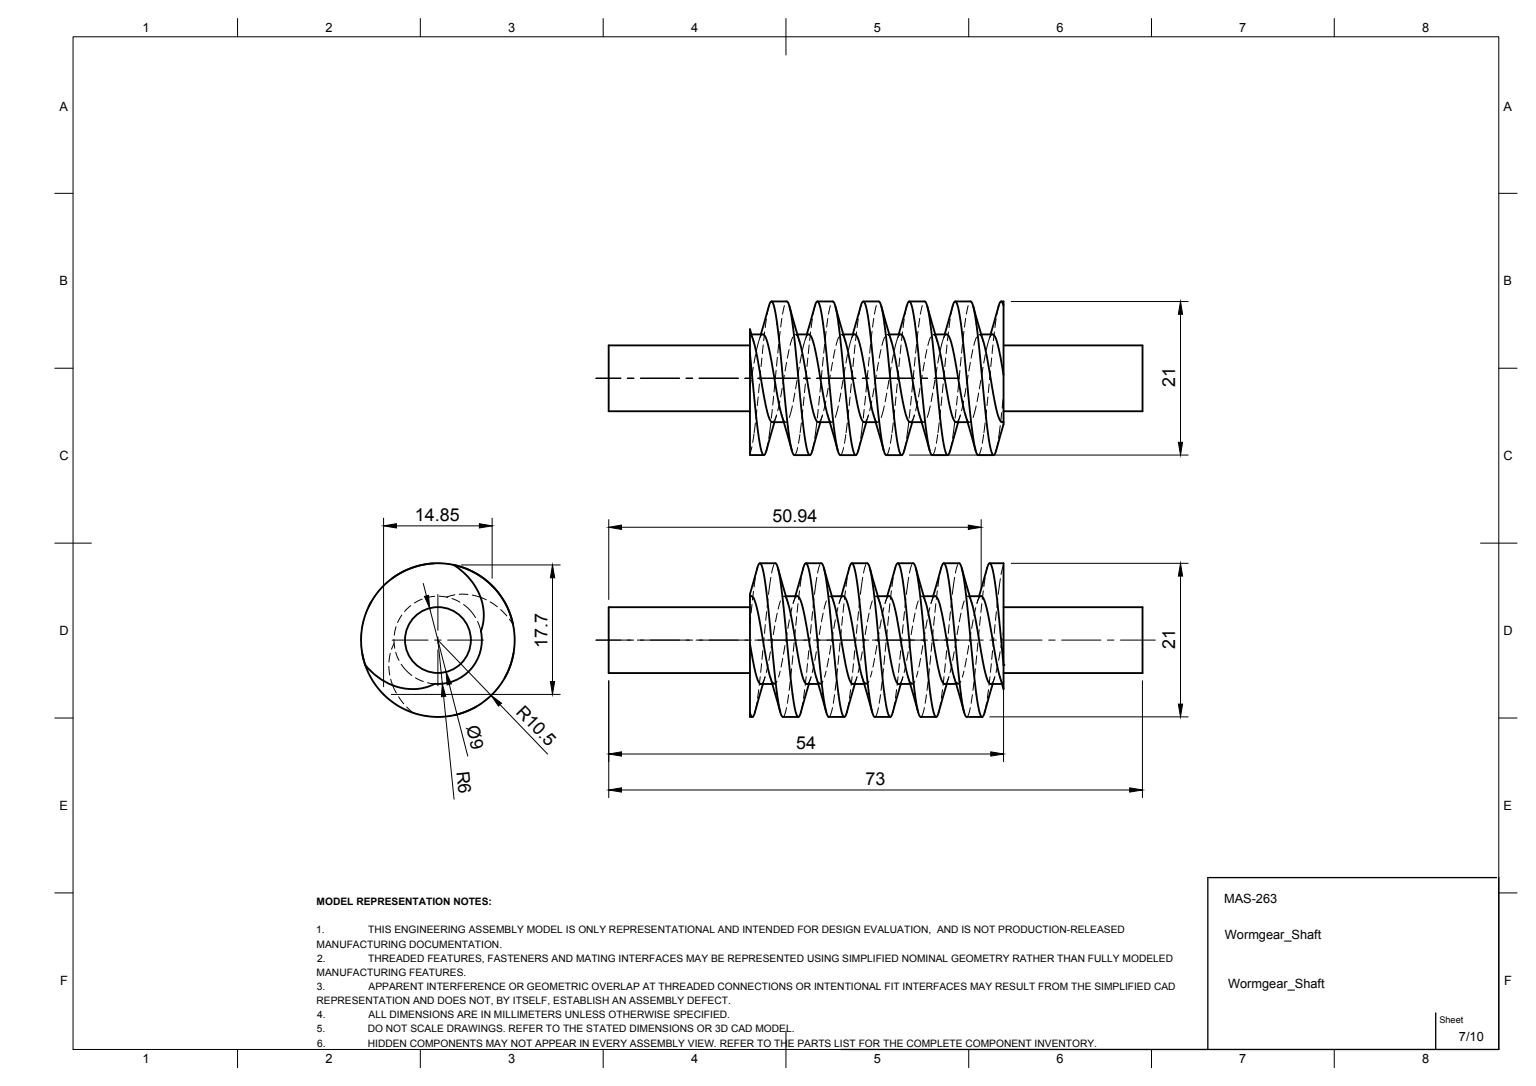
ISO-10303-21;
HEADER;
/* Generated by software containing ST-Developer
 * from STEP Tools, Inc. (www.steptools.com) 
 */

FILE_DESCRIPTION(
/* description */ (''),
/* implementation_level */ '2;1');

FILE_NAME(
/* name */ 'Wormgear_Shaft.step',
/* time_stamp */ '2026-10-12T15:47:30-07:00',
/* author */ (''),
/* organization */ (''),
/* preprocessor_version */ 'ST-DEVELOPER v20.2',
/* originating_system */ 'Autodesk Translation Framework v15.15.0.0',
/* authorisation */ '');

FILE_SCHEMA (('AUTOMOTIVE_DESIGN { 1 0 10303 214 3 1 1 }'));
ENDSEC;

DATA;
#10=MECHANICAL_DESIGN_GEOMETRIC_PRESENTATION_REPRESENTATION('',(#85),#88483);
#67=SHAPE_REPRESENTATION_RELATIONSHIP('SRR','None',#88523,#76);
#76=ADVANCED_BREP_SHAPE_REPRESENTATION('',(#120),#88477);
#85=STYLED_ITEM('',(#88574),#120);
#120=MANIFOLD_SOLID_BREP('Body1',#12995);
#238=ELLIPSE('',#13840,8.40043383461932,7.09899410493904);
#239=ELLIPSE('',#13843,8.34870203930529,7.04180185640227);
#366=FACE_BOUND('',#1889,.T.);
#367=FACE_BOUND('',#1894,.T.);
#519=PLANE('',#13839);
#520=PLANE('',#13842);
#521=PLANE('',#13849);
#522=PLANE('',#13850);
#758=B_SPLINE_SURFACE_WITH_KNOTS('',3,3,((#85029,#85030,#85031,#85032),
(#85033,#85034,#85035,#85036),(#85037,#85038,#85039,#85040),(#85041,#85042,
#85043,#85044)),.UNSPECIFIED.,.F.,.F.,.F.,(4,4),(4,4),(0.0217391304347818,
0.617536119336012),(0.774386899537597,1.),.UNSPECIFIED.);
#759=B_SPLINE_SURFACE_WITH_KNOTS('',3,3,((#85046,#85047,#85048,#85049,#85050,
#85051,#85052,#85053,#85054,#85055),(#85056,#85057,#85058,#85059,#85060,
#85061,#85062,#85063,#85064,#85065),(#85066,#85067,#85068,#85069,#85070,
#85071,#85072,#85073,#85074,#85075),(#85076,#85077,#85078,#85079,#85080,
#85081,#85082,#85083,#85084,#85085)),.UNSPECIFIED.,.F.,.F.,.F.,(4,4),(4,
1,1,1,1,1,1,4),(0.0216104565420008,1.00130145442866),(-0.000128673892780755,
0.142857142857143,0.285714285714286,0.428571428571429,0.571428571428571,
0.714285714285714,0.857142857142857,1.00130145442866),.UNSPECIFIED.);
#760=B_SPLINE_SURFACE_WITH_KNOTS('',3,3,((#85096,#85097,#85098,#85099,#85100,
#85101,#85102,#85103),(#85104,#85105,#85106,#85107,#85108,#85109,#85110,
#85111),(#85112,#85113,#85114,#85115,#85116,#85117,#85118,#85119),(#85120,
#85121,#85122,#85123,#85124,#85125,#85126,#85127)),.UNSPECIFIED.,.F.,.F.,
 .F.,(4,4),(4,1,1,1,1,4),(0.,1.00001448148635),(0.144829272278474,0.266996519095835,
0.389163765913196,0.633498259547918,0.877832753182639,1.00001448148635),
 .UNSPECIFIED.);
#761=B_SPLINE_SURFACE_WITH_KNOTS('',3,3,((#85395,#85396,#85397,#85398,#85399,
#85400,#85401,#85402,#85403),(#85404,#85405,#85406,#85407,#85408,#85409,
#85410,#85411,#85412),(#85413,#85414,#85415,#85416,#85417,#85418,#85419,
#85420,#85421),(#85422,#85423,#85424,#85425,#85426,#85427,#85428,#85429,
#85430)),.UNSPECIFIED.,.F.,.F.,.F.,(4,4),(4,1,1,1,1,1,4),(-1.22172294938054E-5,
1.),(-1.22172294938054E-5,0.12216720883009,0.24433441766018,0.488668835320359,
0.610836044150449,0.733003252980539,0.855170461810629),.UNSPECIFIED.);
#762=B_SPLINE_SURFACE_WITH_KNOTS('',3,3,((#85465,#85466,#85467,#85468),
(#85469,#85470,#85471,#85472),(#85473,#85474,#85475,#85476),(#85477,#85478,
#85479,#85480)),.UNSPECIFIED.,.F.,.F.,.F.,(4,4),(4,4),(0.512899287463832,
1.),(0.,0.18445259717643),.UNSPECIFIED.);
#763=B_SPLINE_SURFACE_WITH_KNOTS('',3,3,((#85482,#85483,#85484,#85485,#85486,
#85487,#85488,#85489,#85490,#85491),(#85492,#85493,#85494,#85495,#85496,
#85497,#85498,#85499,#85500,#85501),(#85502,#85503,#85504,#85505,#85506,
#85507,#85508,#85509,#85510,#85511),(#85512,#85513,#85514,#85515,#85516,
#85517,#85518,#85519,#85520,#85521)),.UNSPECIFIED.,.F.,.F.,.F.,(4,4),(4,
1,1,1,1,1,1,4),(0.0216104646765061,1.),(-0.000128665758275638,0.142857142857143,
0.285714285714286,0.428571428571429,0.571428571428571,0.714285714285714,
0.857142857142857,1.),.UNSPECIFIED.);
#764=B_SPLINE_SURFACE_WITH_KNOTS('',3,3,((#85543,#85544,#85545,#85546),
(#85547,#85548,#85549,#85550),(#85551,#85552,#85553,#85554),(#85555,#85556,
#85557,#85558)),.UNSPECIFIED.,.F.,.F.,.F.,(4,4),(4,4),(0.382464506767468,
0.978260874456547),(0.,0.225612834551505),.UNSPECIFIED.);
#765=B_SPLINE_SURFACE_WITH_KNOTS('',3,3,((#85560,#85561,#85562,#85563,#85564,
#85565,#85566,#85567,#85568,#85569),(#85570,#85571,#85572,#85573,#85574,
#85575,#85576,#85577,#85578,#85579),(#85580,#85581,#85582,#85583,#85584,
#85585,#85586,#85587,#85588,#85589),(#85590,#85591,#85592,#85593,#85594,
#85595,#85596,#85597,#85598,#85599)),.UNSPECIFIED.,.F.,.F.,.F.,(4,4),(4,
1,1,1,1,1,1,4),(0.,0.97838954356546),(-0.00012866910891396,0.142857142857143,
0.285714285714286,0.428571428571429,0.571428571428571,0.714285714285714,
0.857142857142857,1.00010925279131),.UNSPECIFIED.);
#766=B_SPLINE_SURFACE_WITH_KNOTS('',3,3,((#85613,#85614,#85615,#85616,#85617,
#85618,#85619,#85620,#85621,#85622),(#85623,#85624,#85625,#85626,#85627,
#85628,#85629,#85630,#85631,#85632),(#85633,#85634,#85635,#85636,#85637,
#85638,#85639,#85640,#85641,#85642),(#85643,#85644,#85645,#85646,#85647,
#85648,#85649,#85650,#85651,#85652)),.UNSPECIFIED.,.F.,.F.,.F.,(4,4),(4,
1,1,1,1,1,1,4),(0.,1.),(0.,0.142857142857143,0.285714285714286,0.428571428571429,
0.571428571428571,0.714285714285714,0.857142857142857,1.),.UNSPECIFIED.);
#767=B_SPLINE_SURFACE_WITH_KNOTS('',3,3,((#85654,#85655,#85656,#85657,#85658,
#85659,#85660,#85661,#85662,#85663),(#85664,#85665,#85666,#85667,#85668,
#85669,#85670,#85671,#85672,#85673),(#85674,#85675,#85676,#85677,#85678,
#85679,#85680,#85681,#85682,#85683),(#85684,#85685,#85686,#85687,#85688,
#85689,#85690,#85691,#85692,#85693)),.UNSPECIFIED.,.F.,.F.,.F.,(4,4),(4,
1,1,1,1,1,1,4),(0.0216103522188689,1.),(-0.00012877821591213,0.142857142857143,
0.285714285714286,0.428571428571429,0.571428571428571,0.714285714285714,
0.857142857142857,1.00010930858083),.UNSPECIFIED.);
#768=B_SPLINE_SURFACE_WITH_KNOTS('',3,3,((#85708,#85709,#85710,#85711,#85712,
#85713,#85714,#85715,#85716,#85717),(#85718,#85719,#85720,#85721,#85722,
#85723,#85724,#85725,#85726,#85727),(#85728,#85729,#85730,#85731,#85732,
#85733,#85734,#85735,#85736,#85737),(#85738,#85739,#85740,#85741,#85742,
#85743,#85744,#85745,#85746,#85747)),.UNSPECIFIED.,.F.,.F.,.F.,(4,4),(4,
1,1,1,1,1,1,4),(0.,0.97838966897386),(-0.00012879451731267,0.142857142857143,
0.285714285714286,0.428571428571429,0.571428571428571,0.714285714285714,
0.857142857142857,1.00010890844888),.UNSPECIFIED.);
#769=B_SPLINE_SURFACE_WITH_KNOTS('',3,3,((#85762,#85763,#85764,#85765,#85766,
#85767,#85768,#85769,#85770,#85771),(#85772,#85773,#85774,#85775,#85776,
#85777,#85778,#85779,#85780,#85781),(#85782,#85783,#85784,#85785,#85786,
#85787,#85788,#85789,#85790,#85791),(#85792,#85793,#85794,#85795,#85796,
#85797,#85798,#85799,#85800,#85801)),.UNSPECIFIED.,.F.,.F.,.F.,(4,4),(4,
1,1,1,1,1,1,4),(0.,1.),(0.,0.142857142857143,0.285714285714286,0.428571428571429,
0.571428571428571,0.714285714285714,0.857142857142857,1.),.UNSPECIFIED.);
#770=B_SPLINE_SURFACE_WITH_KNOTS('',3,3,((#85804,#85805,#85806,#85807,#85808,
#85809,#85810,#85811,#85812,#85813),(#85814,#85815,#85816,#85817,#85818,
#85819,#85820,#85821,#85822,#85823),(#85824,#85825,#85826,#85827,#85828,
#85829,#85830,#85831,#85832,#85833),(#85834,#85835,#85836,#85837,#85838,
#85839,#85840,#85841,#85842,#85843)),.UNSPECIFIED.,.F.,.F.,.F.,(4,4),(4,
1,1,1,1,1,1,4),(0.0216102027499123,1.),(-0.000128927684868709,0.142857142857143,
0.285714285714286,0.428571428571429,0.571428571428571,0.714285714285714,
0.857142857142857,1.00010894090728),.UNSPECIFIED.);
#771=B_SPLINE_SURFACE_WITH_KNOTS('',3,3,((#85858,#85859,#85860,#85861,#85862,
#85863,#85864,#85865,#85866,#85867),(#85868,#85869,#85870,#85871,#85872,
#85873,#85874,#85875,#85876,#85877),(#85878,#85879,#85880,#85881,#85882,
#85883,#85884,#85885,#85886,#85887),(#85888,#85889,#85890,#85891,#85892,
#85893,#85894,#85895,#85896,#85897)),.UNSPECIFIED.,.F.,.F.,.F.,(4,4),(4,
1,1,1,1,1,1,4),(-3.49469805785124E-7,0.978389836394998),(-0.000128961938451469,
0.142857142857143,0.285714285714286,0.428571428571429,0.571428571428571,
0.714285714285714,0.857142857142857,1.00010852689685),.UNSPECIFIED.);
#772=B_SPLINE_SURFACE_WITH_KNOTS('',3,3,((#85920,#85921,#85922,#85923,#85924,
#85925,#85926,#85927,#85928,#85929),(#85930,#85931,#85932,#85933,#85934,
#85935,#85936,#85937,#85938,#85939),(#85940,#85941,#85942,#85943,#85944,
#85945,#85946,#85947,#85948,#85949),(#85950,#85951,#85952,#85953,#85954,
#85955,#85956,#85957,#85958,#85959)),.UNSPECIFIED.,.F.,.F.,.F.,(4,4),(4,
1,1,1,1,1,1,4),(0.,1.00000113587033),(0.,0.142857142857143,0.285714285714286,
0.428571428571429,0.571428571428571,0.714285714285714,0.857142857142857,
1.),.UNSPECIFIED.);
#773=B_SPLINE_SURFACE_WITH_KNOTS('',3,3,((#85962,#85963,#85964,#85965,#85966,
#85967,#85968,#85969,#85970,#85971),(#85972,#85973,#85974,#85975,#85976,
#85977,#85978,#85979,#85980,#85981),(#85982,#85983,#85984,#85985,#85986,
#85987,#85988,#85989,#85990,#85991),(#85992,#85993,#85994,#85995,#85996,
#85997,#85998,#85999,#86000,#86001)),.UNSPECIFIED.,.F.,.F.,.F.,(4,4),(4,
1,1,1,1,1,1,4),(0.0216101883594699,1.),(-0.000128942075311584,0.142857142857143,
0.285714285714286,0.428571428571429,0.571428571428571,0.714285714285714,
0.857142857142857,1.00010890887743),.UNSPECIFIED.);
#774=B_SPLINE_SURFACE_WITH_KNOTS('',3,3,((#86028,#86029,#86030,#86031,#86032,
#86033,#86034,#86035,#86036,#86037),(#86038,#86039,#86040,#86041,#86042,
#86043,#86044,#86045,#86046,#86047),(#86048,#86049,#86050,#86051,#86052,
#86053,#86054,#86055,#86056,#86057),(#86058,#86059,#86060,#86061,#86062,
#86063,#86064,#86065,#86066,#86067)),.UNSPECIFIED.,.F.,.F.,.F.,(4,4),(4,
1,1,1,1,1,1,4),(0.,0.978389731943835),(-0.00012885748728817,0.142857142857143,
0.285714285714286,0.428571428571429,0.571428571428571,0.714285714285714,
0.857142857142857,1.00010875621283),.UNSPECIFIED.);
#775=B_SPLINE_SURFACE_WITH_KNOTS('',3,3,((#86082,#86083,#86084,#86085,#86086,
#86087,#86088,#86089,#86090,#86091),(#86092,#86093,#86094,#86095,#86096,
#86097,#86098,#86099,#86100,#86101),(#86102,#86103,#86104,#86105,#86106,
#86107,#86108,#86109,#86110,#86111),(#86112,#86113,#86114,#86115,#86116,
#86117,#86118,#86119,#86120,#86121)),.UNSPECIFIED.,.F.,.F.,.F.,(4,4),(4,
1,1,1,1,1,1,4),(0.,1.),(0.,0.142857142857143,0.285714285714286,0.428571428571429,
0.571428571428571,0.714285714285714,0.857142857142857,1.),.UNSPECIFIED.);
#776=B_SPLINE_SURFACE_WITH_KNOTS('',3,3,((#86124,#86125,#86126,#86127,#86128,
#86129,#86130,#86131,#86132,#86133),(#86134,#86135,#86136,#86137,#86138,
#86139,#86140,#86141,#86142,#86143),(#86144,#86145,#86146,#86147,#86148,
#86149,#86150,#86151,#86152,#86153),(#86154,#86155,#86156,#86157,#86158,
#86159,#86160,#86161,#86162,#86163)),.UNSPECIFIED.,.F.,.F.,.F.,(4,4),(4,
1,1,1,1,1,1,4),(0.0216103414761888,1.),(-0.000128788958592299,0.142857142857143,
0.285714285714286,0.428571428571429,0.571428571428571,0.714285714285714,
0.857142857142857,1.00010927970758),.UNSPECIFIED.);
#777=B_SPLINE_SURFACE_WITH_KNOTS('',3,3,((#86190,#86191,#86192,#86193,#86194,
#86195,#86196,#86197,#86198,#86199),(#86200,#86201,#86202,#86203,#86204,
#86205,#86206,#86207,#86208,#86209),(#86210,#86211,#86212,#86213,#86214,
#86215,#86216,#86217,#86218,#86219),(#86220,#86221,#86222,#86223,#86224,
#86225,#86226,#86227,#86228,#86229)),.UNSPECIFIED.,.F.,.F.,.F.,(4,4),(4,
1,1,1,1,1,1,4),(0.,0.978389590969423),(-0.000128716512876252,0.142857142857143,
0.285714285714286,0.428571428571429,0.571428571428571,0.714285714285714,
0.857142857142857,1.00010911520136),.UNSPECIFIED.);
#778=B_SPLINE_SURFACE_WITH_KNOTS('',3,3,((#86244,#86245,#86246,#86247,#86248,
#86249,#86250,#86251,#86252,#86253),(#86254,#86255,#86256,#86257,#86258,
#86259,#86260,#86261,#86262,#86263),(#86264,#86265,#86266,#86267,#86268,
#86269,#86270,#86271,#86272,#86273),(#86274,#86275,#86276,#86277,#86278,
#86279,#86280,#86281,#86282,#86283)),.UNSPECIFIED.,.F.,.F.,.F.,(4,4),(4,
1,1,1,1,1,1,4),(0.,1.),(0.,0.142857142857143,0.285714285714286,0.428571428571429,
0.571428571428571,0.714285714285714,0.857142857142857,1.),.UNSPECIFIED.);
#779=B_SPLINE_SURFACE_WITH_KNOTS('',3,3,((#86286,#86287,#86288,#86289),
(#86290,#86291,#86292,#86293),(#86294,#86295,#86296,#86297),(#86298,#86299,
#86300,#86301)),.UNSPECIFIED.,.F.,.F.,.F.,(4,4),(4,4),(0.,0.487101414751205),
(0.815547136912673,1.),.UNSPECIFIED.);
#780=B_SPLINE_SURFACE_WITH_KNOTS('',3,3,((#86303,#86304,#86305,#86306,#86307,
#86308,#86309,#86310,#86311,#86312),(#86313,#86314,#86315,#86316,#86317,
#86318,#86319,#86320,#86321,#86322),(#86323,#86324,#86325,#86326,#86327,
#86328,#86329,#86330,#86331,#86332),(#86333,#86334,#86335,#86336,#86337,
#86338,#86339,#86340,#86341,#86342)),.UNSPECIFIED.,.F.,.F.,.F.,(4,4),(4,
1,1,1,1,1,1,4),(-0.00139422224055136,0.978389538674135),(-0.00139422224055136,
0.142857142857143,0.285714285714286,0.428571428571429,0.571428571428571,
0.714285714285714,0.857142857142857,1.00012866910892),.UNSPECIFIED.);
#781=B_SPLINE_SURFACE_WITH_KNOTS('',3,3,((#86343,#86344,#86345,#86346,#86347,
#86348,#86349,#86350,#86351,#86352),(#86353,#86354,#86355,#86356,#86357,
#86358,#86359,#86360,#86361,#86362),(#86363,#86364,#86365,#86366,#86367,
#86368,#86369,#86370,#86371,#86372),(#86373,#86374,#86375,#86376,#86377,
#86378,#86379,#86380,#86381,#86382)),.UNSPECIFIED.,.F.,.F.,.F.,(4,4),(4,
1,1,1,1,1,1,4),(0.0216103522188697,1.),(-0.000128778215911952,0.142857142857143,
0.285714285714286,0.428571428571429,0.571428571428571,0.714285714285714,
0.857142857142857,1.00012877821591),.UNSPECIFIED.);
#782=B_SPLINE_SURFACE_WITH_KNOTS('',3,3,((#86393,#86394,#86395,#86396,#86397,
#86398,#86399,#86400,#86401,#86402),(#86403,#86404,#86405,#86406,#86407,
#86408,#86409,#86410,#86411,#86412),(#86413,#86414,#86415,#86416,#86417,
#86418,#86419,#86420,#86421,#86422),(#86423,#86424,#86425,#86426,#86427,
#86428,#86429,#86430,#86431,#86432)),.UNSPECIFIED.,.F.,.F.,.F.,(4,4),(4,
1,1,1,1,1,1,4),(0.,0.978389664082536),(-0.000128794517316134,0.142857142857143,
0.285714285714286,0.428571428571429,0.571428571428571,0.714285714285714,
0.857142857142857,1.00012879451732),.UNSPECIFIED.);
#783=B_SPLINE_SURFACE_WITH_KNOTS('',3,3,((#86443,#86444,#86445,#86446,#86447,
#86448,#86449,#86450,#86451,#86452),(#86453,#86454,#86455,#86456,#86457,
#86458,#86459,#86460,#86461,#86462),(#86463,#86464,#86465,#86466,#86467,
#86468,#86469,#86470,#86471,#86472),(#86473,#86474,#86475,#86476,#86477,
#86478,#86479,#86480,#86481,#86482)),.UNSPECIFIED.,.F.,.F.,.F.,(4,4),(4,
1,1,1,1,1,1,4),(0.,1.),(0.,0.142857142857143,0.285714285714286,0.428571428571429,
0.571428571428571,0.714285714285714,0.857142857142857,1.),.UNSPECIFIED.);
#784=B_SPLINE_SURFACE_WITH_KNOTS('',3,3,((#86483,#86484,#86485,#86486,#86487,
#86488,#86489,#86490,#86491,#86492),(#86493,#86494,#86495,#86496,#86497,
#86498,#86499,#86500,#86501,#86502),(#86503,#86504,#86505,#86506,#86507,
#86508,#86509,#86510,#86511,#86512),(#86513,#86514,#86515,#86516,#86517,
#86518,#86519,#86520,#86521,#86522)),.UNSPECIFIED.,.F.,.F.,.F.,(4,4),(4,
1,1,1,1,1,1,4),(0.0216102027499124,1.),(-0.000128927684869032,0.142857142857143,
0.285714285714286,0.428571428571429,0.571428571428571,0.714285714285714,
0.857142857142857,1.00012892768487),.UNSPECIFIED.);
#785=B_SPLINE_SURFACE_WITH_KNOTS('',3,3,((#86533,#86534,#86535,#86536,#86537,
#86538,#86539,#86540,#86541,#86542),(#86543,#86544,#86545,#86546,#86547,
#86548,#86549,#86550,#86551,#86552),(#86553,#86554,#86555,#86556,#86557,
#86558,#86559,#86560,#86561,#86562),(#86563,#86564,#86565,#86566,#86567,
#86568,#86569,#86570,#86571,#86572)),.UNSPECIFIED.,.F.,.F.,.F.,(4,4),(4,
1,1,1,1,1,1,4),(-3.49469809180723E-7,0.978389831503672),(-0.000128961938453871,
0.142857142857143,0.285714285714286,0.428571428571429,0.571428571428571,
0.714285714285714,0.857142857142857,1.00012896193845),.UNSPECIFIED.);
#786=B_SPLINE_SURFACE_WITH_KNOTS('',3,3,((#86591,#86592,#86593,#86594,#86595,
#86596,#86597,#86598,#86599,#86600),(#86601,#86602,#86603,#86604,#86605,
#86606,#86607,#86608,#86609,#86610),(#86611,#86612,#86613,#86614,#86615,
#86616,#86617,#86618,#86619,#86620),(#86621,#86622,#86623,#86624,#86625,
#86626,#86627,#86628,#86629,#86630)),.UNSPECIFIED.,.F.,.F.,.F.,(4,4),(4,
1,1,1,1,1,1,4),(0.,1.00000113587032),(0.,0.142857142857143,0.285714285714286,
0.428571428571429,0.571428571428571,0.714285714285714,0.857142857142857,
1.),.UNSPECIFIED.);
#787=B_SPLINE_SURFACE_WITH_KNOTS('',3,3,((#86631,#86632,#86633,#86634,#86635,
#86636,#86637,#86638,#86639,#86640),(#86641,#86642,#86643,#86644,#86645,
#86646,#86647,#86648,#86649,#86650),(#86651,#86652,#86653,#86654,#86655,
#86656,#86657,#86658,#86659,#86660),(#86661,#86662,#86663,#86664,#86665,
#86666,#86667,#86668,#86669,#86670)),.UNSPECIFIED.,.F.,.F.,.F.,(4,4),(4,
1,1,1,1,1,1,4),(0.0216101418372936,1.00000073923771),(-0.000128988597488103,
0.142857142857143,0.285714285714286,0.428571428571429,0.571428571428571,
0.714285714285714,0.857142857142857,1.00012898859749),.UNSPECIFIED.);
#788=B_SPLINE_SURFACE_WITH_KNOTS('',3,3,((#86689,#86690,#86691,#86692,#86693,
#86694,#86695,#86696,#86697,#86698),(#86699,#86700,#86701,#86702,#86703,
#86704,#86705,#86706,#86707,#86708),(#86709,#86710,#86711,#86712,#86713,
#86714,#86715,#86716,#86717,#86718),(#86719,#86720,#86721,#86722,#86723,
#86724,#86725,#86726,#86727,#86728)),.UNSPECIFIED.,.F.,.F.,.F.,(4,4),(4,
1,1,1,1,1,1,4),(0.,0.978389769713518),(-0.000128900148299539,0.142857142857143,
0.285714285714286,0.428571428571429,0.571428571428571,0.714285714285714,
0.857142857142857,1.0001289001483),.UNSPECIFIED.);
#789=B_SPLINE_SURFACE_WITH_KNOTS('',3,3,((#86739,#86740,#86741,#86742,#86743,
#86744,#86745,#86746,#86747,#86748),(#86749,#86750,#86751,#86752,#86753,
#86754,#86755,#86756,#86757,#86758),(#86759,#86760,#86761,#86762,#86763,
#86764,#86765,#86766,#86767,#86768),(#86769,#86770,#86771,#86772,#86773,
#86774,#86775,#86776,#86777,#86778)),.UNSPECIFIED.,.F.,.F.,.F.,(4,4),(4,
1,1,1,1,1,1,4),(-6.04327751791771E-7,1.),(0.,0.142857142857143,0.285714285714286,
0.428571428571429,0.571428571428571,0.714285714285714,0.857142857142857,
1.),.UNSPECIFIED.);
#790=B_SPLINE_SURFACE_WITH_KNOTS('',3,3,((#86779,#86780,#86781,#86782,#86783,
#86784,#86785,#86786,#86787,#86788),(#86789,#86790,#86791,#86792,#86793,
#86794,#86795,#86796,#86797,#86798),(#86799,#86800,#86801,#86802,#86803,
#86804,#86805,#86806,#86807,#86808),(#86809,#86810,#86811,#86812,#86813,
#86814,#86815,#86816,#86817,#86818)),.UNSPECIFIED.,.F.,.F.,.F.,(4,4),(4,
1,1,1,1,1,1,4),(0.0216103068508826,1.),(-0.000128823583898755,0.142857142857143,
0.285714285714286,0.428571428571429,0.571428571428571,0.714285714285714,
0.857142857142857,1.0001288235839),.UNSPECIFIED.);
#791=B_SPLINE_SURFACE_WITH_KNOTS('',3,3,((#86841,#86842,#86843,#86844,#86845,
#86846,#86847,#86848,#86849,#86850),(#86851,#86852,#86853,#86854,#86855,
#86856,#86857,#86858,#86859,#86860),(#86861,#86862,#86863,#86864,#86865,
#86866,#86867,#86868,#86869,#86870),(#86871,#86872,#86873,#86874,#86875,
#86876,#86877,#86878,#86879,#86880)),.UNSPECIFIED.,.F.,.F.,.F.,(4,4),(4,
1,1,1,1,1,1,4),(0.,0.978389618033113),(-0.000128748467894749,0.142857142857143,
0.285714285714286,0.428571428571429,0.571428571428571,0.714285714285714,
0.857142857142857,1.0001287484679),.UNSPECIFIED.);
#792=B_SPLINE_SURFACE_WITH_KNOTS('',3,3,((#86891,#86892,#86893,#86894,#86895,
#86896,#86897,#86898,#86899,#86900),(#86901,#86902,#86903,#86904,#86905,
#86906,#86907,#86908,#86909,#86910),(#86911,#86912,#86913,#86914,#86915,
#86916,#86917,#86918,#86919,#86920),(#86921,#86922,#86923,#86924,#86925,
#86926,#86927,#86928,#86929,#86930)),.UNSPECIFIED.,.F.,.F.,.F.,(4,4),(4,
1,1,1,1,1,1,4),(0.,1.),(0.,0.142857142857143,0.285714285714286,0.428571428571429,
0.571428571428571,0.714285714285714,0.857142857142857,1.),.UNSPECIFIED.);
#793=B_SPLINE_SURFACE_WITH_KNOTS('',3,3,((#86931,#86932,#86933,#86934,#86935,
#86936,#86937,#86938,#86939,#86940),(#86941,#86942,#86943,#86944,#86945,
#86946,#86947,#86948,#86949,#86950),(#86951,#86952,#86953,#86954,#86955,
#86956,#86957,#86958,#86959,#86960),(#86961,#86962,#86963,#86964,#86965,
#86966,#86967,#86968,#86969,#86970)),.UNSPECIFIED.,.F.,.F.,.F.,(4,4),(4,
1,1,1,1,1,1,4),(0.0216104303767174,1.),(-0.000128700058064298,0.142857142857143,
0.285714285714286,0.428571428571429,0.571428571428571,0.714285714285714,
0.857142857142857,1.00012870005806),.UNSPECIFIED.);
#794=B_SPLINE_SURFACE_WITH_KNOTS('',3,3,((#86993,#86994,#86995,#86996,#86997,
#86998,#86999,#87000,#87001,#87002),(#87003,#87004,#87005,#87006,#87007,
#87008,#87009,#87010,#87011,#87012),(#87013,#87014,#87015,#87016,#87017,
#87018,#87019,#87020,#87021,#87022),(#87023,#87024,#87025,#87026,#87027,
#87028,#87029,#87030,#87031,#87032)),.UNSPECIFIED.,.F.,.F.,.F.,(4,4),(4,
1,1,1,1,1,1,4),(0.,0.978370229937023),(0.,0.142857142857143,0.285714285714286,
0.428571428571429,0.571428571428571,0.714285714285714,0.857142857142857,
1.0001093603718),.UNSPECIFIED.);
#795=B_SPLINE_SURFACE_WITH_KNOTS('',3,3,((#87043,#87044,#87045,#87046,#87047,
#87048,#87049,#87050,#87051,#87052),(#87053,#87054,#87055,#87056,#87057,
#87058,#87059,#87060,#87061,#87062),(#87063,#87064,#87065,#87066,#87067,
#87068,#87069,#87070,#87071,#87072),(#87073,#87074,#87075,#87076,#87077,
#87078,#87079,#87080,#87081,#87082)),.UNSPECIFIED.,.F.,.F.,.F.,(4,4),(4,
1,1,1,1,1,1,4),(0.,1.),(0.,0.142857142857143,0.285714285714286,0.428571428571429,
0.571428571428571,0.714285714285714,0.857142857142857,1.),.UNSPECIFIED.);
#1196=FACE_OUTER_BOUND('',#1881,.T.);
#1197=FACE_OUTER_BOUND('',#1882,.T.);
#1198=FACE_OUTER_BOUND('',#1883,.T.);
#1199=FACE_OUTER_BOUND('',#1884,.T.);
#1200=FACE_OUTER_BOUND('',#1885,.T.);
#1201=FACE_OUTER_BOUND('',#1886,.T.);
#1202=FACE_OUTER_BOUND('',#1887,.T.);
#1203=FACE_OUTER_BOUND('',#1888,.T.);
#1204=FACE_OUTER_BOUND('',#1890,.T.);
#1205=FACE_OUTER_BOUND('',#1891,.T.);
#1206=FACE_OUTER_BOUND('',#1892,.T.);
#1207=FACE_OUTER_BOUND('',#1893,.T.);
#1208=FACE_OUTER_BOUND('',#1895,.T.);
#1209=FACE_OUTER_BOUND('',#1896,.T.);
#1210=FACE_OUTER_BOUND('',#1897,.T.);
#1211=FACE_OUTER_BOUND('',#1898,.T.);
#1212=FACE_OUTER_BOUND('',#1899,.T.);
#1213=FACE_OUTER_BOUND('',#1900,.T.);
#1214=FACE_OUTER_BOUND('',#1901,.T.);
#1215=FACE_OUTER_BOUND('',#1902,.T.);
#1216=FACE_OUTER_BOUND('',#1903,.T.);
#1217=FACE_OUTER_BOUND('',#1904,.T.);
#1218=FACE_OUTER_BOUND('',#1905,.T.);
#1219=FACE_OUTER_BOUND('',#1906,.T.);
#1220=FACE_OUTER_BOUND('',#1907,.T.);
#1221=FACE_OUTER_BOUND('',#1908,.T.);
#1222=FACE_OUTER_BOUND('',#1909,.T.);
#1223=FACE_OUTER_BOUND('',#1910,.T.);
#1224=FACE_OUTER_BOUND('',#1911,.T.);
#1225=FACE_OUTER_BOUND('',#1912,.T.);
#1226=FACE_OUTER_BOUND('',#1913,.T.);
#1227=FACE_OUTER_BOUND('',#1914,.T.);
#1228=FACE_OUTER_BOUND('',#1915,.T.);
#1229=FACE_OUTER_BOUND('',#1916,.T.);
#1230=FACE_OUTER_BOUND('',#1917,.T.);
#1231=FACE_OUTER_BOUND('',#1918,.T.);
#1232=FACE_OUTER_BOUND('',#1919,.T.);
#1233=FACE_OUTER_BOUND('',#1920,.T.);
#1234=FACE_OUTER_BOUND('',#1921,.T.);
#1235=FACE_OUTER_BOUND('',#1922,.T.);
#1236=FACE_OUTER_BOUND('',#1923,.T.);
#1237=FACE_OUTER_BOUND('',#1924,.T.);
#1238=FACE_OUTER_BOUND('',#1925,.T.);
#1239=FACE_OUTER_BOUND('',#1926,.T.);
#1240=FACE_OUTER_BOUND('',#1927,.T.);
#1241=FACE_OUTER_BOUND('',#1928,.T.);
#1242=FACE_OUTER_BOUND('',#1929,.T.);
#1243=FACE_OUTER_BOUND('',#1930,.T.);
#1244=FACE_OUTER_BOUND('',#1931,.T.);
#1245=FACE_OUTER_BOUND('',#1932,.T.);
#1246=FACE_OUTER_BOUND('',#1933,.T.);
#1881=EDGE_LOOP('',(#10958,#10959,#10960,#10961,#10962,#10963));
#1882=EDGE_LOOP('',(#10964,#10965,#10966,#10967,#10968,#10969,#10970,#10971));
#1883=EDGE_LOOP('',(#10972,#10973,#10974,#10975,#10976,#10977,#10978,#10979));
#1884=EDGE_LOOP('',(#10980,#10981,#10982,#10983,#10984,#10985,#10986,#10987));
#1885=EDGE_LOOP('',(#10988,#10989,#10990,#10991,#10992,#10993,#10994,#10995));
#1886=EDGE_LOOP('',(#10996,#10997,#10998,#10999,#11000,#11001,#11002,#11003,
#11004));
#1887=EDGE_LOOP('',(#11005,#11006,#11007));
#1888=EDGE_LOOP('',(#11008,#11009,#11010,#11011,#11012,#11013));
#1889=EDGE_LOOP('',(#11014));
#1890=EDGE_LOOP('',(#11015,#11016,#11017));
#1891=EDGE_LOOP('',(#11018,#11019,#11020,#11021,#11022,#11023));
#1892=EDGE_LOOP('',(#11024,#11025,#11026,#11027));
#1893=EDGE_LOOP('',(#11028,#11029,#11030,#11031,#11032,#11033,#11034));
#1894=EDGE_LOOP('',(#11035));
#1895=EDGE_LOOP('',(#11036,#11037,#11038,#11039));
#1896=EDGE_LOOP('',(#11040,#11041,#11042));
#1897=EDGE_LOOP('',(#11043,#11044,#11045,#11046,#11047,#11048));
#1898=EDGE_LOOP('',(#11049,#11050,#11051,#11052));
#1899=EDGE_LOOP('',(#11053,#11054,#11055,#11056));
#1900=EDGE_LOOP('',(#11057));
#1901=EDGE_LOOP('',(#11058,#11059,#11060));
#1902=EDGE_LOOP('',(#11061,#11062,#11063,#11064,#11065));
#1903=EDGE_LOOP('',(#11066,#11067,#11068,#11069));
#1904=EDGE_LOOP('',(#11070,#11071,#11072,#11073,#11074));
#1905=EDGE_LOOP('',(#11075,#11076,#11077,#11078,#11079));
#1906=EDGE_LOOP('',(#11080,#11081,#11082,#11083));
#1907=EDGE_LOOP('',(#11084,#11085,#11086,#11087,#11088));
#1908=EDGE_LOOP('',(#11089,#11090,#11091,#11092,#11093));
#1909=EDGE_LOOP('',(#11094,#11095,#11096,#11097));
#1910=EDGE_LOOP('',(#11098,#11099,#11100,#11101,#11102));
#1911=EDGE_LOOP('',(#11103,#11104,#11105,#11106,#11107));
#1912=EDGE_LOOP('',(#11108,#11109,#11110,#11111));
#1913=EDGE_LOOP('',(#11112,#11113,#11114,#11115,#11116));
#1914=EDGE_LOOP('',(#11117,#11118,#11119,#11120,#11121));
#1915=EDGE_LOOP('',(#11122,#11123,#11124,#11125));
#1916=EDGE_LOOP('',(#11126,#11127,#11128));
#1917=EDGE_LOOP('',(#11129,#11130,#11131,#11132,#11133));
#1918=EDGE_LOOP('',(#11134,#11135,#11136,#11137));
#1919=EDGE_LOOP('',(#11138,#11139,#11140,#11141));
#1920=EDGE_LOOP('',(#11142,#11143,#11144,#11145));
#1921=EDGE_LOOP('',(#11146,#11147,#11148,#11149));
#1922=EDGE_LOOP('',(#11150,#11151,#11152,#11153));
#1923=EDGE_LOOP('',(#11154,#11155,#11156,#11157));
#1924=EDGE_LOOP('',(#11158,#11159,#11160,#11161));
#1925=EDGE_LOOP('',(#11162,#11163,#11164,#11165));
#1926=EDGE_LOOP('',(#11166,#11167,#11168,#11169));
#1927=EDGE_LOOP('',(#11170,#11171,#11172,#11173));
#1928=EDGE_LOOP('',(#11174,#11175,#11176,#11177));
#1929=EDGE_LOOP('',(#11178,#11179,#11180,#11181));
#1930=EDGE_LOOP('',(#11182,#11183,#11184,#11185));
#1931=EDGE_LOOP('',(#11186,#11187,#11188,#11189,#11190));
#1932=EDGE_LOOP('',(#11191,#11192,#11193,#11194));
#1933=EDGE_LOOP('',(#11195));
#2618=CIRCLE('',#13830,6.);
#2619=CIRCLE('',#13836,6.);
#2620=CIRCLE('',#13838,6.);
#2621=CIRCLE('',#13841,4.5);
#2622=CIRCLE('',#13844,4.5);
#2623=CIRCLE('',#13846,4.5);
#2624=CIRCLE('',#13848,4.5);
#3560=B_SPLINE_CURVE_WITH_KNOTS('',3,(#81965,#81966,#81967,#81968,#81969,
#81970,#81971,#81972,#81973,#81974,#81975,#81976,#81977,#81978,#81979,#81980,
#81981,#81982,#81983,#81984,#81985,#81986,#81987,#81988,#81989,#81990,#81991,
#81992,#81993,#81994,#81995,#81996,#81997,#81998,#81999,#82000,#82001,#82002,
#82003,#82004,#82005,#82006,#82007,#82008,#82009,#82010,#82011,#82012,#82013,
#82014,#82015,#82016,#82017,#82018,#82019,#82020,#82021,#82022,#82023,#82024,
#82025,#82026,#82027,#82028),.UNSPECIFIED.,.F.,.F.,(4,3,3,3,3,3,3,3,3,3,
3,3,3,3,3,3,3,3,3,3,3,4),(0.479292617177209,0.505000840917307,0.530713137629105,
0.547756394224347,0.57336762750038,0.598976297476449,0.62458735299975,0.650198139465077,
0.675813884972614,0.684683947910694,0.710199819641625,0.735710769342924,
0.761221509088754,0.786730721796191,0.812243799751802,0.821611501597041,
0.847360903592922,0.873107128637788,0.898853495292093,0.924597895094032,
0.95034373058283,0.958539055283388),.UNSPECIFIED.);
#3561=B_SPLINE_CURVE_WITH_KNOTS('',3,(#82030,#82031,#82032,#82033,#82034,
#82035,#82036,#82037,#82038,#82039,#82040,#82041,#82042,#82043,#82044,#82045,
#82046,#82047,#82048,#82049,#82050,#82051,#82052,#82053,#82054,#82055,#82056,
#82057,#82058,#82059,#82060,#82061,#82062,#82063,#82064,#82065,#82066,#82067,
#82068,#82069,#82070,#82071,#82072,#82073,#82074,#82075,#82076,#82077,#82078,
#82079,#82080,#82081,#82082,#82083,#82084,#82085,#82086,#82087,#82088,#82089,
#82090,#82091,#82092,#82093,#82094,#82095,#82096,#82097,#82098,#82099,#82100,
#82101,#82102,#82103,#82104,#82105,#82106,#82107,#82108,#82109,#82110,#82111,
#82112,#82113,#82114,#82115,#82116,#82117,#82118,#82119,#82120,#82121,#82122,
#82123,#82124,#82125,#82126,#82127,#82128,#82129,#82130,#82131,#82132),
 .UNSPECIFIED.,.F.,.F.,(4,3,3,3,3,3,3,3,3,3,3,3,3,3,3,3,3,3,3,3,3,3,3,3,
3,3,3,3,3,3,3,3,3,3,4),(0.,0.0255611682442398,0.0511196475252543,0.0766807791052086,
0.102241920428134,0.127808798952552,0.136937787707076,0.162568577806161,
0.188195056364783,0.213821211828165,0.23944549133029,0.265072298366607,
0.273875575414151,0.299433431887937,0.32498835629455,0.350545625560006,
0.376102741264404,0.401665398667488,0.410813363121227,0.436405033823088,
0.461991883117399,0.487578024623893,0.513162172427522,0.538748975424076,
0.547751150828302,0.573364266367873,0.59897482287007,0.624587772130241,
0.650200456525016,0.675818106794432,0.684688938535378,0.710236075973954,
0.735777726404149,0.761318556176312,0.780281541707351),.UNSPECIFIED.);
#3562=B_SPLINE_CURVE_WITH_KNOTS('',3,(#82136,#82137,#82138,#82139,#82140,
#82141),.UNSPECIFIED.,.F.,.F.,(4,2,4),(0.,0.216145308133088,0.432258182334419),
 .UNSPECIFIED.);
#3563=B_SPLINE_CURVE_WITH_KNOTS('',3,(#82142,#82143,#82144,#82145,#82146,
#82147,#82148,#82149,#82150,#82151,#82152,#82153,#82154,#82155,#82156,#82157,
#82158,#82159,#82160,#82161,#82162,#82163,#82164,#82165,#82166,#82167,#82168,
#82169,#82170,#82171,#82172,#82173,#82174,#82175,#82176,#82177,#82178,#82179,
#82180,#82181,#82182,#82183,#82184,#82185,#82186,#82187,#82188,#82189,#82190,
#82191,#82192,#82193,#82194,#82195,#82196,#82197,#82198,#82199,#82200,#82201,
#82202,#82203,#82204,#82205),.UNSPECIFIED.,.F.,.F.,(4,3,3,3,3,3,3,3,3,3,
3,3,3,3,3,3,3,3,3,3,3,4),(0.,0.0257479719507909,0.0514943137831926,0.0772430807474856,
0.102991209339309,0.12874269019043,0.136940747823198,0.162456524286232,
0.18796862101097,0.213482344429356,0.23899560263191,0.264514271518437,0.273881495646396,
0.299499689510765,0.325113349245822,0.350726484436241,0.376337663430009,
0.401951356406392,0.410822243469594,0.436536016946579,0.462248012834959,
0.47929261717721),.UNSPECIFIED.);
#3564=B_SPLINE_CURVE_WITH_KNOTS('',3,(#82211,#82212,#82213,#82214,#82215,
#82216,#82217,#82218,#82219,#82220,#82221,#82222,#82223,#82224,#82225,#82226,
#82227,#82228,#82229,#82230,#82231,#82232,#82233,#82234,#82235,#82236,#82237,
#82238,#82239,#82240,#82241,#82242,#82243,#82244,#82245,#82246,#82247,#82248,
#82249,#82250,#82251,#82252,#82253,#82254,#82255,#82256,#82257,#82258,#82259,
#82260,#82261,#82262,#82263,#82264,#82265,#82266,#82267,#82268,#82269,#82270,
#82271,#82272,#82273,#82274),.UNSPECIFIED.,.F.,.F.,(4,3,3,3,3,3,3,3,3,3,
3,3,3,3,3,3,3,3,3,3,3,4),(0.479292617177209,0.505001327382096,0.530714120836313,
0.547756394224347,0.573367708107215,0.5989764517365,0.624587569678354,0.650198411765993,
0.675814202278988,0.684683947910694,0.710199270596006,0.735709680648712,
0.761219898903124,0.786728601757571,0.812241190362207,0.82161150159704,
0.847361553520347,0.873108430011801,0.89885544393772,0.92460048661686,0.950346953615207,
0.958539055283387),.UNSPECIFIED.);
#3565=B_SPLINE_CURVE_WITH_KNOTS('',3,(#82276,#82277,#82278,#82279,#82280,
#82281,#82282,#82283,#82284,#82285,#82286,#82287,#82288,#82289,#82290,#82291,
#82292,#82293,#82294,#82295,#82296,#82297,#82298,#82299,#82300,#82301,#82302,
#82303,#82304,#82305,#82306,#82307,#82308,#82309,#82310,#82311,#82312,#82313,
#82314,#82315,#82316,#82317,#82318,#82319,#82320,#82321,#82322,#82323,#82324,
#82325,#82326,#82327,#82328,#82329,#82330,#82331,#82332,#82333,#82334,#82335,
#82336,#82337,#82338,#82339,#82340,#82341,#82342,#82343,#82344,#82345,#82346,
#82347,#82348,#82349,#82350,#82351,#82352,#82353,#82354,#82355,#82356,#82357,
#82358,#82359,#82360,#82361,#82362,#82363,#82364,#82365,#82366,#82367,#82368,
#82369,#82370,#82371,#82372,#82373,#82374,#82375,#82376,#82377,#82378,#82379,
#82380,#82381,#82382,#82383,#82384,#82385,#82386,#82387,#82388,#82389,#82390,
#82391,#82392,#82393,#82394,#82395,#82396,#82397,#82398,#82399,#82400,#82401,
#82402),.UNSPECIFIED.,.F.,.F.,(4,3,3,3,3,3,3,3,3,3,3,3,3,3,3,3,3,3,3,3,
3,3,3,3,3,3,3,3,3,3,3,3,3,3,3,3,3,3,3,3,3,3,4),(0.,0.0255611464246521,0.05111961735306,
0.0766807545207074,0.102241907980011,0.127808803185896,0.13693415075477,
0.162564198332204,0.188189930450198,0.21381533459465,0.239438860313218,
0.265064910696906,0.273868301509539,0.299425506394592,0.324979768153375,
0.35053635819426,0.376092785100791,0.401654739600194,0.410802452264309,
0.436393221748823,0.46197917265453,0.487564421430711,0.513147680282411,
0.538733601021664,0.547736603019078,0.573349086037912,0.598959003993817,
0.62457130498956,0.650183335334688,0.675800322512345,0.684670753773848,
0.710187725086894,0.73569977633771,0.761211621888362,0.786721943062233,
0.812236134492197,0.821604904528618,0.847355702730773,0.873103324254661,
0.89885108648345,0.924596880763502,0.9503441081478,0.958539055283387),
 .UNSPECIFIED.);
#3566=B_SPLINE_CURVE_WITH_KNOTS('',3,(#82403,#82404,#82405,#82406,#82407,
#82408,#82409,#82410,#82411,#82412,#82413,#82414,#82415,#82416,#82417,#82418,
#82419,#82420,#82421,#82422,#82423,#82424,#82425,#82426,#82427,#82428,#82429,
#82430,#82431,#82432,#82433,#82434,#82435,#82436,#82437,#82438,#82439,#82440,
#82441,#82442,#82443,#82444,#82445,#82446,#82447,#82448,#82449,#82450,#82451,
#82452,#82453,#82454,#82455,#82456,#82457,#82458,#82459,#82460,#82461,#82462,
#82463,#82464,#82465,#82466),.UNSPECIFIED.,.F.,.F.,(4,3,3,3,3,3,3,3,3,3,
3,3,3,3,3,3,3,3,3,3,3,4),(0.,0.0255621962959842,0.0511217133779092,0.0766838931244148,
0.102246087451785,0.12781402264808,0.136940747823198,0.162572051839977,
0.188199041285704,0.213825704029898,0.239450488906111,0.265077799247033,
0.273881495646396,0.299439922937785,0.324995409932617,0.35055322974378,
0.376110888981581,0.401674079835378,0.410822243469594,0.436808285767853,
0.462788710530963,0.479292617177209),.UNSPECIFIED.);
#3567=B_SPLINE_CURVE_WITH_KNOTS('',3,(#82468,#82469,#82470,#82471,#82472,
#82473,#82474,#82475,#82476,#82477,#82478,#82479,#82480,#82481,#82482,#82483,
#82484,#82485,#82486,#82487,#82488,#82489,#82490,#82491,#82492,#82493,#82494,
#82495,#82496,#82497,#82498,#82499,#82500,#82501,#82502,#82503,#82504,#82505,
#82506,#82507,#82508,#82509,#82510,#82511,#82512,#82513,#82514,#82515,#82516,
#82517,#82518,#82519,#82520,#82521,#82522,#82523,#82524,#82525,#82526,#82527,
#82528,#82529,#82530,#82531),.UNSPECIFIED.,.F.,.F.,(4,3,3,3,3,3,3,3,3,3,
3,3,3,3,3,3,3,3,3,3,3,4),(0.47929261717721,0.50526908884444,0.531253388712084,
0.547756394224346,0.573317123506841,0.598872836724378,0.624427812859824,
0.649980850854883,0.675536835901665,0.684683947910693,0.710308819151011,
0.735931126543647,0.761555691319374,0.787179876706826,0.812808757477038,
0.82161150159704,0.847176507707005,0.872736342186476,0.898295157372897,
0.923851855982624,0.949411200600672,0.958539055283387),.UNSPECIFIED.);
#3568=B_SPLINE_CURVE_WITH_KNOTS('',3,(#82533,#82534,#82535,#82536,#82537,
#82538,#82539,#82540,#82541,#82542,#82543,#82544,#82545,#82546,#82547,#82548,
#82549,#82550,#82551,#82552,#82553,#82554,#82555,#82556,#82557,#82558,#82559,
#82560,#82561,#82562,#82563,#82564,#82565,#82566,#82567,#82568,#82569,#82570,
#82571,#82572,#82573,#82574,#82575,#82576,#82577,#82578,#82579,#82580,#82581,
#82582,#82583,#82584,#82585,#82586,#82587,#82588,#82589,#82590,#82591,#82592,
#82593,#82594,#82595,#82596,#82597,#82598,#82599,#82600,#82601,#82602,#82603,
#82604,#82605,#82606,#82607,#82608,#82609,#82610,#82611,#82612,#82613,#82614,
#82615,#82616,#82617,#82618,#82619,#82620,#82621,#82622,#82623,#82624,#82625,
#82626,#82627,#82628,#82629,#82630,#82631,#82632,#82633,#82634,#82635,#82636,
#82637,#82638,#82639,#82640,#82641,#82642,#82643,#82644,#82645,#82646,#82647,
#82648,#82649,#82650,#82651,#82652,#82653,#82654,#82655,#82656,#82657,#82658,
#82659),.UNSPECIFIED.,.F.,.F.,(4,3,3,3,3,3,3,3,3,3,3,3,3,3,3,3,3,3,3,3,
3,3,3,3,3,3,3,3,3,3,3,3,3,3,3,3,3,3,3,3,3,3,4),(0.,0.0257468698833424,0.0514921116641796,
0.0772397799040712,0.102986810214673,0.128737192099745,0.136934150754769,
0.162448594603267,0.187959355420383,0.213471738614108,0.238983654397716,
0.264500978128848,0.273868301509539,0.299485263220318,0.32509769272638,
0.350709600094688,0.376319552699293,0.401932020998882,0.410802452264308,
0.436388483272024,0.461971827501006,0.48755761887005,0.513143244771744,
0.538734180026944,0.547736603019078,0.573298556820878,0.598855497016331,
0.624411704087103,0.649965975236065,0.675523196940356,0.684670753773847,
0.710296844933874,0.735920372698376,0.761546159030797,0.787171566648004,
0.812801671053547,0.821604904528617,0.847171306528443,0.872732535722516,
0.898292742853538,0.923850831355127,0.949411562047455,0.958539055283386),
 .UNSPECIFIED.);
#3569=B_SPLINE_CURVE_WITH_KNOTS('',3,(#82660,#82661,#82662,#82663,#82664,
#82665,#82666,#82667,#82668,#82669,#82670,#82671,#82672,#82673,#82674,#82675,
#82676,#82677,#82678,#82679,#82680,#82681,#82682,#82683,#82684,#82685,#82686,
#82687,#82688,#82689,#82690,#82691,#82692,#82693,#82694,#82695,#82696,#82697,
#82698,#82699,#82700,#82701,#82702,#82703,#82704,#82705,#82706,#82707,#82708,
#82709,#82710,#82711,#82712,#82713,#82714,#82715,#82716,#82717,#82718,#82719,
#82720,#82721,#82722,#82723),.UNSPECIFIED.,.F.,.F.,(4,3,3,3,3,3,3,3,3,3,
3,3,3,3,3,3,3,3,3,3,3,4),(0.,0.0257485479088003,0.0514954739738495,0.0772448314910723,
0.102993552532202,0.128745623912882,0.136940747823198,0.16245608850035,
0.187967734750382,0.213480989744456,0.23899377013341,0.264511950710105,
0.273881495646396,0.299499709480288,0.3251133965368,0.35072656922542,0.376337791412174,
0.401951535304368,0.410822243469594,0.436536442242556,0.462248854910223,
0.47929261717721),.UNSPECIFIED.);
#3570=B_SPLINE_CURVE_WITH_KNOTS('',3,(#82729,#82730,#82731,#82732,#82733,
#82734,#82735,#82736,#82737,#82738,#82739,#82740,#82741,#82742,#82743,#82744,
#82745,#82746,#82747,#82748,#82749,#82750,#82751,#82752,#82753,#82754,#82755,
#82756,#82757,#82758,#82759,#82760,#82761,#82762,#82763,#82764,#82765,#82766,
#82767,#82768,#82769,#82770,#82771,#82772,#82773,#82774,#82775,#82776,#82777,
#82778,#82779,#82780,#82781,#82782,#82783,#82784,#82785,#82786,#82787,#82788,
#82789,#82790,#82791,#82792),.UNSPECIFIED.,.F.,.F.,(4,3,3,3,3,3,3,3,3,3,
3,3,3,3,3,3,3,3,3,3,3,4),(0.479292617177209,0.505001679057846,0.530714831987189,
0.547756394224347,0.573367782262073,0.598976595249061,0.624587774647072,
0.650198673372923,0.675814512887766,0.684683947910694,0.710198896452721,
0.735708938883533,0.761218802071892,0.78672715789912,0.812239413611988,
0.82161150159704,0.84736198318122,0.873109289958388,0.898856730869144,0.924602197319219,
0.950349080143881,0.958539055283387),.UNSPECIFIED.);
#3571=B_SPLINE_CURVE_WITH_KNOTS('',3,(#82794,#82795,#82796,#82797,#82798,
#82799,#82800,#82801,#82802,#82803,#82804,#82805,#82806,#82807,#82808,#82809,
#82810,#82811,#82812,#82813,#82814,#82815,#82816,#82817,#82818,#82819,#82820,
#82821,#82822,#82823,#82824,#82825,#82826,#82827,#82828,#82829,#82830,#82831,
#82832,#82833,#82834,#82835,#82836,#82837,#82838,#82839,#82840,#82841,#82842,
#82843,#82844,#82845,#82846,#82847,#82848,#82849,#82850,#82851,#82852,#82853,
#82854,#82855,#82856,#82857,#82858,#82859,#82860,#82861,#82862,#82863,#82864,
#82865,#82866,#82867,#82868,#82869,#82870,#82871,#82872,#82873,#82874,#82875,
#82876,#82877,#82878,#82879,#82880,#82881,#82882,#82883,#82884,#82885,#82886,
#82887,#82888,#82889,#82890,#82891,#82892,#82893,#82894,#82895,#82896,#82897,
#82898,#82899,#82900,#82901,#82902,#82903,#82904,#82905,#82906,#82907,#82908,
#82909,#82910,#82911,#82912,#82913,#82914,#82915,#82916,#82917,#82918,#82919,
#82920),.UNSPECIFIED.,.F.,.F.,(4,3,3,3,3,3,3,3,3,3,3,3,3,3,3,3,3,3,3,3,
3,3,3,3,3,3,3,3,3,3,3,3,3,3,3,3,3,3,3,3,3,3,4),(0.,0.0255619939227406,0.0511213281374935,
0.0766833444398237,0.102245384185567,0.127813169841507,0.13693415075477,
0.162564057304859,0.188189643439327,0.213814896138194,0.239438267791297,
0.265064161788029,0.273868301509539,0.299425560181825,0.324979862788474,
0.350536474274596,0.376092911315033,0.401654859286199,0.410802452264309,
0.436392939165486,0.461978611441267,0.487563589554087,0.513146582949068,
0.538732247536879,0.547736603019078,0.573349179912026,0.598959184439744,
0.624571560133446,0.650183657974615,0.67580070134257,0.684670753773848,
0.71018715005693,0.735698636171859,0.761209935684971,0.786719723058999,
0.812233402235842,0.821604904528618,0.847356377225811,0.873104674637665,
0.898853108159833,0.924599569023129,0.950347450985566,0.958539055283387),
 .UNSPECIFIED.);
#3572=B_SPLINE_CURVE_WITH_KNOTS('',3,(#82921,#82922,#82923,#82924,#82925,
#82926,#82927,#82928,#82929,#82930,#82931,#82932,#82933,#82934,#82935,#82936,
#82937,#82938,#82939,#82940,#82941,#82942,#82943,#82944,#82945,#82946,#82947,
#82948,#82949,#82950,#82951,#82952,#82953,#82954,#82955,#82956,#82957,#82958,
#82959,#82960,#82961,#82962,#82963,#82964,#82965,#82966,#82967,#82968,#82969,
#82970,#82971,#82972,#82973,#82974,#82975,#82976,#82977,#82978,#82979,#82980,
#82981,#82982,#82983,#82984),.UNSPECIFIED.,.F.,.F.,(4,3,3,3,3,3,3,3,3,3,
3,3,3,3,3,3,3,3,3,3,3,4),(0.,0.0255629888202805,0.0511233135427478,0.0766863162753848,
0.102249340582942,0.127818110100948,0.136940747823198,0.162571934653423,
0.188198802218777,0.213825337772865,0.239449992859417,0.265077170929289,
0.273881495646396,0.299439968602179,0.3249954888192,0.350553323253718,0.376110986287893,
0.401674165036479,0.410822243469594,0.436807223890087,0.4627865956417,0.479292617174637),
 .UNSPECIFIED.);
#3573=B_SPLINE_CURVE_WITH_KNOTS('',3,(#82986,#82987,#82988,#82989,#82990,
#82991,#82992,#82993,#82994,#82995,#82996,#82997,#82998,#82999,#83000,#83001,
#83002,#83003,#83004,#83005,#83006,#83007,#83008,#83009,#83010,#83011,#83012,
#83013,#83014,#83015,#83016,#83017,#83018,#83019,#83020,#83021,#83022,#83023,
#83024,#83025,#83026,#83027,#83028,#83029,#83030,#83031,#83032,#83033,#83034,
#83035,#83036,#83037,#83038,#83039,#83040,#83041,#83042,#83043,#83044,#83045,
#83046,#83047,#83048,#83049),.UNSPECIFIED.,.F.,.F.,(4,3,3,3,3,3,3,3,3,3,
3,3,3,3,3,3,3,3,3,3,3,4),(0.47929261717721,0.505268190015835,0.53125158411797,
0.547756394224346,0.573317100440759,0.598872801966681,0.624427783168165,
0.649980835915105,0.675536849746693,0.684683947910693,0.710308737821271,
0.735930966056476,0.761555456007261,0.78717956941456,0.812808383216706,
0.82161150159704,0.847177217066114,0.872737757364608,0.898297267271713,
0.923854652547247,0.949414667311442,0.958539055283387),.UNSPECIFIED.);
#3574=B_SPLINE_CURVE_WITH_KNOTS('',3,(#83051,#83052,#83053,#83054,#83055,
#83056,#83057,#83058,#83059,#83060,#83061,#83062,#83063,#83064,#83065,#83066,
#83067,#83068,#83069,#83070,#83071,#83072,#83073,#83074,#83075,#83076,#83077,
#83078,#83079,#83080,#83081,#83082,#83083,#83084,#83085,#83086,#83087,#83088,
#83089,#83090,#83091,#83092,#83093,#83094,#83095,#83096,#83097,#83098,#83099,
#83100,#83101,#83102,#83103,#83104,#83105,#83106,#83107,#83108,#83109,#83110,
#83111,#83112,#83113,#83114,#83115,#83116,#83117,#83118,#83119,#83120,#83121,
#83122,#83123,#83124,#83125,#83126,#83127,#83128,#83129,#83130,#83131,#83132,
#83133,#83134,#83135,#83136,#83137,#83138,#83139,#83140,#83141,#83142,#83143,
#83144,#83145,#83146,#83147,#83148,#83149,#83150,#83151,#83152,#83153,#83154,
#83155,#83156,#83157,#83158,#83159,#83160,#83161,#83162,#83163,#83164,#83165,
#83166,#83167,#83168,#83169,#83170,#83171,#83172,#83173,#83174,#83175,#83176,
#83177),.UNSPECIFIED.,.F.,.F.,(4,3,3,3,3,3,3,3,3,3,3,3,3,3,3,3,3,3,3,3,
3,3,3,3,3,3,3,3,3,3,3,3,3,3,3,3,3,3,3,3,3,3,4),(0.,0.0257474663313306,0.051493313275948,
0.0772415934420302,0.102989237768966,0.128740231865067,0.136934150754769,
0.162448139512518,0.187958429852175,0.213470323759636,0.238981740416334,
0.264498554012216,0.273868301509539,0.299485292022666,0.325097758125654,
0.350709712822948,0.376319718744946,0.401932248431029,0.410802452264308,
0.436388264300392,0.461971383426754,0.487556942438714,0.513142332269183,
0.538733027566822,0.547736603019078,0.573298537314448,0.598855469883609,
0.624411686786277,0.64996597784542,0.675523234025067,0.684670753773847,
0.710296746065935,0.735920177050789,0.76154587098572,0.787171189128425,
0.812801209325657,0.821604904528617,0.847172060057425,0.872734039337613,
0.898294985218545,0.923853804170973,0.949415248127543,0.958539055283386),
 .UNSPECIFIED.);
#3575=B_SPLINE_CURVE_WITH_KNOTS('',3,(#83178,#83179,#83180,#83181,#83182,
#83183,#83184,#83185,#83186,#83187,#83188,#83189,#83190,#83191,#83192,#83193,
#83194,#83195,#83196,#83197,#83198,#83199,#83200,#83201,#83202,#83203,#83204,
#83205,#83206,#83207,#83208,#83209,#83210,#83211,#83212,#83213,#83214,#83215,
#83216,#83217,#83218,#83219,#83220,#83221,#83222,#83223,#83224,#83225,#83226,
#83227,#83228,#83229,#83230,#83231,#83232,#83233,#83234,#83235,#83236,#83237,
#83238,#83239,#83240,#83241),.UNSPECIFIED.,.F.,.F.,(4,3,3,3,3,3,3,3,3,3,
3,3,3,3,3,3,3,3,3,3,3,4),(0.,0.0257492105713833,0.0514968095059438,0.0772468481796215,
0.102996253150109,0.12874900710514,0.136940747823198,0.162455568546276,
0.187966677069076,0.213479372579753,0.238991582093521,0.264509179016115,
0.273881495646396,0.299499769501555,0.325113525936777,0.350726780699462,
0.376338091987283,0.401951934277687,0.410822243469594,0.436536985254516,
0.462249929267478,0.47929261717721),.UNSPECIFIED.);
#3576=B_SPLINE_CURVE_WITH_KNOTS('',3,(#83247,#83248,#83249,#83250,#83251,
#83252,#83253,#83254,#83255,#83256,#83257,#83258,#83259,#83260,#83261,#83262,
#83263,#83264,#83265,#83266,#83267,#83268,#83269,#83270,#83271,#83272,#83273,
#83274,#83275,#83276,#83277,#83278,#83279,#83280,#83281,#83282,#83283,#83284,
#83285,#83286,#83287,#83288,#83289,#83290,#83291,#83292,#83293,#83294,#83295,
#83296,#83297,#83298,#83299,#83300,#83301,#83302,#83303,#83304,#83305,#83306,
#83307,#83308,#83309,#83310),.UNSPECIFIED.,.F.,.F.,(4,3,3,3,3,3,3,3,3,3,
3,3,3,3,3,3,3,3,3,3,3,4),(0.479292617177209,0.505001112402896,0.530713686248326,
0.547756394224347,0.573367668816933,0.598976376178496,0.624587462770878,
0.650198276493159,0.675814043328,0.684683947910694,0.710199508692036,0.735710152743036,
0.761220597085833,0.786729520960406,0.812242321661702,0.82161150159704,
0.847361274447889,0.873107871298353,0.898854607494945,0.924599374399674,
0.950345570599475,0.958539055283387),.UNSPECIFIED.);
#3577=B_SPLINE_CURVE_WITH_KNOTS('',3,(#83312,#83313,#83314,#83315,#83316,
#83317,#83318,#83319,#83320,#83321,#83322,#83323,#83324,#83325,#83326,#83327,
#83328,#83329,#83330,#83331,#83332,#83333,#83334,#83335,#83336,#83337,#83338,
#83339,#83340,#83341,#83342,#83343,#83344,#83345,#83346,#83347,#83348,#83349,
#83350,#83351,#83352,#83353,#83354,#83355,#83356,#83357,#83358,#83359,#83360,
#83361,#83362,#83363,#83364,#83365,#83366,#83367,#83368,#83369,#83370,#83371,
#83372,#83373,#83374,#83375,#83376,#83377,#83378,#83379,#83380,#83381,#83382,
#83383,#83384,#83385,#83386,#83387,#83388,#83389,#83390,#83391,#83392,#83393,
#83394,#83395,#83396,#83397,#83398,#83399,#83400,#83401,#83402,#83403,#83404,
#83405,#83406,#83407,#83408,#83409,#83410,#83411,#83412,#83413,#83414,#83415,
#83416,#83417,#83418,#83419,#83420,#83421,#83422,#83423,#83424,#83425,#83426,
#83427,#83428,#83429,#83430,#83431,#83432,#83433,#83434,#83435,#83436,#83437,
#83438),.UNSPECIFIED.,.F.,.F.,(4,3,3,3,3,3,3,3,3,3,3,3,3,3,3,3,3,3,3,3,
3,3,3,3,3,3,3,3,3,3,3,3,3,3,3,3,3,3,3,3,3,3,4),(0.,0.02556233511759,0.0511220164970866,
0.0766843857678656,0.102246781025239,0.127814923376965,0.13693415075477,
0.162563984146602,0.188189495193546,0.213814670831708,0.239437964536715,
0.265063779997811,0.273868301509539,0.299425587203,0.324979912003907,0.350536538379918,
0.376092986033964,0.401654938265957,0.410802452264309,0.436392827093722,
0.461978389004138,0.487563260120719,0.513146148707476,0.538731712359866,
0.547736603019078,0.573349224994543,0.598959271795233,0.624571685120951,
0.650183817761065,0.675800891428116,0.684670753773848,0.710186931607258,
0.735698203093025,0.761209295327788,0.786718880128828,0.812232365003339,
0.821604904528618,0.847356626751991,0.873105174015333,0.898853855418756,
0.924600562266398,0.950348685556951,0.958539055283387),.UNSPECIFIED.);
#3578=B_SPLINE_CURVE_WITH_KNOTS('',3,(#83439,#83440,#83441,#83442,#83443,
#83444,#83445,#83446,#83447,#83448,#83449,#83450,#83451,#83452,#83453,#83454,
#83455,#83456,#83457,#83458,#83459,#83460,#83461,#83462,#83463,#83464,#83465,
#83466,#83467,#83468,#83469,#83470,#83471,#83472,#83473,#83474,#83475,#83476,
#83477,#83478,#83479,#83480,#83481,#83482,#83483,#83484,#83485,#83486,#83487,
#83488,#83489,#83490,#83491,#83492,#83493,#83494,#83495,#83496,#83497,#83498,
#83499,#83500,#83501,#83502),.UNSPECIFIED.,.F.,.F.,(4,3,3,3,3,3,3,3,3,3,
3,3,3,3,3,3,3,3,3,3,3,4),(0.,0.0255635666326801,0.0511244793994705,0.076688080187019,
0.102251706962356,0.127821081108941,0.136940747823198,0.162571815981994,
0.188198561587646,0.213824971768371,0.239449499925226,0.265076549959684,
0.273881495646396,0.299440012611685,0.324995568541792,0.350553426157864,
0.376111105043384,0.401674288772044,0.410822243469594,0.43680646043743,
0.462785075549229,0.479292617177209),.UNSPECIFIED.);
#3579=B_SPLINE_CURVE_WITH_KNOTS('',3,(#83504,#83505,#83506,#83507,#83508,
#83509,#83510,#83511,#83512,#83513,#83514,#83515,#83516,#83517,#83518,#83519,
#83520,#83521,#83522,#83523,#83524,#83525,#83526,#83527,#83528,#83529,#83530,
#83531,#83532,#83533,#83534,#83535,#83536,#83537,#83538,#83539,#83540,#83541,
#83542,#83543,#83544,#83545,#83546,#83547,#83548,#83549,#83550,#83551,#83552,
#83553,#83554,#83555,#83556,#83557,#83558,#83559,#83560,#83561,#83562,#83563,
#83564,#83565,#83566,#83567),.UNSPECIFIED.,.F.,.F.,(4,3,3,3,3,3,3,3,3,3,
3,3,3,3,3,3,3,3,3,3,3,4),(0.479292617179906,0.505267046530367,0.531249287460817,
0.547756394224346,0.573317095800904,0.598872806297043,0.62442781629965,
0.649980909248029,0.675536979617555,0.684683947910693,0.71030857285459,
0.735930637841139,0.761554969027824,0.787178926838093,0.812807591189663,
0.82161150159704,0.847178127100071,0.872739574414869,0.89829997927434,0.923858250403141,
0.949419131562034,0.958539055283387),.UNSPECIFIED.);
#3580=B_SPLINE_CURVE_WITH_KNOTS('',3,(#83569,#83570,#83571,#83572,#83573,
#83574,#83575,#83576,#83577,#83578,#83579,#83580,#83581,#83582,#83583,#83584,
#83585,#83586,#83587,#83588,#83589,#83590,#83591,#83592,#83593,#83594,#83595,
#83596,#83597,#83598,#83599,#83600,#83601,#83602,#83603,#83604,#83605,#83606,
#83607,#83608,#83609,#83610,#83611,#83612,#83613,#83614,#83615,#83616,#83617,
#83618,#83619,#83620,#83621,#83622,#83623,#83624,#83625,#83626,#83627,#83628,
#83629,#83630,#83631,#83632,#83633,#83634,#83635,#83636,#83637,#83638,#83639,
#83640,#83641,#83642,#83643,#83644,#83645,#83646,#83647,#83648,#83649,#83650,
#83651,#83652,#83653,#83654,#83655,#83656,#83657,#83658,#83659,#83660,#83661,
#83662,#83663,#83664,#83665,#83666,#83667,#83668,#83669,#83670,#83671,#83672,
#83673,#83674,#83675,#83676,#83677,#83678,#83679,#83680,#83681,#83682,#83683,
#83684,#83685,#83686,#83687,#83688,#83689,#83690,#83691,#83692,#83693,#83694,
#83695),.UNSPECIFIED.,.F.,.F.,(4,3,3,3,3,3,3,3,3,3,3,3,3,3,3,3,3,3,3,3,
3,3,3,3,3,3,3,3,3,3,3,3,3,3,3,3,3,3,3,3,3,3,4),(0.,0.0257481533409456,0.0514946980789381,
0.0772436849279218,0.102992038986384,0.128743741659937,0.136934150754769,
0.162447594607815,0.187957321333388,0.213468628709931,0.238979446831854,
0.264495648410872,0.273868301509539,0.299485364667177,0.325097913405818,
0.350709964231731,0.376320073731763,0.401932716793888,0.410802452264308,
0.436387986336631,0.461970819036555,0.487556081452547,0.513141169428889,
0.538731557184643,0.547736603019078,0.573298539642115,0.598855488832839,
0.624411743116122,0.649966083470479,0.675523405962016,0.684670753773847,
0.710296552579017,0.735919791615974,0.761545298101024,0.787170432048045,
0.812800274548105,0.821604904528617,0.84717303404939,0.872735984507688,
0.898297889248134,0.92385765765822,0.949420030719154,0.958539055283386),
 .UNSPECIFIED.);
#3581=B_SPLINE_CURVE_WITH_KNOTS('',3,(#83696,#83697,#83698,#83699,#83700,
#83701,#83702,#83703,#83704,#83705,#83706,#83707,#83708,#83709,#83710,#83711,
#83712,#83713,#83714,#83715,#83716,#83717,#83718,#83719,#83720,#83721,#83722,
#83723,#83724,#83725,#83726,#83727,#83728,#83729,#83730,#83731,#83732,#83733,
#83734,#83735,#83736,#83737,#83738,#83739,#83740,#83741,#83742,#83743,#83744,
#83745,#83746,#83747,#83748,#83749,#83750,#83751,#83752,#83753,#83754,#83755,
#83756,#83757,#83758,#83759),.UNSPECIFIED.,.F.,.F.,(4,3,3,3,3,3,3,3,3,3,
3,3,3,3,3,3,3,3,3,3,3,4),(0.,0.0257491523438341,0.0514966921238077,0.0772466708701257,
0.102996015643584,0.128748709483213,0.136940747823198,0.162455615107776,
0.187966771796078,0.21347951743795,0.238991778112778,0.264509427354194,
0.273881495646396,0.299499762668791,0.325113511405751,0.350726757305157,
0.376338059087739,0.401951891032166,0.410822243469593,0.436536934850327,
0.462249829569396,0.47929261717721),.UNSPECIFIED.);
#3582=B_SPLINE_CURVE_WITH_KNOTS('',3,(#83765,#83766,#83767,#83768,#83769,
#83770,#83771,#83772,#83773,#83774,#83775,#83776,#83777,#83778,#83779,#83780,
#83781,#83782,#83783,#83784,#83785,#83786,#83787,#83788,#83789,#83790,#83791,
#83792,#83793,#83794,#83795,#83796,#83797,#83798,#83799,#83800,#83801,#83802,
#83803,#83804,#83805,#83806,#83807,#83808,#83809,#83810,#83811,#83812,#83813,
#83814,#83815,#83816,#83817,#83818,#83819,#83820,#83821,#83822,#83823,#83824,
#83825,#83826,#83827,#83828),.UNSPECIFIED.,.F.,.F.,(4,3,3,3,3,3,3,3,3,3,
3,3,3,3,3,3,3,3,3,3,3,4),(0.479292617177209,0.505000671870075,0.530712796156197,
0.547756394224347,0.573367607382753,0.598976259761798,0.624587301684935,
0.650198076948859,0.67581381494733,0.684683947910694,0.710200019009184,
0.735711164707781,0.761222093924401,0.786731491916345,0.812244747773555,
0.82161150159704,0.847360662097727,0.873106644909574,0.898852770635322,
0.924596931000677,0.950342531080525,0.958539055283387),.UNSPECIFIED.);
#3583=B_SPLINE_CURVE_WITH_KNOTS('',3,(#83830,#83831,#83832,#83833,#83834,
#83835,#83836,#83837,#83838,#83839,#83840,#83841,#83842,#83843,#83844,#83845,
#83846,#83847,#83848,#83849,#83850,#83851,#83852,#83853,#83854,#83855,#83856,
#83857,#83858,#83859,#83860,#83861,#83862,#83863,#83864,#83865,#83866,#83867,
#83868,#83869,#83870,#83871,#83872,#83873,#83874,#83875,#83876,#83877,#83878,
#83879,#83880,#83881,#83882,#83883,#83884,#83885,#83886,#83887,#83888,#83889,
#83890,#83891,#83892,#83893,#83894,#83895,#83896,#83897,#83898,#83899,#83900,
#83901,#83902,#83903,#83904,#83905,#83906,#83907,#83908,#83909,#83910,#83911,
#83912,#83913,#83914,#83915,#83916,#83917,#83918,#83919,#83920,#83921,#83922,
#83923,#83924,#83925,#83926,#83927,#83928,#83929,#83930,#83931,#83932,#83933,
#83934,#83935,#83936,#83937,#83938,#83939,#83940,#83941,#83942,#83943,#83944,
#83945,#83946,#83947,#83948,#83949,#83950,#83951,#83952,#83953,#83954,#83955,
#83956),.UNSPECIFIED.,.F.,.F.,(4,3,3,3,3,3,3,3,3,3,3,3,3,3,3,3,3,3,3,3,
3,3,3,3,3,3,3,3,3,3,3,3,3,3,3,3,3,3,3,3,3,3,4),(0.,0.0255614058406569,0.0511201411777619,
0.0766815478440569,0.102242973130247,0.127810141641151,0.13693415075477,
0.162564161855662,0.18818985595306,0.213815220313041,0.239438705376993,
0.265064714254088,0.273868301509539,0.299425520738351,0.324979792724313,
0.350536386846161,0.376092814257761,0.401654764016234,0.410802452264309,
0.436393134716681,0.461978999751451,0.487564165024772,0.513147341926946,
0.53873318350802,0.547736603019078,0.573349111543881,0.598959052713892,
0.624571373229419,0.650183420861739,0.675800421845165,0.684670753773848,
0.710187543876092,0.735699417010997,0.761211090428249,0.78672124330388,
0.81223527319308,0.821604904528618,0.847355917984526,0.873103755286946,
0.898851731942261,0.924597739210931,0.950345175843443,0.958539055283387),
 .UNSPECIFIED.);
#3584=B_SPLINE_CURVE_WITH_KNOTS('',3,(#83957,#83958,#83959,#83960,#83961,
#83962,#83963,#83964,#83965,#83966,#83967,#83968,#83969,#83970,#83971,#83972,
#83973,#83974,#83975,#83976,#83977,#83978,#83979,#83980,#83981,#83982,#83983,
#83984,#83985,#83986,#83987,#83988,#83989,#83990,#83991,#83992,#83993,#83994,
#83995,#83996,#83997,#83998,#83999,#84000,#84001,#84002,#84003,#84004,#84005,
#84006,#84007,#84008,#84009,#84010,#84011,#84012,#84013,#84014,#84015,#84016,
#84017,#84018,#84019,#84020),.UNSPECIFIED.,.F.,.F.,(4,3,3,3,3,3,3,3,3,3,
3,3,3,3,3,3,3,3,3,3,3,4),(0.,0.0255626373109835,0.0511226039897656,0.0766852421264175,
0.102247898883866,0.127816299142739,0.136940747823198,0.162571993699622,
0.188198922364561,0.213825521276229,0.239450240801314,0.265077484261085,
0.273881495646396,0.299439946143816,0.324995449256306,0.350553274616682,
0.376110933258725,0.401674114513703,0.410822243469594,0.436807692773927,
0.462787529398712,0.479292617174633),.UNSPECIFIED.);
#3585=B_SPLINE_CURVE_WITH_KNOTS('',3,(#84022,#84023,#84024,#84025,#84026,
#84027,#84028,#84029,#84030,#84031,#84032,#84033,#84034,#84035,#84036,#84037,
#84038,#84039,#84040,#84041,#84042,#84043,#84044,#84045,#84046,#84047,#84048,
#84049,#84050,#84051,#84052,#84053,#84054,#84055,#84056,#84057,#84058,#84059,
#84060,#84061,#84062,#84063,#84064,#84065,#84066,#84067,#84068,#84069,#84070,
#84071,#84072,#84073,#84074,#84075,#84076,#84077,#84078,#84079,#84080,#84081,
#84082,#84083,#84084,#84085),.UNSPECIFIED.,.F.,.F.,(4,3,3,3,3,3,3,3,3,3,
3,3,3,3,3,3,3,3,3,3,3,4),(0.47929261717721,0.505267152182088,0.531249499696255,
0.547756394224346,0.573317095142505,0.598872803757218,0.624427810106277,
0.649980898385333,0.675536962638426,0.684683947910693,0.710308590703365,
0.735930673424052,0.761555021973375,0.787178996872414,0.812807677753939,
0.82161150159704,0.84717804259122,0.872739405615204,0.898299727215526,0.923857915879837,
0.949418716310487,0.958539055283387),.UNSPECIFIED.);
#3586=B_SPLINE_CURVE_WITH_KNOTS('',3,(#84087,#84088,#84089,#84090,#84091,
#84092,#84093,#84094,#84095,#84096,#84097,#84098,#84099,#84100,#84101,#84102,
#84103,#84104,#84105,#84106,#84107,#84108,#84109,#84110,#84111,#84112,#84113,
#84114,#84115,#84116,#84117,#84118,#84119,#84120,#84121,#84122,#84123,#84124,
#84125,#84126,#84127,#84128,#84129,#84130,#84131,#84132,#84133,#84134,#84135,
#84136,#84137,#84138,#84139,#84140,#84141,#84142,#84143,#84144,#84145,#84146,
#84147,#84148,#84149,#84150,#84151,#84152,#84153,#84154,#84155,#84156,#84157,
#84158,#84159,#84160,#84161,#84162,#84163,#84164,#84165,#84166,#84167,#84168,
#84169,#84170,#84171,#84172,#84173,#84174,#84175,#84176,#84177,#84178,#84179,
#84180,#84181,#84182,#84183,#84184,#84185,#84186,#84187,#84188,#84189,#84190,
#84191,#84192,#84193,#84194,#84195,#84196,#84197,#84198,#84199,#84200,#84201,
#84202,#84203,#84204,#84205,#84206,#84207,#84208,#84209,#84210,#84211,#84212,
#84213),.UNSPECIFIED.,.F.,.F.,(4,3,3,3,3,3,3,3,3,3,3,3,3,3,3,3,3,3,3,3,
3,3,3,3,3,3,3,3,3,3,3,3,3,3,3,3,3,3,3,3,3,3,4),(0.,0.0257479118882393,0.0514942112903244,
0.0772429495412298,0.102991053849869,0.128742507063266,0.136934150754769,
0.162447788870315,0.1879577165684,0.213469233143456,0.238980264774859,0.264496684713239,
0.273868301509539,0.299485334381649,0.325097849185929,0.350709861176942,
0.376319929144802,0.401932527152614,0.410802452264308,0.436388087284282,
0.461971024086556,0.487556394413245,0.513141592275077,0.538732092072625,
0.547736603019078,0.57329853543293,0.59885547530275,0.6244117128732,0.649966032281209,
0.675523327806675,0.684670753773847,0.710296631142861,0.735919948316494,
0.761545531427997,0.787170740871235,0.812800656523678,0.821604904528617,
0.847172677299873,0.872735271851408,0.898296824929134,0.923856244968091,
0.94941827689922,0.958539055283386),.UNSPECIFIED.);
#3587=B_SPLINE_CURVE_WITH_KNOTS('',3,(#84214,#84215,#84216,#84217,#84218,
#84219,#84220,#84221,#84222,#84223,#84224,#84225,#84226,#84227,#84228,#84229,
#84230,#84231,#84232,#84233,#84234,#84235,#84236,#84237,#84238,#84239,#84240,
#84241,#84242,#84243,#84244,#84245,#84246,#84247,#84248,#84249,#84250,#84251,
#84252,#84253,#84254,#84255,#84256,#84257,#84258,#84259,#84260,#84261,#84262,
#84263,#84264,#84265,#84266,#84267,#84268,#84269,#84270,#84271,#84272,#84273,
#84274,#84275,#84276,#84277),.UNSPECIFIED.,.F.,.F.,(4,3,3,3,3,3,3,3,3,3,
3,3,3,3,3,3,3,3,3,3,3,4),(0.,0.0257484974013576,0.05149537221129,0.077244677886759,
0.102993346900836,0.128745366395548,0.136940747823198,0.162456127284197,
0.187967813632376,0.213481110331621,0.23899393326664,0.264512157330573,
0.273881495646396,0.29949970651347,0.325113389931437,0.350726558060159,
0.376337775174149,0.401951513305493,0.410822243469593,0.436536403375429,
0.462248777981185,0.47929261717721),.UNSPECIFIED.);
#3588=B_SPLINE_CURVE_WITH_KNOTS('',3,(#84285,#84286,#84287,#84288,#84289,
#84290),.UNSPECIFIED.,.F.,.F.,(4,2,4),(0.,0.216145052008235,0.432257670232604),
 .UNSPECIFIED.);
#3589=B_SPLINE_CURVE_WITH_KNOTS('',3,(#84292,#84293,#84294,#84295,#84296,
#84297,#84298,#84299,#84300,#84301,#84302,#84303,#84304,#84305,#84306,#84307,
#84308,#84309,#84310,#84311,#84312,#84313,#84314,#84315,#84316,#84317,#84318,
#84319,#84320,#84321,#84322,#84323,#84324,#84325,#84326,#84327,#84328,#84329,
#84330,#84331,#84332,#84333,#84334,#84335,#84336,#84337,#84338,#84339,#84340,
#84341,#84342,#84343,#84344,#84345,#84346,#84347,#84348,#84349,#84350,#84351,
#84352,#84353,#84354,#84355,#84356,#84357,#84358,#84359,#84360,#84361,#84362,
#84363,#84364,#84365,#84366,#84367,#84368,#84369,#84370,#84371,#84372,#84373,
#84374,#84375,#84376,#84377,#84378,#84379,#84380,#84381,#84382,#84383,#84384,
#84385,#84386,#84387,#84388,#84389,#84390,#84391,#84392,#84393,#84394,#84395,
#84396,#84397,#84398,#84399,#84400,#84401,#84402,#84403,#84404,#84405,#84406,
#84407,#84408,#84409,#84410,#84411,#84412,#84413,#84414,#84415,#84416,#84417,
#84418),.UNSPECIFIED.,.F.,.F.,(4,3,3,3,3,3,3,3,3,3,3,3,3,3,3,3,3,3,3,3,
3,3,3,3,3,3,3,3,3,3,3,3,3,3,3,3,3,3,3,3,3,3,4),(0.,0.0255606924572304,0.0511187002880486,
0.0766793648644971,0.102240041316473,0.127806456428402,0.13693415075477,
0.162564246062696,0.18819002867775,0.213815486626741,0.239439067836035,
0.265065175540469,0.273868301509539,0.299425486139408,0.324979735220857,
0.350536323838371,0.376092755852858,0.401654724993392,0.410802452264309,
0.436393374733914,0.461979476717824,0.487564872613919,0.513148275975265,
0.538734336496269,0.547736603019078,0.573349050106841,0.59895893629183,
0.624571212136073,0.650183221308245,0.675800193454039,0.684670753773848,
0.710188054217764,0.735700429024432,0.761212587338756,0.786723214354636,
0.812237699421663,0.821604904528618,0.847355305604822,0.873102528839054,
0.898849894994097,0.924595295694261,0.950342136178106,0.958539055283387),
 .UNSPECIFIED.);
#3590=B_SPLINE_CURVE_WITH_KNOTS('',3,(#84419,#84420,#84421,#84422,#84423,
#84424,#84425,#84426,#84427,#84428,#84429,#84430,#84431,#84432,#84433,#84434,
#84435,#84436,#84437,#84438,#84439,#84440,#84441,#84442,#84443,#84444,#84445,
#84446,#84447,#84448,#84449,#84450,#84451,#84452,#84453,#84454,#84455,#84456,
#84457,#84458,#84459,#84460,#84461,#84462,#84463,#84464,#84465,#84466,#84467,
#84468,#84469,#84470,#84471,#84472,#84473,#84474,#84475,#84476,#84477,#84478,
#84479,#84480,#84481,#84482),.UNSPECIFIED.,.F.,.F.,(4,3,3,3,3,3,3,3,3,3,
3,3,3,3,3,3,3,3,3,3,3,4),(0.,0.0255619238931804,0.0511211630306363,0.0766830590417173,
0.102244966928892,0.127812613752488,0.136940747823198,0.162572077910745,
0.188199095097715,0.213825787602894,0.239450603277954,0.265077945569875,
0.273881495646396,0.299439911543206,0.324995391750202,0.350553211605967,
0.376110874851102,0.401674075489097,0.410822243469594,0.436808654596317,
0.46278944530477,0.479292617174629),.UNSPECIFIED.);
#3591=B_SPLINE_CURVE_WITH_KNOTS('',3,(#84484,#84485,#84486,#84487,#84488,
#84489,#84490,#84491,#84492,#84493,#84494,#84495,#84496,#84497,#84498,#84499,
#84500,#84501,#84502,#84503,#84504,#84505,#84506,#84507,#84508,#84509,#84510,
#84511,#84512,#84513,#84514,#84515,#84516,#84517,#84518,#84519,#84520,#84521,
#84522,#84523,#84524,#84525,#84526,#84527,#84528,#84529,#84530,#84531,#84532,
#84533,#84534,#84535,#84536,#84537,#84538,#84539,#84540,#84541,#84542,#84543,
#84544,#84545,#84546,#84547),.UNSPECIFIED.,.F.,.F.,(4,3,3,3,3,3,3,3,3,3,
3,3,3,3,3,3,3,3,3,3,3,4),(0.47929261717721,0.505268272173354,0.531251749094228,
0.547756394224346,0.57331710180848,0.598872803689831,0.62442778376179,0.649980834522848,
0.675536845133206,0.684683947910693,0.710308747141793,0.735930984531055,
0.761555483271823,0.787179605223059,0.812808427118386,0.82161150159704,
0.84717715204078,0.872737627590923,0.898297073699267,0.923854395875952,
0.949414349001511,0.958539055283387),.UNSPECIFIED.);
#3592=B_SPLINE_CURVE_WITH_KNOTS('',3,(#84549,#84550,#84551,#84552,#84553,
#84554,#84555,#84556,#84557,#84558,#84559,#84560,#84561,#84562,#84563,#84564,
#84565,#84566,#84567,#84568,#84569,#84570,#84571,#84572,#84573,#84574,#84575,
#84576,#84577,#84578,#84579,#84580,#84581,#84582,#84583,#84584,#84585,#84586,
#84587,#84588,#84589,#84590,#84591,#84592,#84593,#84594,#84595,#84596,#84597,
#84598,#84599,#84600,#84601,#84602,#84603,#84604,#84605,#84606,#84607,#84608,
#84609,#84610,#84611,#84612,#84613,#84614,#84615,#84616,#84617,#84618,#84619,
#84620,#84621,#84622,#84623,#84624,#84625,#84626,#84627,#84628,#84629,#84630,
#84631,#84632,#84633,#84634,#84635,#84636,#84637,#84638,#84639,#84640,#84641,
#84642,#84643,#84644,#84645,#84646,#84647,#84648,#84649,#84650,#84651,#84652,
#84653,#84654,#84655,#84656,#84657,#84658,#84659,#84660,#84661,#84662,#84663,
#84664,#84665,#84666,#84667,#84668,#84669,#84670,#84671,#84672,#84673,#84674,
#84675),.UNSPECIFIED.,.F.,.F.,(4,3,3,3,3,3,3,3,3,3,3,3,3,3,3,3,3,3,3,3,
3,3,3,3,3,3,3,3,3,3,3,3,3,3,3,3,3,3,3,3,3,3,4),(0.,0.0257472569772838,0.0514928914413629,
0.0772409566538184,0.102988385235593,0.12873916413656,0.136934150754769,
0.162448301022051,0.187958758354364,0.213470825960218,0.23898241982469,
0.264499414557891,0.273868301509539,0.299485278229076,0.325097727717576,
0.350709661941676,0.376319645244957,0.401932149444248,0.410802452264308,
0.436388343469677,0.461971544040781,0.487557187203235,0.513142662573877,
0.538733444881708,0.547736603019078,0.573298542099209,0.598855475235286,
0.624411686527281,0.649965968415386,0.675523210295452,0.684670753773847,
0.710296787588882,0.735920259438635,0.76154599274883,0.78717134925136,0.812801405924429,
0.821604904528617,0.847171786706504,0.872733493741441,0.898294171285005,
0.923852724794528,0.949413909379723,0.958539055283386),.UNSPECIFIED.);
#3593=B_SPLINE_CURVE_WITH_KNOTS('',3,(#84676,#84677,#84678,#84679,#84680,
#84681,#84682,#84683,#84684,#84685,#84686,#84687,#84688,#84689,#84690,#84691,
#84692,#84693,#84694,#84695,#84696,#84697,#84698,#84699,#84700,#84701,#84702,
#84703,#84704,#84705,#84706,#84707,#84708,#84709,#84710,#84711,#84712,#84713,
#84714,#84715,#84716,#84717,#84718,#84719,#84720,#84721,#84722,#84723,#84724,
#84725,#84726,#84727,#84728,#84729,#84730,#84731,#84732,#84733,#84734,#84735,
#84736,#84737,#84738,#84739),.UNSPECIFIED.,.F.,.F.,(4,3,3,3,3,3,3,3,3,3,
3,3,3,3,3,3,3,3,3,3,3,4),(0.,0.0257479279250796,0.0514942251218129,0.0772429470007209,
0.102991030381649,0.128742466196639,0.136940747823198,0.162456557033928,
0.187968687603579,0.213482446206961,0.238995740295273,0.264514445849957,
0.273881495646396,0.299499689255512,0.325113348199751,0.350726481849042,
0.376337658878936,0.401951349310238,0.410822243469593,0.436535985935545,
0.462247951405,0.47929261717721),.UNSPECIFIED.);
#3594=B_SPLINE_CURVE_WITH_KNOTS('',3,(#84742,#84743,#84744,#84745,#84746,
#84747,#84748,#84749,#84750,#84751,#84752,#84753,#84754,#84755,#84756,#84757,
#84758,#84759,#84760,#84761,#84762,#84763,#84764,#84765,#84766,#84767,#84768,
#84769,#84770,#84771,#84772,#84773,#84774,#84775,#84776,#84777,#84778,#84779,
#84780,#84781),.UNSPECIFIED.,.F.,.F.,(4,3,3,3,3,3,3,3,3,3,3,3,3,4),(0.479292617179918,
0.505270201534281,0.531255614881935,0.547759154438251,0.573320916637539,
0.598877661713949,0.624433668411704,0.649987736156769,0.675544750003459,
0.684692228552392,0.710230981397045,0.735766124290673,0.761303447116751,
0.780281286407365),.UNSPECIFIED.);
#3595=B_SPLINE_CURVE_WITH_KNOTS('',3,(#84786,#84787,#84788,#84789,#84790,
#84791,#84792,#84793,#84794,#84795,#84796,#84797,#84798,#84799,#84800,#84801,
#84802,#84803,#84804,#84805,#84806,#84807,#84808,#84809,#84810,#84811,#84812,
#84813,#84814,#84815,#84816,#84817,#84818,#84819,#84820,#84821,#84822),
 .UNSPECIFIED.,.F.,.F.,(4,3,3,3,3,3,3,3,3,3,3,3,4),(-0.587674682252879,
-0.522275543829995,-0.458090181278496,-0.394772087238499,-0.332851241040222,
-0.290582655255106,-0.278920555202013,-0.270271621870392,-0.211810705909702,
-0.154597029996384,-0.0981542104956995,-0.0429508698655889,0.),
 .UNSPECIFIED.);
#3596=B_SPLINE_CURVE_WITH_KNOTS('',3,(#84824,#84825,#84826,#84827,#84828,
#84829,#84830,#84831,#84832,#84833,#84834,#84835,#84836,#84837,#84838,#84839,
#84840,#84841,#84842,#84843,#84844,#84845,#84846,#84847,#84848,#84849,#84850,
#84851,#84852,#84853,#84854,#84855,#84856,#84857,#84858,#84859,#84860,#84861,
#84862,#84863,#84864,#84865,#84866,#84867,#84868,#84869,#84870,#84871,#84872,
#84873,#84874,#84875,#84876,#84877,#84878,#84879,#84880,#84881,#84882,#84883,
#84884,#84885,#84886,#84887,#84888,#84889,#84890,#84891,#84892,#84893,#84894,
#84895,#84896,#84897,#84898,#84899,#84900,#84901,#84902,#84903,#84904,#84905,
#84906,#84907,#84908,#84909,#84910,#84911,#84912,#84913,#84914,#84915,#84916,
#84917,#84918,#84919,#84920,#84921,#84922,#84923,#84924,#84925,#84926,#84927,
#84928,#84929,#84930,#84931,#84932,#84933,#84934,#84935,#84936,#84937,#84938,
#84939,#84940,#84941),.UNSPECIFIED.,.F.,.F.,(4,3,3,3,3,3,3,3,3,3,3,3,3,
3,3,3,3,3,3,3,3,3,3,3,3,3,3,3,3,3,3,3,3,3,3,3,3,3,3,4),(-2.21853380163141,
-2.14169700900979,-2.06000622499644,-1.98211684071596,-1.94032109877607,
-1.92940218041483,-1.89664180199272,-1.81493387295641,-1.73704918283534,
-1.65550918141576,-1.64157430304436,-1.63094960942268,-1.55302694654912,
-1.47530023545016,-1.410889177157,-1.33294761057228,-1.25462606115837,-1.23895063150748,
-1.22943147765607,-1.21204834416161,-1.13439080518558,-1.05606095724006,
-0.977636631083868,-0.899720638530548,-0.825388030509179,-0.812979956321517,
-0.734650421044989,-0.656887708961902,-0.602390206445073,-0.524409242543717,
-0.460391483368985,-0.43238371373004,-0.413066499848313,-0.402820754727463,
-0.325843178167182,-0.247449175911852,-0.169023585066473,-0.0906453771061667,
-0.01226716914586,-3.85504356227988E-5),.UNSPECIFIED.);
#3597=B_SPLINE_CURVE_WITH_KNOTS('',3,(#84944,#84945,#84946,#84947,#84948,
#84949,#84950,#84951,#84952,#84953,#84954,#84955,#84956,#84957,#84958,#84959,
#84960,#84961,#84962,#84963,#84964,#84965,#84966,#84967,#84968,#84969,#84970,
#84971,#84972,#84973,#84974,#84975,#84976,#84977,#84978,#84979,#84980,#84981,
#84982,#84983,#84984,#84985,#84986,#84987,#84988,#84989),.UNSPECIFIED.,
 .F.,.F.,(4,3,3,3,3,3,3,3,3,3,3,3,3,3,3,4),(-0.593406414910134,-0.551632623974457,
-0.508637403999538,-0.476718450480326,-0.455431999029698,-0.441536524705485,
-0.395342652559364,-0.347935919259055,-0.308483973940118,-0.294081551185092,
-0.243706144295089,-0.192379500820218,-0.139588002045789,-0.0860358862173692,
-0.0315002188398129,0.),.UNSPECIFIED.);
#3598=B_SPLINE_CURVE_WITH_KNOTS('',3,(#84990,#84991,#84992,#84993,#84994,
#84995,#84996,#84997,#84998,#84999,#85000,#85001,#85002,#85003,#85004,#85005,
#85006,#85007,#85008,#85009,#85010,#85011,#85012,#85013,#85014,#85015,#85016,
#85017,#85018,#85019,#85020,#85021,#85022,#85023,#85024,#85025,#85026),
 .UNSPECIFIED.,.F.,.F.,(4,3,3,3,3,3,3,3,3,3,3,3,4),(-0.47345883347035,-0.421785176279112,
-0.371368479159938,-0.321739753842847,-0.273397162061595,-0.229764201701003,
-0.222185125570855,-0.176965222652948,-0.132800326254763,-0.0998029709030014,
-0.057155654322561,-0.0156176608406257,-1.17079676490498E-5),
 .UNSPECIFIED.);
#3599=B_SPLINE_CURVE_WITH_KNOTS('',3,(#85087,#85088,#85089,#85090,#85091,
#85092,#85093,#85094),.UNSPECIFIED.,.F.,.F.,(4,1,1,1,1,4),(0.144829272278474,
0.266996519095835,0.389163765913196,0.633498259547918,0.877832753182639,
1.),.UNSPECIFIED.);
#3600=B_SPLINE_CURVE_WITH_KNOTS('',3,(#85129,#85130,#85131,#85132,#85133,
#85134,#85135,#85136,#85137,#85138,#85139,#85140,#85141,#85142,#85143,#85144,
#85145,#85146,#85147),.UNSPECIFIED.,.F.,.F.,(4,3,3,3,3,3,4),(0.815535452893383,
0.847523529162131,0.877832753182639,0.913211852549041,0.948843428238211,
0.98416694468468,1.),.UNSPECIFIED.);
#3601=B_SPLINE_CURVE_WITH_KNOTS('',3,(#85151,#85152,#85153,#85154,#85155,
#85156,#85157,#85158,#85159,#85160,#85161,#85162,#85163,#85164,#85165,#85166,
#85167,#85168,#85169,#85170,#85171,#85172,#85173,#85174,#85175,#85176,#85177,
#85178,#85179,#85180,#85181,#85182,#85183,#85184,#85185,#85186,#85187),
 .UNSPECIFIED.,.F.,.F.,(4,3,3,3,3,3,3,3,3,3,3,3,4),(-0.473459590222709,
-0.421790762051377,-0.37138598180264,-0.321768833120639,-0.273433624494914,
-0.229795000551108,-0.221386012412719,-0.176179340889983,-0.132023266728005,
-0.099803605201648,-0.0571527054274905,-0.0156155844320621,-1.1601141627616E-5),
 .UNSPECIFIED.);
#3602=B_SPLINE_CURVE_WITH_KNOTS('',3,(#85189,#85190,#85191,#85192,#85193,
#85194,#85195,#85196,#85197,#85198,#85199,#85200,#85201,#85202,#85203,#85204,
#85205,#85206,#85207,#85208,#85209,#85210,#85211,#85212,#85213,#85214,#85215,
#85216,#85217,#85218,#85219,#85220,#85221,#85222),.UNSPECIFIED.,.F.,.F.,
(4,3,3,3,3,3,3,3,3,3,3,4),(-0.587778750364654,-0.522392013442643,-0.458246883948291,
-0.39497298076002,-0.333146586530125,-0.280267059023603,-0.270271030376407,
-0.21181010441986,-0.154596418410281,-0.0981535891351624,-0.0429502360987486,
0.),.UNSPECIFIED.);
#3603=B_SPLINE_CURVE_WITH_KNOTS('',3,(#85224,#85225,#85226,#85227,#85228,
#85229,#85230,#85231,#85232,#85233,#85234,#85235,#85236,#85237,#85238,#85239,
#85240,#85241,#85242,#85243,#85244,#85245,#85246,#85247,#85248,#85249,#85250,
#85251,#85252,#85253,#85254,#85255,#85256,#85257,#85258,#85259,#85260,#85261,
#85262,#85263,#85264,#85265,#85266,#85267,#85268,#85269,#85270,#85271,#85272,
#85273,#85274,#85275,#85276,#85277,#85278,#85279,#85280,#85281,#85282,#85283,
#85284,#85285,#85286,#85287,#85288,#85289,#85290,#85291,#85292,#85293,#85294,
#85295,#85296,#85297,#85298,#85299,#85300,#85301,#85302,#85303,#85304,#85305,
#85306,#85307,#85308,#85309,#85310,#85311,#85312,#85313,#85314,#85315,#85316,
#85317,#85318,#85319,#85320,#85321,#85322,#85323,#85324,#85325,#85326,#85327,
#85328,#85329,#85330,#85331,#85332,#85333,#85334,#85335,#85336,#85337,#85338,
#85339,#85340,#85341),.UNSPECIFIED.,.F.,.F.,(4,3,3,3,3,3,3,3,3,3,3,3,3,
3,3,3,3,3,3,3,3,3,3,3,3,3,3,3,3,3,3,3,3,3,3,3,3,3,3,4),(-2.21853380163141,
-2.14147687580222,-2.05984115648833,-1.98219940142569,-1.94038305070594,
-1.92982950632801,-1.90569661828717,-1.82789475155552,-1.81493399854668,
-1.73723203187215,-1.65564638113919,-1.64262516049492,-1.63166177462369,
-1.55405438820831,-1.47598659309221,-1.4108894289403,-1.33296387367606,
-1.25559958045839,-1.2374200788259,-1.22345195044101,-1.14563978964884,
-1.06790309904323,-1.00663999520165,-0.928722650056018,-0.850384574996885,
-0.829262259425257,-0.819802210939349,-0.798261686933839,-0.720531563347699,
-0.642165018867216,-0.563716269145714,-0.485760922111857,-0.413856073237234,
-0.404560305583847,-0.326120745631757,-0.248239195955339,-0.198141526613365,
-0.120433480757384,-0.0425282133148996,0.),.UNSPECIFIED.);
#3604=B_SPLINE_CURVE_WITH_KNOTS('',3,(#85344,#85345,#85346,#85347,#85348,
#85349,#85350,#85351,#85352,#85353,#85354,#85355,#85356,#85357,#85358,#85359,
#85360,#85361,#85362,#85363,#85364,#85365,#85366,#85367,#85368,#85369,#85370,
#85371,#85372,#85373,#85374,#85375,#85376,#85377,#85378,#85379,#85380,#85381,
#85382,#85383,#85384,#85385,#85386,#85387,#85388,#85389,#85390,#85391,#85392),
 .UNSPECIFIED.,.F.,.F.,(4,3,3,3,3,3,3,3,3,3,3,3,3,3,3,3,4),(-0.593405610245497,
-0.551428083606103,-0.508498879669832,-0.476717699690467,-0.458169903899235,
-0.442929634384365,-0.396892175868468,-0.34991960007854,-0.31930222027659,
-0.303005267879666,-0.289328418066246,-0.238863157543073,-0.187445469095536,
-0.134580054596664,-0.0809600612898856,-0.0263940066113425,0.),
 .UNSPECIFIED.);
#3605=B_SPLINE_CURVE_WITH_KNOTS('',3,(#85432,#85433,#85434,#85435,#85436,
#85437,#85438,#85439,#85440,#85441,#85442,#85443,#85444,#85445,#85446,#85447,
#85448,#85449,#85450,#85451,#85452,#85453),.UNSPECIFIED.,.F.,.F.,(4,3,3,
3,3,3,3,4),(0.,0.0333176175948162,0.0669610730078588,0.100473730255888,
0.12216720883009,0.147816659999738,0.173346358925325,0.184428015042582),
 .UNSPECIFIED.);
#3606=B_SPLINE_CURVE_WITH_KNOTS('',3,(#85456,#85457,#85458,#85459,#85460,
#85461,#85462,#85463,#85464),.UNSPECIFIED.,.F.,.F.,(4,1,1,1,1,1,4),(0.,
0.12216720883009,0.24433441766018,0.488668835320359,0.610836044150449,0.733003252980539,
0.855170461810629),.UNSPECIFIED.);
#3607=B_SPLINE_CURVE_WITH_KNOTS('',3,(#85524,#85525,#85526,#85527,#85528,
#85529,#85530,#85531,#85532,#85533),.UNSPECIFIED.,.F.,.F.,(4,1,1,1,1,1,
1,4),(0.,0.142857142857143,0.285714285714286,0.428571428571429,0.571428571428571,
0.714285714285714,0.857142857142857,1.),.UNSPECIFIED.);
#3608=B_SPLINE_CURVE_WITH_KNOTS('',3,(#85602,#85603,#85604,#85605,#85606,
#85607,#85608,#85609,#85610,#85611),.UNSPECIFIED.,.F.,.F.,(4,1,1,1,1,1,
1,4),(0.,0.142857142857143,0.285714285714286,0.428571428571429,0.571428571428571,
0.714285714285714,0.857142857142857,1.),.UNSPECIFIED.);
#3609=B_SPLINE_CURVE_WITH_KNOTS('',3,(#85697,#85698,#85699,#85700,#85701,
#85702,#85703,#85704,#85705,#85706),.UNSPECIFIED.,.F.,.F.,(4,1,1,1,1,1,
1,4),(0.,0.142857142857143,0.285714285714286,0.428571428571429,0.571428571428571,
0.714285714285714,0.857142857142857,1.),.UNSPECIFIED.);
#3610=B_SPLINE_CURVE_WITH_KNOTS('',3,(#85751,#85752,#85753,#85754,#85755,
#85756,#85757,#85758,#85759,#85760),.UNSPECIFIED.,.F.,.F.,(4,1,1,1,1,1,
1,4),(0.,0.142857142857143,0.285714285714286,0.428571428571429,0.571428571428571,
0.714285714285714,0.857142857142857,1.),.UNSPECIFIED.);
#3611=B_SPLINE_CURVE_WITH_KNOTS('',3,(#85847,#85848,#85849,#85850,#85851,
#85852,#85853,#85854,#85855,#85856),.UNSPECIFIED.,.F.,.F.,(4,1,1,1,1,1,
1,4),(0.,0.142857142857143,0.285714285714286,0.428571428571429,0.571428571428571,
0.714285714285714,0.857142857142857,1.),.UNSPECIFIED.);
#3612=B_SPLINE_CURVE_WITH_KNOTS('',3,(#85901,#85902,#85903,#85904,#85905,
#85906,#85907,#85908,#85909,#85910,#85911,#85912,#85913,#85914,#85915,#85916,
#85917,#85918),.UNSPECIFIED.,.F.,.F.,(4,2,2,2,2,2,2,2,4),(0.,0.411606409146398,
0.882606331055097,1.58532698900216,2.58333249194717,3.58155989188507,4.32087044195073,
4.8178921514512,5.24318392699258),.UNSPECIFIED.);
#3613=B_SPLINE_CURVE_WITH_KNOTS('',3,(#86005,#86006,#86007,#86008,#86009,
#86010,#86011,#86012,#86013,#86014,#86015,#86016,#86017,#86018,#86019,#86020,
#86021,#86022,#86023,#86024,#86025,#86026),.UNSPECIFIED.,.F.,.F.,(4,3,3,
3,3,3,3,4),(0.,0.142857142857143,0.285714285714286,0.428571428571429,0.571428571428571,
0.714285714285714,0.857142857142857,1.),.UNSPECIFIED.);
#3614=B_SPLINE_CURVE_WITH_KNOTS('',3,(#86071,#86072,#86073,#86074,#86075,
#86076,#86077,#86078,#86079,#86080),.UNSPECIFIED.,.F.,.F.,(4,1,1,1,1,1,
1,4),(0.,0.142857142857143,0.285714285714286,0.428571428571429,0.571428571428571,
0.714285714285714,0.857142857142857,1.),.UNSPECIFIED.);
#3615=B_SPLINE_CURVE_WITH_KNOTS('',3,(#86167,#86168,#86169,#86170,#86171,
#86172,#86173,#86174,#86175,#86176,#86177,#86178,#86179,#86180,#86181,#86182,
#86183,#86184,#86185,#86186,#86187,#86188),.UNSPECIFIED.,.F.,.F.,(4,3,3,
3,3,3,3,4),(0.,0.142857142857143,0.285714285714286,0.428571428571429,0.571428571428571,
0.714285714285714,0.857142857142857,1.),.UNSPECIFIED.);
#3616=B_SPLINE_CURVE_WITH_KNOTS('',3,(#86233,#86234,#86235,#86236,#86237,
#86238,#86239,#86240,#86241,#86242),.UNSPECIFIED.,.F.,.F.,(4,1,1,1,1,1,
1,4),(0.,0.142857142857143,0.285714285714286,0.428571428571429,0.571428571428571,
0.714285714285714,0.857142857142857,1.),.UNSPECIFIED.);
#3617=B_SPLINE_CURVE_WITH_KNOTS('',3,(#86383,#86384,#86385,#86386,#86387,
#86388,#86389,#86390,#86391,#86392),.UNSPECIFIED.,.F.,.F.,(4,1,1,1,1,1,
1,4),(0.,0.142857142857143,0.285714285714286,0.428571428571429,0.571428571428571,
0.714285714285714,0.857142857142857,1.),.UNSPECIFIED.);
#3618=B_SPLINE_CURVE_WITH_KNOTS('',3,(#86433,#86434,#86435,#86436,#86437,
#86438,#86439,#86440,#86441,#86442),.UNSPECIFIED.,.F.,.F.,(4,1,1,1,1,1,
1,4),(0.,0.142857142857143,0.285714285714286,0.428571428571429,0.571428571428571,
0.714285714285714,0.857142857142857,1.),.UNSPECIFIED.);
#3619=B_SPLINE_CURVE_WITH_KNOTS('',3,(#86523,#86524,#86525,#86526,#86527,
#86528,#86529,#86530,#86531,#86532),.UNSPECIFIED.,.F.,.F.,(4,1,1,1,1,1,
1,4),(0.,0.142857142857143,0.285714285714286,0.428571428571429,0.571428571428571,
0.714285714285714,0.857142857142857,1.),.UNSPECIFIED.);
#3620=B_SPLINE_CURVE_WITH_KNOTS('',3,(#86573,#86574,#86575,#86576,#86577,
#86578,#86579,#86580,#86581,#86582,#86583,#86584,#86585,#86586,#86587,#86588,
#86589,#86590),.UNSPECIFIED.,.F.,.F.,(4,2,2,2,2,2,2,2,4),(0.,0.411606409146402,
0.882606331055175,1.58532698900237,2.58333249194715,3.5815598918848,4.32087044194964,
4.8178921514492,5.24318392698968),.UNSPECIFIED.);
#3621=B_SPLINE_CURVE_WITH_KNOTS('',3,(#86671,#86672,#86673,#86674,#86675,
#86676,#86677,#86678,#86679,#86680,#86681,#86682,#86683,#86684,#86685,#86686,
#86687,#86688),.UNSPECIFIED.,.F.,.F.,(4,2,2,2,2,2,2,2,4),(-5.06897673155691,
-4.67104605560332,-4.21569535708223,-3.5363229670094,-2.57147642457375,
-1.60641534306576,-0.891668820224186,-0.411161088211719,0.),
 .UNSPECIFIED.);
#3622=B_SPLINE_CURVE_WITH_KNOTS('',3,(#86729,#86730,#86731,#86732,#86733,
#86734,#86735,#86736,#86737,#86738),.UNSPECIFIED.,.F.,.F.,(4,1,1,1,1,1,
1,4),(0.,0.142857142857143,0.285714285714286,0.428571428571429,0.571428571428571,
0.714285714285714,0.857142857142857,1.),.UNSPECIFIED.);
#3623=B_SPLINE_CURVE_WITH_KNOTS('',3,(#86819,#86820,#86821,#86822,#86823,
#86824,#86825,#86826,#86827,#86828,#86829,#86830,#86831,#86832,#86833,#86834,
#86835,#86836,#86837,#86838,#86839,#86840),.UNSPECIFIED.,.F.,.F.,(4,3,3,
3,3,3,3,4),(0.,0.142857142857143,0.285714285714286,0.428571428571429,0.571428571428571,
0.714285714285714,0.857142857142857,1.),.UNSPECIFIED.);
#3624=B_SPLINE_CURVE_WITH_KNOTS('',3,(#86881,#86882,#86883,#86884,#86885,
#86886,#86887,#86888,#86889,#86890),.UNSPECIFIED.,.F.,.F.,(4,1,1,1,1,1,
1,4),(0.,0.142857142857143,0.285714285714286,0.428571428571429,0.571428571428571,
0.714285714285714,0.857142857142857,1.),.UNSPECIFIED.);
#3625=B_SPLINE_CURVE_WITH_KNOTS('',3,(#86971,#86972,#86973,#86974,#86975,
#86976,#86977,#86978,#86979,#86980,#86981,#86982,#86983,#86984,#86985,#86986,
#86987,#86988,#86989,#86990,#86991,#86992),.UNSPECIFIED.,.F.,.F.,(4,3,3,
3,3,3,3,4),(0.,0.142857142857143,0.285714285714286,0.428571428571429,0.571428571428571,
0.714285714285714,0.857142857142857,1.),.UNSPECIFIED.);
#3626=B_SPLINE_CURVE_WITH_KNOTS('',3,(#87033,#87034,#87035,#87036,#87037,
#87038,#87039,#87040,#87041,#87042),.UNSPECIFIED.,.F.,.F.,(4,1,1,1,1,1,
1,4),(0.,0.142857142857143,0.285714285714286,0.428571428571429,0.571428571428571,
0.714285714285714,0.857142857142857,1.),.UNSPECIFIED.);
#3985=LINE('',#81963,#4455);
#3986=LINE('',#82209,#4456);
#3987=LINE('',#82727,#4457);
#3988=LINE('',#83245,#4458);
#3989=LINE('',#83763,#4459);
#3990=LINE('',#84281,#4460);
#3991=LINE('',#85045,#4461);
#3992=LINE('',#85095,#4462);
#3993=LINE('',#85148,#4463);
#3994=LINE('',#85455,#4464);
#3995=LINE('',#85481,#4465);
#3996=LINE('',#85523,#4466);
#3997=LINE('',#85537,#4467);
#3998=LINE('',#85540,#4468);
#3999=LINE('',#85559,#4469);
#4000=LINE('',#85600,#4470);
#4001=LINE('',#85612,#4471);
#4002=LINE('',#85653,#4472);
#4003=LINE('',#85695,#4473);
#4004=LINE('',#85707,#4474);
#4005=LINE('',#85749,#4475);
#4006=LINE('',#85761,#4476);
#4007=LINE('',#85802,#4477);
#4008=LINE('',#85803,#4478);
#4009=LINE('',#85845,#4479);
#4010=LINE('',#85857,#4480);
#4011=LINE('',#85899,#4481);
#4012=LINE('',#85919,#4482);
#4013=LINE('',#85960,#4483);
#4014=LINE('',#85961,#4484);
#4015=LINE('',#86003,#4485);
#4016=LINE('',#86027,#4486);
#4017=LINE('',#86069,#4487);
#4018=LINE('',#86081,#4488);
#4019=LINE('',#86122,#4489);
#4020=LINE('',#86123,#4490);
#4021=LINE('',#86165,#4491);
#4022=LINE('',#86189,#4492);
#4023=LINE('',#86231,#4493);
#4024=LINE('',#86243,#4494);
#4025=LINE('',#86284,#4495);
#4026=LINE('',#86285,#4496);
#4027=LINE('',#86302,#4497);
#4455=VECTOR('',#16095,6.);
#4456=VECTOR('',#16100,6.);
#4457=VECTOR('',#16103,6.);
#4458=VECTOR('',#16106,6.);
#4459=VECTOR('',#16109,6.);
#4460=VECTOR('',#16112,6.);
#4461=VECTOR('',#16125,20.);
#4462=VECTOR('',#16126,20.);
#4463=VECTOR('',#16127,20.);
#4464=VECTOR('',#16134,20.);
#4465=VECTOR('',#16135,20.);
#4466=VECTOR('',#16136,20.);
#4467=VECTOR('',#16141,4.5);
#4468=VECTOR('',#16144,4.5);
#4469=VECTOR('',#16149,20.);
#4470=VECTOR('',#16150,20.);
#4471=VECTOR('',#16151,20.);
#4472=VECTOR('',#16152,20.);
#4473=VECTOR('',#16153,20.);
#4474=VECTOR('',#16154,20.);
#4475=VECTOR('',#16155,20.);
#4476=VECTOR('',#16156,20.);
#4477=VECTOR('',#16157,20.);
#4478=VECTOR('',#16158,20.);
#4479=VECTOR('',#16159,20.);
#4480=VECTOR('',#16160,20.);
#4481=VECTOR('',#16161,20.);
#4482=VECTOR('',#16162,20.);
#4483=VECTOR('',#16163,20.);
#4484=VECTOR('',#16164,20.);
#4485=VECTOR('',#16165,20.);
#4486=VECTOR('',#16166,20.);
#4487=VECTOR('',#16167,20.);
#4488=VECTOR('',#16168,20.);
#4489=VECTOR('',#16169,20.);
#4490=VECTOR('',#16170,20.);
#4491=VECTOR('',#16171,20.);
#4492=VECTOR('',#16172,20.);
#4493=VECTOR('',#16173,20.);
#4494=VECTOR('',#16174,20.);
#4495=VECTOR('',#16175,20.);
#4496=VECTOR('',#16176,20.);
#4497=VECTOR('',#16177,20.);
#5665=VERTEX_POINT('',#81961);
#5666=VERTEX_POINT('',#81962);
#5667=VERTEX_POINT('',#81964);
#5668=VERTEX_POINT('',#82029);
#5669=VERTEX_POINT('',#82133);
#5670=VERTEX_POINT('',#82135);
#5671=VERTEX_POINT('',#82207);
#5672=VERTEX_POINT('',#82208);
#5673=VERTEX_POINT('',#82210);
#5674=VERTEX_POINT('',#82275);
#5675=VERTEX_POINT('',#82467);
#5676=VERTEX_POINT('',#82532);
#5677=VERTEX_POINT('',#82725);
#5678=VERTEX_POINT('',#82726);
#5679=VERTEX_POINT('',#82728);
#5680=VERTEX_POINT('',#82793);
#5681=VERTEX_POINT('',#82985);
#5682=VERTEX_POINT('',#83050);
#5683=VERTEX_POINT('',#83243);
#5684=VERTEX_POINT('',#83244);
#5685=VERTEX_POINT('',#83246);
#5686=VERTEX_POINT('',#83311);
#5687=VERTEX_POINT('',#83503);
#5688=VERTEX_POINT('',#83568);
#5689=VERTEX_POINT('',#83761);
#5690=VERTEX_POINT('',#83762);
#5691=VERTEX_POINT('',#83764);
#5692=VERTEX_POINT('',#83829);
#5693=VERTEX_POINT('',#84021);
#5694=VERTEX_POINT('',#84086);
#5695=VERTEX_POINT('',#84279);
#5696=VERTEX_POINT('',#84280);
#5697=VERTEX_POINT('',#84282);
#5698=VERTEX_POINT('',#84284);
#5699=VERTEX_POINT('',#84291);
#5700=VERTEX_POINT('',#84483);
#5701=VERTEX_POINT('',#84548);
#5702=VERTEX_POINT('',#84741);
#5703=VERTEX_POINT('',#84784);
#5704=VERTEX_POINT('',#84785);
#5705=VERTEX_POINT('',#84823);
#5706=VERTEX_POINT('',#84942);
#5707=VERTEX_POINT('',#85027);
#5708=VERTEX_POINT('',#85086);
#5709=VERTEX_POINT('',#85128);
#5710=VERTEX_POINT('',#85150);
#5711=VERTEX_POINT('',#85188);
#5712=VERTEX_POINT('',#85223);
#5713=VERTEX_POINT('',#85342);
#5714=VERTEX_POINT('',#85393);
#5715=VERTEX_POINT('',#85431);
#5716=VERTEX_POINT('',#85454);
#5717=VERTEX_POINT('',#85522);
#5718=VERTEX_POINT('',#85535);
#5719=VERTEX_POINT('',#85539);
#5720=VERTEX_POINT('',#85601);
#5721=VERTEX_POINT('',#85694);
#5722=VERTEX_POINT('',#85696);
#5723=VERTEX_POINT('',#85748);
#5724=VERTEX_POINT('',#85750);
#5725=VERTEX_POINT('',#85844);
#5726=VERTEX_POINT('',#85846);
#5727=VERTEX_POINT('',#85898);
#5728=VERTEX_POINT('',#85900);
#5729=VERTEX_POINT('',#86002);
#5730=VERTEX_POINT('',#86004);
#5731=VERTEX_POINT('',#86068);
#5732=VERTEX_POINT('',#86070);
#5733=VERTEX_POINT('',#86164);
#5734=VERTEX_POINT('',#86166);
#5735=VERTEX_POINT('',#86230);
#5736=VERTEX_POINT('',#86232);
#7491=EDGE_CURVE('',#5665,#5666,#3985,.T.);
#7492=EDGE_CURVE('',#5665,#5667,#3560,.T.);
#7493=EDGE_CURVE('',#5667,#5668,#3561,.T.);
#7494=EDGE_CURVE('',#5668,#5669,#2618,.T.);
#7495=EDGE_CURVE('',#5669,#5670,#3562,.T.);
#7496=EDGE_CURVE('',#5670,#5666,#3563,.T.);
#7497=EDGE_CURVE('',#5671,#5672,#3986,.T.);
#7498=EDGE_CURVE('',#5671,#5673,#3564,.T.);
#7499=EDGE_CURVE('',#5673,#5674,#3565,.T.);
#7500=EDGE_CURVE('',#5674,#5665,#3566,.T.);
#7501=EDGE_CURVE('',#5666,#5675,#3567,.T.);
#7502=EDGE_CURVE('',#5675,#5676,#3568,.T.);
#7503=EDGE_CURVE('',#5676,#5672,#3569,.T.);
#7504=EDGE_CURVE('',#5677,#5678,#3987,.T.);
#7505=EDGE_CURVE('',#5677,#5679,#3570,.T.);
#7506=EDGE_CURVE('',#5679,#5680,#3571,.T.);
#7507=EDGE_CURVE('',#5680,#5671,#3572,.T.);
#7508=EDGE_CURVE('',#5672,#5681,#3573,.T.);
#7509=EDGE_CURVE('',#5681,#5682,#3574,.T.);
#7510=EDGE_CURVE('',#5682,#5678,#3575,.T.);
#7511=EDGE_CURVE('',#5683,#5684,#3988,.T.);
#7512=EDGE_CURVE('',#5683,#5685,#3576,.T.);
#7513=EDGE_CURVE('',#5685,#5686,#3577,.T.);
#7514=EDGE_CURVE('',#5686,#5677,#3578,.T.);
#7515=EDGE_CURVE('',#5678,#5687,#3579,.T.);
#7516=EDGE_CURVE('',#5687,#5688,#3580,.T.);
#7517=EDGE_CURVE('',#5688,#5684,#3581,.T.);
#7518=EDGE_CURVE('',#5689,#5690,#3989,.T.);
#7519=EDGE_CURVE('',#5689,#5691,#3582,.T.);
#7520=EDGE_CURVE('',#5691,#5692,#3583,.T.);
#7521=EDGE_CURVE('',#5692,#5683,#3584,.T.);
#7522=EDGE_CURVE('',#5684,#5693,#3585,.T.);
#7523=EDGE_CURVE('',#5693,#5694,#3586,.T.);
#7524=EDGE_CURVE('',#5694,#5690,#3587,.T.);
#7525=EDGE_CURVE('',#5695,#5696,#3990,.T.);
#7526=EDGE_CURVE('',#5695,#5697,#2619,.T.);
#7527=EDGE_CURVE('',#5697,#5698,#3588,.T.);
#7528=EDGE_CURVE('',#5698,#5699,#3589,.T.);
#7529=EDGE_CURVE('',#5699,#5689,#3590,.T.);
#7530=EDGE_CURVE('',#5690,#5700,#3591,.T.);
#7531=EDGE_CURVE('',#5700,#5701,#3592,.T.);
#7532=EDGE_CURVE('',#5701,#5696,#3593,.T.);
#7533=EDGE_CURVE('',#5696,#5702,#3594,.T.);
#7534=EDGE_CURVE('',#5702,#5695,#2620,.T.);
#7535=EDGE_CURVE('',#5703,#5704,#3595,.T.);
#7536=EDGE_CURVE('',#5705,#5703,#3596,.T.);
#7537=EDGE_CURVE('',#5706,#5705,#238,.T.);
#7538=EDGE_CURVE('',#5669,#5706,#3597,.T.);
#7539=EDGE_CURVE('',#5704,#5668,#3598,.T.);
#7540=EDGE_CURVE('',#5707,#5707,#2621,.T.);
#7541=EDGE_CURVE('',#5670,#5706,#3991,.T.);
#7542=EDGE_CURVE('',#5705,#5708,#3599,.T.);
#7543=EDGE_CURVE('',#5675,#5708,#3992,.T.);
#7544=EDGE_CURVE('',#5703,#5709,#3600,.T.);
#7545=EDGE_CURVE('',#5708,#5709,#3993,.T.);
#7546=EDGE_CURVE('',#5710,#5702,#3601,.T.);
#7547=EDGE_CURVE('',#5711,#5710,#3602,.T.);
#7548=EDGE_CURVE('',#5712,#5711,#3603,.T.);
#7549=EDGE_CURVE('',#5713,#5712,#239,.T.);
#7550=EDGE_CURVE('',#5697,#5713,#3604,.T.);
#7551=EDGE_CURVE('',#5714,#5714,#2622,.T.);
#7552=EDGE_CURVE('',#5715,#5711,#3605,.T.);
#7553=EDGE_CURVE('',#5715,#5716,#3994,.T.);
#7554=EDGE_CURVE('',#5716,#5712,#3606,.T.);
#7555=EDGE_CURVE('',#5710,#5715,#3995,.T.);
#7556=EDGE_CURVE('',#5701,#5717,#3996,.T.);
#7557=EDGE_CURVE('',#5717,#5715,#3607,.T.);
#7558=EDGE_CURVE('',#5718,#5718,#2623,.T.);
#7559=EDGE_CURVE('',#5718,#5707,#3997,.T.);
#7560=EDGE_CURVE('',#5714,#5719,#3998,.T.);
#7561=EDGE_CURVE('',#5719,#5719,#2624,.T.);
#7562=EDGE_CURVE('',#5713,#5698,#3999,.T.);
#7563=EDGE_CURVE('',#5716,#5699,#4000,.T.);
#7564=EDGE_CURVE('',#5720,#5716,#3608,.T.);
#7565=EDGE_CURVE('',#5720,#5691,#4001,.T.);
#7566=EDGE_CURVE('',#5717,#5720,#4002,.T.);
#7567=EDGE_CURVE('',#5694,#5721,#4003,.T.);
#7568=EDGE_CURVE('',#5721,#5722,#3609,.T.);
#7569=EDGE_CURVE('',#5700,#5722,#4004,.T.);
#7570=EDGE_CURVE('',#5723,#5692,#4005,.T.);
#7571=EDGE_CURVE('',#5724,#5723,#3610,.T.);
#7572=EDGE_CURVE('',#5724,#5685,#4006,.T.);
#7573=EDGE_CURVE('',#5721,#5724,#4007,.T.);
#7574=EDGE_CURVE('',#5722,#5723,#4008,.T.);
#7575=EDGE_CURVE('',#5688,#5725,#4009,.T.);
#7576=EDGE_CURVE('',#5725,#5726,#3611,.T.);
#7577=EDGE_CURVE('',#5693,#5726,#4010,.T.);
#7578=EDGE_CURVE('',#5727,#5686,#4011,.T.);
#7579=EDGE_CURVE('',#5728,#5727,#3612,.T.);
#7580=EDGE_CURVE('',#5728,#5679,#4012,.T.);
#7581=EDGE_CURVE('',#5725,#5728,#4013,.T.);
#7582=EDGE_CURVE('',#5726,#5727,#4014,.T.);
#7583=EDGE_CURVE('',#5682,#5729,#4015,.T.);
#7584=EDGE_CURVE('',#5729,#5730,#3613,.T.);
#7585=EDGE_CURVE('',#5687,#5730,#4016,.T.);
#7586=EDGE_CURVE('',#5731,#5680,#4017,.T.);
#7587=EDGE_CURVE('',#5732,#5731,#3614,.T.);
#7588=EDGE_CURVE('',#5732,#5673,#4018,.T.);
#7589=EDGE_CURVE('',#5729,#5732,#4019,.T.);
#7590=EDGE_CURVE('',#5730,#5731,#4020,.T.);
#7591=EDGE_CURVE('',#5676,#5733,#4021,.T.);
#7592=EDGE_CURVE('',#5733,#5734,#3615,.T.);
#7593=EDGE_CURVE('',#5681,#5734,#4022,.T.);
#7594=EDGE_CURVE('',#5735,#5674,#4023,.T.);
#7595=EDGE_CURVE('',#5736,#5735,#3616,.T.);
#7596=EDGE_CURVE('',#5736,#5667,#4024,.T.);
#7597=EDGE_CURVE('',#5733,#5736,#4025,.T.);
#7598=EDGE_CURVE('',#5734,#5735,#4026,.T.);
#7599=EDGE_CURVE('',#5709,#5704,#4027,.T.);
#7600=EDGE_CURVE('',#5722,#5717,#3617,.T.);
#7601=EDGE_CURVE('',#5723,#5720,#3618,.T.);
#7602=EDGE_CURVE('',#5726,#5721,#3619,.T.);
#7603=EDGE_CURVE('',#5727,#5724,#3620,.T.);
#7604=EDGE_CURVE('',#5730,#5725,#3621,.T.);
#7605=EDGE_CURVE('',#5731,#5728,#3622,.T.);
#7606=EDGE_CURVE('',#5734,#5729,#3623,.T.);
#7607=EDGE_CURVE('',#5735,#5732,#3624,.T.);
#7608=EDGE_CURVE('',#5708,#5733,#3625,.T.);
#7609=EDGE_CURVE('',#5709,#5736,#3626,.T.);
#10958=ORIENTED_EDGE('',*,*,#7491,.F.);
#10959=ORIENTED_EDGE('',*,*,#7492,.T.);
#10960=ORIENTED_EDGE('',*,*,#7493,.T.);
#10961=ORIENTED_EDGE('',*,*,#7494,.T.);
#10962=ORIENTED_EDGE('',*,*,#7495,.T.);
#10963=ORIENTED_EDGE('',*,*,#7496,.T.);
#10964=ORIENTED_EDGE('',*,*,#7497,.F.);
#10965=ORIENTED_EDGE('',*,*,#7498,.T.);
#10966=ORIENTED_EDGE('',*,*,#7499,.T.);
#10967=ORIENTED_EDGE('',*,*,#7500,.T.);
#10968=ORIENTED_EDGE('',*,*,#7491,.T.);
#10969=ORIENTED_EDGE('',*,*,#7501,.T.);
#10970=ORIENTED_EDGE('',*,*,#7502,.T.);
#10971=ORIENTED_EDGE('',*,*,#7503,.T.);
#10972=ORIENTED_EDGE('',*,*,#7504,.F.);
#10973=ORIENTED_EDGE('',*,*,#7505,.T.);
#10974=ORIENTED_EDGE('',*,*,#7506,.T.);
#10975=ORIENTED_EDGE('',*,*,#7507,.T.);
#10976=ORIENTED_EDGE('',*,*,#7497,.T.);
#10977=ORIENTED_EDGE('',*,*,#7508,.T.);
#10978=ORIENTED_EDGE('',*,*,#7509,.T.);
#10979=ORIENTED_EDGE('',*,*,#7510,.T.);
#10980=ORIENTED_EDGE('',*,*,#7511,.F.);
#10981=ORIENTED_EDGE('',*,*,#7512,.T.);
#10982=ORIENTED_EDGE('',*,*,#7513,.T.);
#10983=ORIENTED_EDGE('',*,*,#7514,.T.);
#10984=ORIENTED_EDGE('',*,*,#7504,.T.);
#10985=ORIENTED_EDGE('',*,*,#7515,.T.);
#10986=ORIENTED_EDGE('',*,*,#7516,.T.);
#10987=ORIENTED_EDGE('',*,*,#7517,.T.);
#10988=ORIENTED_EDGE('',*,*,#7518,.F.);
#10989=ORIENTED_EDGE('',*,*,#7519,.T.);
#10990=ORIENTED_EDGE('',*,*,#7520,.T.);
#10991=ORIENTED_EDGE('',*,*,#7521,.T.);
#10992=ORIENTED_EDGE('',*,*,#7511,.T.);
#10993=ORIENTED_EDGE('',*,*,#7522,.T.);
#10994=ORIENTED_EDGE('',*,*,#7523,.T.);
#10995=ORIENTED_EDGE('',*,*,#7524,.T.);
#10996=ORIENTED_EDGE('',*,*,#7525,.F.);
#10997=ORIENTED_EDGE('',*,*,#7526,.T.);
#10998=ORIENTED_EDGE('',*,*,#7527,.T.);
#10999=ORIENTED_EDGE('',*,*,#7528,.T.);
#11000=ORIENTED_EDGE('',*,*,#7529,.T.);
#11001=ORIENTED_EDGE('',*,*,#7518,.T.);
#11002=ORIENTED_EDGE('',*,*,#7530,.T.);
#11003=ORIENTED_EDGE('',*,*,#7531,.T.);
#11004=ORIENTED_EDGE('',*,*,#7532,.T.);
#11005=ORIENTED_EDGE('',*,*,#7525,.T.);
#11006=ORIENTED_EDGE('',*,*,#7533,.T.);
#11007=ORIENTED_EDGE('',*,*,#7534,.T.);
#11008=ORIENTED_EDGE('',*,*,#7535,.F.);
#11009=ORIENTED_EDGE('',*,*,#7536,.F.);
#11010=ORIENTED_EDGE('',*,*,#7537,.F.);
#11011=ORIENTED_EDGE('',*,*,#7538,.F.);
#11012=ORIENTED_EDGE('',*,*,#7494,.F.);
#11013=ORIENTED_EDGE('',*,*,#7539,.F.);
#11014=ORIENTED_EDGE('',*,*,#7540,.F.);
#11015=ORIENTED_EDGE('',*,*,#7538,.T.);
#11016=ORIENTED_EDGE('',*,*,#7541,.F.);
#11017=ORIENTED_EDGE('',*,*,#7495,.F.);
#11018=ORIENTED_EDGE('',*,*,#7537,.T.);
#11019=ORIENTED_EDGE('',*,*,#7542,.T.);
#11020=ORIENTED_EDGE('',*,*,#7543,.F.);
#11021=ORIENTED_EDGE('',*,*,#7501,.F.);
#11022=ORIENTED_EDGE('',*,*,#7496,.F.);
#11023=ORIENTED_EDGE('',*,*,#7541,.T.);
#11024=ORIENTED_EDGE('',*,*,#7536,.T.);
#11025=ORIENTED_EDGE('',*,*,#7544,.T.);
#11026=ORIENTED_EDGE('',*,*,#7545,.F.);
#11027=ORIENTED_EDGE('',*,*,#7542,.F.);
#11028=ORIENTED_EDGE('',*,*,#7534,.F.);
#11029=ORIENTED_EDGE('',*,*,#7546,.F.);
#11030=ORIENTED_EDGE('',*,*,#7547,.F.);
#11031=ORIENTED_EDGE('',*,*,#7548,.F.);
#11032=ORIENTED_EDGE('',*,*,#7549,.F.);
#11033=ORIENTED_EDGE('',*,*,#7550,.F.);
#11034=ORIENTED_EDGE('',*,*,#7526,.F.);
#11035=ORIENTED_EDGE('',*,*,#7551,.T.);
#11036=ORIENTED_EDGE('',*,*,#7548,.T.);
#11037=ORIENTED_EDGE('',*,*,#7552,.F.);
#11038=ORIENTED_EDGE('',*,*,#7553,.T.);
#11039=ORIENTED_EDGE('',*,*,#7554,.T.);
#11040=ORIENTED_EDGE('',*,*,#7547,.T.);
#11041=ORIENTED_EDGE('',*,*,#7555,.T.);
#11042=ORIENTED_EDGE('',*,*,#7552,.T.);
#11043=ORIENTED_EDGE('',*,*,#7546,.T.);
#11044=ORIENTED_EDGE('',*,*,#7533,.F.);
#11045=ORIENTED_EDGE('',*,*,#7532,.F.);
#11046=ORIENTED_EDGE('',*,*,#7556,.T.);
#11047=ORIENTED_EDGE('',*,*,#7557,.T.);
#11048=ORIENTED_EDGE('',*,*,#7555,.F.);
#11049=ORIENTED_EDGE('',*,*,#7558,.F.);
#11050=ORIENTED_EDGE('',*,*,#7559,.T.);
#11051=ORIENTED_EDGE('',*,*,#7540,.T.);
#11052=ORIENTED_EDGE('',*,*,#7559,.F.);
#11053=ORIENTED_EDGE('',*,*,#7551,.F.);
#11054=ORIENTED_EDGE('',*,*,#7560,.T.);
#11055=ORIENTED_EDGE('',*,*,#7561,.F.);
#11056=ORIENTED_EDGE('',*,*,#7560,.F.);
#11057=ORIENTED_EDGE('',*,*,#7561,.T.);
#11058=ORIENTED_EDGE('',*,*,#7550,.T.);
#11059=ORIENTED_EDGE('',*,*,#7562,.T.);
#11060=ORIENTED_EDGE('',*,*,#7527,.F.);
#11061=ORIENTED_EDGE('',*,*,#7529,.F.);
#11062=ORIENTED_EDGE('',*,*,#7563,.F.);
#11063=ORIENTED_EDGE('',*,*,#7564,.F.);
#11064=ORIENTED_EDGE('',*,*,#7565,.T.);
#11065=ORIENTED_EDGE('',*,*,#7519,.F.);
#11066=ORIENTED_EDGE('',*,*,#7566,.T.);
#11067=ORIENTED_EDGE('',*,*,#7564,.T.);
#11068=ORIENTED_EDGE('',*,*,#7553,.F.);
#11069=ORIENTED_EDGE('',*,*,#7557,.F.);
#11070=ORIENTED_EDGE('',*,*,#7524,.F.);
#11071=ORIENTED_EDGE('',*,*,#7567,.T.);
#11072=ORIENTED_EDGE('',*,*,#7568,.T.);
#11073=ORIENTED_EDGE('',*,*,#7569,.F.);
#11074=ORIENTED_EDGE('',*,*,#7530,.F.);
#11075=ORIENTED_EDGE('',*,*,#7521,.F.);
#11076=ORIENTED_EDGE('',*,*,#7570,.F.);
#11077=ORIENTED_EDGE('',*,*,#7571,.F.);
#11078=ORIENTED_EDGE('',*,*,#7572,.T.);
#11079=ORIENTED_EDGE('',*,*,#7512,.F.);
#11080=ORIENTED_EDGE('',*,*,#7573,.T.);
#11081=ORIENTED_EDGE('',*,*,#7571,.T.);
#11082=ORIENTED_EDGE('',*,*,#7574,.F.);
#11083=ORIENTED_EDGE('',*,*,#7568,.F.);
#11084=ORIENTED_EDGE('',*,*,#7517,.F.);
#11085=ORIENTED_EDGE('',*,*,#7575,.T.);
#11086=ORIENTED_EDGE('',*,*,#7576,.T.);
#11087=ORIENTED_EDGE('',*,*,#7577,.F.);
#11088=ORIENTED_EDGE('',*,*,#7522,.F.);
#11089=ORIENTED_EDGE('',*,*,#7514,.F.);
#11090=ORIENTED_EDGE('',*,*,#7578,.F.);
#11091=ORIENTED_EDGE('',*,*,#7579,.F.);
#11092=ORIENTED_EDGE('',*,*,#7580,.T.);
#11093=ORIENTED_EDGE('',*,*,#7505,.F.);
#11094=ORIENTED_EDGE('',*,*,#7581,.T.);
#11095=ORIENTED_EDGE('',*,*,#7579,.T.);
#11096=ORIENTED_EDGE('',*,*,#7582,.F.);
#11097=ORIENTED_EDGE('',*,*,#7576,.F.);
#11098=ORIENTED_EDGE('',*,*,#7510,.F.);
#11099=ORIENTED_EDGE('',*,*,#7583,.T.);
#11100=ORIENTED_EDGE('',*,*,#7584,.T.);
#11101=ORIENTED_EDGE('',*,*,#7585,.F.);
#11102=ORIENTED_EDGE('',*,*,#7515,.F.);
#11103=ORIENTED_EDGE('',*,*,#7507,.F.);
#11104=ORIENTED_EDGE('',*,*,#7586,.F.);
#11105=ORIENTED_EDGE('',*,*,#7587,.F.);
#11106=ORIENTED_EDGE('',*,*,#7588,.T.);
#11107=ORIENTED_EDGE('',*,*,#7498,.F.);
#11108=ORIENTED_EDGE('',*,*,#7589,.T.);
#11109=ORIENTED_EDGE('',*,*,#7587,.T.);
#11110=ORIENTED_EDGE('',*,*,#7590,.F.);
#11111=ORIENTED_EDGE('',*,*,#7584,.F.);
#11112=ORIENTED_EDGE('',*,*,#7503,.F.);
#11113=ORIENTED_EDGE('',*,*,#7591,.T.);
#11114=ORIENTED_EDGE('',*,*,#7592,.T.);
#11115=ORIENTED_EDGE('',*,*,#7593,.F.);
#11116=ORIENTED_EDGE('',*,*,#7508,.F.);
#11117=ORIENTED_EDGE('',*,*,#7500,.F.);
#11118=ORIENTED_EDGE('',*,*,#7594,.F.);
#11119=ORIENTED_EDGE('',*,*,#7595,.F.);
#11120=ORIENTED_EDGE('',*,*,#7596,.T.);
#11121=ORIENTED_EDGE('',*,*,#7492,.F.);
#11122=ORIENTED_EDGE('',*,*,#7597,.T.);
#11123=ORIENTED_EDGE('',*,*,#7595,.T.);
#11124=ORIENTED_EDGE('',*,*,#7598,.F.);
#11125=ORIENTED_EDGE('',*,*,#7592,.F.);
#11126=ORIENTED_EDGE('',*,*,#7535,.T.);
#11127=ORIENTED_EDGE('',*,*,#7599,.F.);
#11128=ORIENTED_EDGE('',*,*,#7544,.F.);
#11129=ORIENTED_EDGE('',*,*,#7549,.T.);
#11130=ORIENTED_EDGE('',*,*,#7554,.F.);
#11131=ORIENTED_EDGE('',*,*,#7563,.T.);
#11132=ORIENTED_EDGE('',*,*,#7528,.F.);
#11133=ORIENTED_EDGE('',*,*,#7562,.F.);
#11134=ORIENTED_EDGE('',*,*,#7531,.F.);
#11135=ORIENTED_EDGE('',*,*,#7569,.T.);
#11136=ORIENTED_EDGE('',*,*,#7600,.T.);
#11137=ORIENTED_EDGE('',*,*,#7556,.F.);
#11138=ORIENTED_EDGE('',*,*,#7520,.F.);
#11139=ORIENTED_EDGE('',*,*,#7565,.F.);
#11140=ORIENTED_EDGE('',*,*,#7601,.F.);
#11141=ORIENTED_EDGE('',*,*,#7570,.T.);
#11142=ORIENTED_EDGE('',*,*,#7574,.T.);
#11143=ORIENTED_EDGE('',*,*,#7601,.T.);
#11144=ORIENTED_EDGE('',*,*,#7566,.F.);
#11145=ORIENTED_EDGE('',*,*,#7600,.F.);
#11146=ORIENTED_EDGE('',*,*,#7523,.F.);
#11147=ORIENTED_EDGE('',*,*,#7577,.T.);
#11148=ORIENTED_EDGE('',*,*,#7602,.T.);
#11149=ORIENTED_EDGE('',*,*,#7567,.F.);
#11150=ORIENTED_EDGE('',*,*,#7513,.F.);
#11151=ORIENTED_EDGE('',*,*,#7572,.F.);
#11152=ORIENTED_EDGE('',*,*,#7603,.F.);
#11153=ORIENTED_EDGE('',*,*,#7578,.T.);
#11154=ORIENTED_EDGE('',*,*,#7582,.T.);
#11155=ORIENTED_EDGE('',*,*,#7603,.T.);
#11156=ORIENTED_EDGE('',*,*,#7573,.F.);
#11157=ORIENTED_EDGE('',*,*,#7602,.F.);
#11158=ORIENTED_EDGE('',*,*,#7516,.F.);
#11159=ORIENTED_EDGE('',*,*,#7585,.T.);
#11160=ORIENTED_EDGE('',*,*,#7604,.T.);
#11161=ORIENTED_EDGE('',*,*,#7575,.F.);
#11162=ORIENTED_EDGE('',*,*,#7506,.F.);
#11163=ORIENTED_EDGE('',*,*,#7580,.F.);
#11164=ORIENTED_EDGE('',*,*,#7605,.F.);
#11165=ORIENTED_EDGE('',*,*,#7586,.T.);
#11166=ORIENTED_EDGE('',*,*,#7590,.T.);
#11167=ORIENTED_EDGE('',*,*,#7605,.T.);
#11168=ORIENTED_EDGE('',*,*,#7581,.F.);
#11169=ORIENTED_EDGE('',*,*,#7604,.F.);
#11170=ORIENTED_EDGE('',*,*,#7509,.F.);
#11171=ORIENTED_EDGE('',*,*,#7593,.T.);
#11172=ORIENTED_EDGE('',*,*,#7606,.T.);
#11173=ORIENTED_EDGE('',*,*,#7583,.F.);
#11174=ORIENTED_EDGE('',*,*,#7499,.F.);
#11175=ORIENTED_EDGE('',*,*,#7588,.F.);
#11176=ORIENTED_EDGE('',*,*,#7607,.F.);
#11177=ORIENTED_EDGE('',*,*,#7594,.T.);
#11178=ORIENTED_EDGE('',*,*,#7598,.T.);
#11179=ORIENTED_EDGE('',*,*,#7607,.T.);
#11180=ORIENTED_EDGE('',*,*,#7589,.F.);
#11181=ORIENTED_EDGE('',*,*,#7606,.F.);
#11182=ORIENTED_EDGE('',*,*,#7502,.F.);
#11183=ORIENTED_EDGE('',*,*,#7543,.T.);
#11184=ORIENTED_EDGE('',*,*,#7608,.T.);
#11185=ORIENTED_EDGE('',*,*,#7591,.F.);
#11186=ORIENTED_EDGE('',*,*,#7539,.T.);
#11187=ORIENTED_EDGE('',*,*,#7493,.F.);
#11188=ORIENTED_EDGE('',*,*,#7596,.F.);
#11189=ORIENTED_EDGE('',*,*,#7609,.F.);
#11190=ORIENTED_EDGE('',*,*,#7599,.T.);
#11191=ORIENTED_EDGE('',*,*,#7545,.T.);
#11192=ORIENTED_EDGE('',*,*,#7609,.T.);
#11193=ORIENTED_EDGE('',*,*,#7597,.F.);
#11194=ORIENTED_EDGE('',*,*,#7608,.F.);
#11195=ORIENTED_EDGE('',*,*,#7558,.T.);
#12236=CYLINDRICAL_SURFACE('',#13829,6.);
#12237=CYLINDRICAL_SURFACE('',#13831,6.);
#12238=CYLINDRICAL_SURFACE('',#13832,6.);
#12239=CYLINDRICAL_SURFACE('',#13833,6.);
#12240=CYLINDRICAL_SURFACE('',#13834,6.);
#12241=CYLINDRICAL_SURFACE('',#13835,6.);
#12242=CYLINDRICAL_SURFACE('',#13837,6.);
#12243=CYLINDRICAL_SURFACE('',#13845,4.5);
#12244=CYLINDRICAL_SURFACE('',#13847,4.5);
#12726=ADVANCED_FACE('',(#1196),#12236,.T.);
#12727=ADVANCED_FACE('',(#1197),#12237,.T.);
#12728=ADVANCED_FACE('',(#1198),#12238,.T.);
#12729=ADVANCED_FACE('',(#1199),#12239,.T.);
#12730=ADVANCED_FACE('',(#1200),#12240,.T.);
#12731=ADVANCED_FACE('',(#1201),#12241,.T.);
#12732=ADVANCED_FACE('',(#1202),#12242,.T.);
#12733=ADVANCED_FACE('',(#1203,#366),#519,.F.);
#12734=ADVANCED_FACE('',(#1204),#758,.T.);
#12735=ADVANCED_FACE('',(#1205),#759,.T.);
#12736=ADVANCED_FACE('',(#1206),#760,.T.);
#12737=ADVANCED_FACE('',(#1207,#367),#520,.T.);
#12738=ADVANCED_FACE('',(#1208),#761,.T.);
#12739=ADVANCED_FACE('',(#1209),#762,.T.);
#12740=ADVANCED_FACE('',(#1210),#763,.T.);
#12741=ADVANCED_FACE('',(#1211),#12243,.T.);
#12742=ADVANCED_FACE('',(#1212),#12244,.T.);
#12743=ADVANCED_FACE('',(#1213),#521,.T.);
#12744=ADVANCED_FACE('',(#1214),#764,.T.);
#12745=ADVANCED_FACE('',(#1215),#765,.T.);
#12746=ADVANCED_FACE('',(#1216),#766,.T.);
#12747=ADVANCED_FACE('',(#1217),#767,.T.);
#12748=ADVANCED_FACE('',(#1218),#768,.T.);
#12749=ADVANCED_FACE('',(#1219),#769,.T.);
#12750=ADVANCED_FACE('',(#1220),#770,.T.);
#12751=ADVANCED_FACE('',(#1221),#771,.T.);
#12752=ADVANCED_FACE('',(#1222),#772,.T.);
#12753=ADVANCED_FACE('',(#1223),#773,.T.);
#12754=ADVANCED_FACE('',(#1224),#774,.T.);
#12755=ADVANCED_FACE('',(#1225),#775,.T.);
#12756=ADVANCED_FACE('',(#1226),#776,.T.);
#12757=ADVANCED_FACE('',(#1227),#777,.T.);
#12758=ADVANCED_FACE('',(#1228),#778,.T.);
#12759=ADVANCED_FACE('',(#1229),#779,.T.);
#12760=ADVANCED_FACE('',(#1230),#780,.T.);
#12761=ADVANCED_FACE('',(#1231),#781,.T.);
#12762=ADVANCED_FACE('',(#1232),#782,.T.);
#12763=ADVANCED_FACE('',(#1233),#783,.T.);
#12764=ADVANCED_FACE('',(#1234),#784,.T.);
#12765=ADVANCED_FACE('',(#1235),#785,.T.);
#12766=ADVANCED_FACE('',(#1236),#786,.T.);
#12767=ADVANCED_FACE('',(#1237),#787,.T.);
#12768=ADVANCED_FACE('',(#1238),#788,.T.);
#12769=ADVANCED_FACE('',(#1239),#789,.T.);
#12770=ADVANCED_FACE('',(#1240),#790,.T.);
#12771=ADVANCED_FACE('',(#1241),#791,.T.);
#12772=ADVANCED_FACE('',(#1242),#792,.T.);
#12773=ADVANCED_FACE('',(#1243),#793,.T.);
#12774=ADVANCED_FACE('',(#1244),#794,.T.);
#12775=ADVANCED_FACE('',(#1245),#795,.T.);
#12776=ADVANCED_FACE('',(#1246),#522,.F.);
#12995=CLOSED_SHELL('',(#12726,#12727,#12728,#12729,#12730,#12731,#12732,
#12733,#12734,#12735,#12736,#12737,#12738,#12739,#12740,#12741,#12742,#12743,
#12744,#12745,#12746,#12747,#12748,#12749,#12750,#12751,#12752,#12753,#12754,
#12755,#12756,#12757,#12758,#12759,#12760,#12761,#12762,#12763,#12764,#12765,
#12766,#12767,#12768,#12769,#12770,#12771,#12772,#12773,#12774,#12775,#12776));
#13828=AXIS2_PLACEMENT_3D('',#81959,#16091,#16092);
#13829=AXIS2_PLACEMENT_3D('',#81960,#16093,#16094);
#13830=AXIS2_PLACEMENT_3D('',#82134,#16096,#16097);
#13831=AXIS2_PLACEMENT_3D('',#82206,#16098,#16099);
#13832=AXIS2_PLACEMENT_3D('',#82724,#16101,#16102);
#13833=AXIS2_PLACEMENT_3D('',#83242,#16104,#16105);
#13834=AXIS2_PLACEMENT_3D('',#83760,#16107,#16108);
#13835=AXIS2_PLACEMENT_3D('',#84278,#16110,#16111);
#13836=AXIS2_PLACEMENT_3D('',#84283,#16113,#16114);
#13837=AXIS2_PLACEMENT_3D('',#84740,#16115,#16116);
#13838=AXIS2_PLACEMENT_3D('',#84782,#16117,#16118);
#13839=AXIS2_PLACEMENT_3D('',#84783,#16119,#16120);
#13840=AXIS2_PLACEMENT_3D('',#84943,#16121,#16122);
#13841=AXIS2_PLACEMENT_3D('',#85028,#16123,#16124);
#13842=AXIS2_PLACEMENT_3D('',#85149,#16128,#16129);
#13843=AXIS2_PLACEMENT_3D('',#85343,#16130,#16131);
#13844=AXIS2_PLACEMENT_3D('',#85394,#16132,#16133);
#13845=AXIS2_PLACEMENT_3D('',#85534,#16137,#16138);
#13846=AXIS2_PLACEMENT_3D('',#85536,#16139,#16140);
#13847=AXIS2_PLACEMENT_3D('',#85538,#16142,#16143);
#13848=AXIS2_PLACEMENT_3D('',#85541,#16145,#16146);
#13849=AXIS2_PLACEMENT_3D('',#85542,#16147,#16148);
#13850=AXIS2_PLACEMENT_3D('',#87083,#16178,#16179);
#16091=DIRECTION('axis',(0.,0.,1.));
#16092=DIRECTION('refdir',(1.,0.,0.));
#16093=DIRECTION('center_axis',(1.,0.,0.));
#16094=DIRECTION('ref_axis',(0.,-0.707106781186547,0.707106781186547));
#16095=DIRECTION('',(-1.,0.,0.));
#16096=DIRECTION('center_axis',(1.,0.,0.));
#16097=DIRECTION('ref_axis',(0.,-0.707106781186547,0.707106781186547));
#16098=DIRECTION('center_axis',(1.,0.,0.));
#16099=DIRECTION('ref_axis',(0.,-0.707106781186547,0.707106781186547));
#16100=DIRECTION('',(-1.,0.,0.));
#16101=DIRECTION('center_axis',(1.,0.,0.));
#16102=DIRECTION('ref_axis',(0.,-0.707106781186547,0.707106781186547));
#16103=DIRECTION('',(-1.,0.,0.));
#16104=DIRECTION('center_axis',(1.,0.,0.));
#16105=DIRECTION('ref_axis',(0.,-0.707106781186547,0.707106781186547));
#16106=DIRECTION('',(-1.,0.,0.));
#16107=DIRECTION('center_axis',(1.,0.,0.));
#16108=DIRECTION('ref_axis',(0.,-0.707106781186547,0.707106781186547));
#16109=DIRECTION('',(-1.,0.,0.));
#16110=DIRECTION('center_axis',(1.,0.,0.));
#16111=DIRECTION('ref_axis',(0.,-0.707106781186547,0.707106781186547));
#16112=DIRECTION('',(-1.,0.,0.));
#16113=DIRECTION('center_axis',(-1.,0.,0.));
#16114=DIRECTION('ref_axis',(0.,-0.707106781186547,0.707106781186547));
#16115=DIRECTION('center_axis',(1.,0.,0.));
#16116=DIRECTION('ref_axis',(0.,-0.707106781186547,0.707106781186547));
#16117=DIRECTION('center_axis',(-1.,0.,0.));
#16118=DIRECTION('ref_axis',(0.,-0.707106781186547,0.707106781186547));
#16119=DIRECTION('center_axis',(1.,0.,0.));
#16120=DIRECTION('ref_axis',(0.,1.,0.));
#16121=DIRECTION('center_axis',(1.,1.40500107149015E-14,5.65401519314285E-15));
#16122=DIRECTION('ref_axis',(-8.92539775295977E-15,0.848328765343848,-0.529469834731104));
#16123=DIRECTION('center_axis',(-1.,0.,0.));
#16124=DIRECTION('ref_axis',(0.,1.,0.));
#16125=DIRECTION('',(-0.250380004054441,-0.684583761701115,-0.684583761701115));
#16126=DIRECTION('',(-0.250380004054442,0.684583761701115,0.684583761701115));
#16127=DIRECTION('',(-1.,0.,0.));
#16128=DIRECTION('center_axis',(1.,0.,0.));
#16129=DIRECTION('ref_axis',(0.,1.,0.));
#16130=DIRECTION('center_axis',(-1.,-4.36462899777869E-14,-5.90366440881238E-14));
#16131=DIRECTION('ref_axis',(2.59961128384679E-14,0.541519248253379,-0.840688351157012));
#16132=DIRECTION('center_axis',(-1.,0.,0.));
#16133=DIRECTION('ref_axis',(0.,1.,0.));
#16134=DIRECTION('',(-1.,0.,0.));
#16135=DIRECTION('',(-0.250380004054442,0.684583761701115,0.684583761701115));
#16136=DIRECTION('',(-0.250380004054441,-0.684583761701115,-0.684583761701115));
#16137=DIRECTION('center_axis',(-1.,0.,0.));
#16138=DIRECTION('ref_axis',(0.,1.,0.));
#16139=DIRECTION('center_axis',(-1.,0.,0.));
#16140=DIRECTION('ref_axis',(0.,1.,0.));
#16141=DIRECTION('',(1.,0.,0.));
#16142=DIRECTION('center_axis',(-1.,0.,0.));
#16143=DIRECTION('ref_axis',(0.,1.,0.));
#16144=DIRECTION('',(1.,0.,0.));
#16145=DIRECTION('center_axis',(1.,0.,0.));
#16146=DIRECTION('ref_axis',(0.,1.,0.));
#16147=DIRECTION('center_axis',(1.,0.,0.));
#16148=DIRECTION('ref_axis',(0.,-0.707106781186547,0.707106781186548));
#16149=DIRECTION('',(-0.250380004054441,0.684583761701115,0.684583761701115));
#16150=DIRECTION('',(-0.250380004054441,-0.684583761701115,-0.684583761701115));
#16151=DIRECTION('',(-0.250380004054441,0.684583761701115,0.684583761701115));
#16152=DIRECTION('',(-1.,0.,0.));
#16153=DIRECTION('',(-0.250380004054441,-0.684583761701115,-0.684583761701115));
#16154=DIRECTION('',(-0.250380004054442,0.684583761701115,0.684583761701115));
#16155=DIRECTION('',(-0.250380004054441,-0.684583761701115,-0.684583761701115));
#16156=DIRECTION('',(-0.250380004054441,0.684583761701115,0.684583761701115));
#16157=DIRECTION('',(-1.,0.,0.));
#16158=DIRECTION('',(-1.,0.,0.));
#16159=DIRECTION('',(-0.250380004054441,-0.684583761701115,-0.684583761701115));
#16160=DIRECTION('',(-0.250380004054442,0.684583761701115,0.684583761701115));
#16161=DIRECTION('',(-0.250380004054441,-0.684583761701115,-0.684583761701115));
#16162=DIRECTION('',(-0.250380004054441,0.684583761701115,0.684583761701115));
#16163=DIRECTION('',(-1.,0.,0.));
#16164=DIRECTION('',(-1.,0.,0.));
#16165=DIRECTION('',(-0.250380004054441,-0.684583761701115,-0.684583761701115));
#16166=DIRECTION('',(-0.250380004054442,0.684583761701115,0.684583761701115));
#16167=DIRECTION('',(-0.250380004054441,-0.684583761701115,-0.684583761701115));
#16168=DIRECTION('',(-0.250380004054441,0.684583761701115,0.684583761701115));
#16169=DIRECTION('',(-1.,0.,0.));
#16170=DIRECTION('',(-1.,0.,0.));
#16171=DIRECTION('',(-0.250380004054441,-0.684583761701115,-0.684583761701115));
#16172=DIRECTION('',(-0.250380004054442,0.684583761701115,0.684583761701115));
#16173=DIRECTION('',(-0.250380004054441,-0.684583761701115,-0.684583761701115));
#16174=DIRECTION('',(-0.250380004054441,0.684583761701115,0.684583761701115));
#16175=DIRECTION('',(-1.,0.,0.));
#16176=DIRECTION('',(-1.,0.,0.));
#16177=DIRECTION('',(-0.250380004054441,-0.684583761701115,-0.684583761701115));
#16178=DIRECTION('center_axis',(1.,0.,0.));
#16179=DIRECTION('ref_axis',(0.,-0.707106781186547,0.707106781186548));
#81959=CARTESIAN_POINT('',(0.,0.,0.));
#81960=CARTESIAN_POINT('Origin',(-31.4159265358979,26.,7.7715611723761E-15));
#81961=CARTESIAN_POINT('',(-13.2129142961191,30.2426811775992,-4.2426001962529));
#81962=CARTESIAN_POINT('',(-15.0614191220869,30.2426782484473,-4.24260312545867));
#81963=CARTESIAN_POINT('',(-31.4159265358979,30.2426406871193,-4.24264068711928));
#81964=CARTESIAN_POINT('',(-14.7837106730077,21.7573593180495,-4.24264068195052));
#81965=CARTESIAN_POINT('Ctrl Pts',(-13.2129142961191,30.2426811775992,-4.2426001962529));
#81966=CARTESIAN_POINT('Ctrl Pts',(-13.2410017129647,30.1234962961936,-4.36178735262007));
#81967=CARTESIAN_POINT('Ctrl Pts',(-13.2690891298103,29.999287665009,-4.47594744906339));
#81968=CARTESIAN_POINT('Ctrl Pts',(-13.2971765466559,29.8705004317943,-4.5846729880636));
#81969=CARTESIAN_POINT('Ctrl Pts',(-13.3252684134104,29.741692794729,-4.6934157525263));
#81970=CARTESIAN_POINT('Ctrl Pts',(-13.3533602801649,29.6083053406003,-4.79672204033205));
#81971=CARTESIAN_POINT('Ctrl Pts',(-13.3814521469194,29.4708168269235,-4.89422420348155));
#81972=CARTESIAN_POINT('Ctrl Pts',(-13.4000726886277,29.3796833103903,-4.95885298416863));
#81973=CARTESIAN_POINT('Ctrl Pts',(-13.4186932303359,29.286748621905,-5.02093247673682));
#81974=CARTESIAN_POINT('Ctrl Pts',(-13.4373137720442,29.1921594803238,-5.08036591715385));
#81975=CARTESIAN_POINT('Ctrl Pts',(-13.4652952223468,29.0500185369615,-5.16967770439425));
#81976=CARTESIAN_POINT('Ctrl Pts',(-13.4932766726495,28.9041139043336,-5.2530287541782));
#81977=CARTESIAN_POINT('Ctrl Pts',(-13.5212581229522,28.7549640208624,-5.33011943991441));
#81978=CARTESIAN_POINT('Ctrl Pts',(-13.5492367727318,28.6058290650555,-5.40720241003029));
#81979=CARTESIAN_POINT('Ctrl Pts',(-13.5772154225113,28.453449784519,-5.47802612351747));
#81980=CARTESIAN_POINT('Ctrl Pts',(-13.6051940722909,28.2983686959519,-5.54233717284218));
#81981=CARTESIAN_POINT('Ctrl Pts',(-13.6331753283905,28.1432731609781,-5.60665421299133));
#81982=CARTESIAN_POINT('Ctrl Pts',(-13.6611565844901,27.9854756029791,-5.66445725473928));
#81983=CARTESIAN_POINT('Ctrl Pts',(-13.6891378405898,27.8255386914581,-5.71554096179788));
#81984=CARTESIAN_POINT('Ctrl Pts',(-13.7171188027312,27.6656034601607,-5.76662413219454));
#81985=CARTESIAN_POINT('Ctrl Pts',(-13.7450997648726,27.5035292189573,-5.81098801655115));
#81986=CARTESIAN_POINT('Ctrl Pts',(-13.773080727014,27.3398942132321,-5.84847702375132));
#81987=CARTESIAN_POINT('Ctrl Pts',(-13.8010671071371,27.176227522697,-5.88597328998547));
#81988=CARTESIAN_POINT('Ctrl Pts',(-13.8290534872602,27.0109997688288,-5.91659195041649));
#81989=CARTESIAN_POINT('Ctrl Pts',(-13.8570398673834,26.8448005976496,-5.94022827425098));
#81990=CARTESIAN_POINT('Ctrl Pts',(-13.8667308191079,26.7872501699964,-5.94841291521625));
#81991=CARTESIAN_POINT('Ctrl Pts',(-13.8764217708324,26.7295833399769,-5.95576078735063));
#81992=CARTESIAN_POINT('Ctrl Pts',(-13.8861127225569,26.6718247952912,-5.96226898457557));
#81993=CARTESIAN_POINT('Ctrl Pts',(-13.9139899859855,26.5056749463158,-5.98099064717824));
#81994=CARTESIAN_POINT('Ctrl Pts',(-13.9418672494142,26.338713434746,-5.99276609931421));
#81995=CARTESIAN_POINT('Ctrl Pts',(-13.9697445128428,26.1715325455289,-5.99754754760846));
#81996=CARTESIAN_POINT('Ctrl Pts',(-13.9976163987277,26.0043839056231,-6.00232807355797));
#81997=CARTESIAN_POINT('Ctrl Pts',(-14.0254882846126,25.8370162900367,-6.00011727873267));
#81998=CARTESIAN_POINT('Ctrl Pts',(-14.0533601704975,25.6700239306005,-5.99091944476168));
#81999=CARTESIAN_POINT('Ctrl Pts',(-14.0812318269964,25.5030329455137,-5.98172168648899));
#82000=CARTESIAN_POINT('Ctrl Pts',(-14.1091034834953,25.336417527901,-5.96553701791644));
#82001=CARTESIAN_POINT('Ctrl Pts',(-14.1369751399941,25.1707694209928,-5.94242178298034));
#82002=CARTESIAN_POINT('Ctrl Pts',(-14.1648451281333,25.0051312295563,-5.91930793169096));
#82003=CARTESIAN_POINT('Ctrl Pts',(-14.1927151162726,24.8404605476793,-5.88926438829303));
#82004=CARTESIAN_POINT('Ctrl Pts',(-14.2205851044118,24.6773417948699,-5.85239910399162));
#82005=CARTESIAN_POINT('Ctrl Pts',(-14.2484593155124,24.5141983257171,-5.815528233729));
#82006=CARTESIAN_POINT('Ctrl Pts',(-14.276333526613,24.3526075654144,-5.77183362777214));
#82007=CARTESIAN_POINT('Ctrl Pts',(-14.3042077377136,24.1931422948714,-5.7214740437598));
#82008=CARTESIAN_POINT('Ctrl Pts',(-14.3144423828323,24.1345910251376,-5.70298338697199));
#82009=CARTESIAN_POINT('Ctrl Pts',(-14.324677027951,24.0763261658875,-5.68359467421659));
#82010=CARTESIAN_POINT('Ctrl Pts',(-14.3349116730697,24.0183755413334,-5.66331744693994));
#82011=CARTESIAN_POINT('Ctrl Pts',(-14.3630440790537,23.8590841855444,-5.60758056663204));
#82012=CARTESIAN_POINT('Ctrl Pts',(-14.3911764850377,23.7021323444495,-5.54511432266296));
#82013=CARTESIAN_POINT('Ctrl Pts',(-14.4193088910216,23.5480833323248,-5.47613957590351));
#82014=CARTESIAN_POINT('Ctrl Pts',(-14.4474378260405,23.3940533267062,-5.40717333922098));
#82015=CARTESIAN_POINT('Ctrl Pts',(-14.4755667610593,23.2429257136142,-5.33170032765871));
#82016=CARTESIAN_POINT('Ctrl Pts',(-14.5036956960782,23.0952427019562,-5.24998905136581));
#82017=CARTESIAN_POINT('Ctrl Pts',(-14.5318247858119,22.9475588780117,-5.16827732564439));
#82018=CARTESIAN_POINT('Ctrl Pts',(-14.5599538755456,22.8033199617192,-5.08032741225067));
#82019=CARTESIAN_POINT('Ctrl Pts',(-14.5880829652792,22.6630431588223,-4.98645355339013));
#82020=CARTESIAN_POINT('Ctrl Pts',(-14.6162099061363,22.5227770721466,-4.8925868658724));
#82021=CARTESIAN_POINT('Ctrl Pts',(-14.6443368469933,22.3864727472703,-4.79279730773824));
#82022=CARTESIAN_POINT('Ctrl Pts',(-14.6724637878503,22.254618346355,-4.68744240162367));
#82023=CARTESIAN_POINT('Ctrl Pts',(-14.7005922972612,22.1227565923209,-4.58208162018649));
#82024=CARTESIAN_POINT('Ctrl Pts',(-14.7287208066722,21.9953454967693,-4.47115506104073));
#82025=CARTESIAN_POINT('Ctrl Pts',(-14.7568493160831,21.8728406817017,-4.35506095954851));
#82026=CARTESIAN_POINT('Ctrl Pts',(-14.7658030852496,21.8338453755561,-4.31810628942479));
#82027=CARTESIAN_POINT('Ctrl Pts',(-14.7747568544161,21.7953469382496,-4.28062831248813));
#82028=CARTESIAN_POINT('Ctrl Pts',(-14.7837106235826,21.7573593128807,-4.24264068711927));
#82029=CARTESIAN_POINT('',(-17.341,27.1984341265848,5.87909479803116));
#82030=CARTESIAN_POINT('Ctrl Pts',(-14.783710716403,21.7573593128807,-4.24264068711927));
#82031=CARTESIAN_POINT('Ctrl Pts',(-14.811635381255,21.6388849936053,-4.12416636784387));
#82032=CARTESIAN_POINT('Ctrl Pts',(-14.839560046107,21.5253639382053,-4.0007141031509));
#82033=CARTESIAN_POINT('Ctrl Pts',(-14.8674847109591,21.4172023830087,-3.87272074925351));
#82034=CARTESIAN_POINT('Ctrl Pts',(-14.8954064382147,21.3090522061044,-3.74474085989806));
#82035=CARTESIAN_POINT('Ctrl Pts',(-14.9233281654703,21.2062606072779,-3.61222107567854));
#82036=CARTESIAN_POINT('Ctrl Pts',(-14.9512498927259,21.1091941405294,-3.47563203532363));
#82037=CARTESIAN_POINT('Ctrl Pts',(-14.9791745175235,21.0121176008308,-3.33902882061339));
#82038=CARTESIAN_POINT('Ctrl Pts',(-15.0070991423211,20.920767565003,-3.19835576152329));
#82039=CARTESIAN_POINT('Ctrl Pts',(-15.0350237671187,20.8354682159095,-3.05411385693448));
#82040=CARTESIAN_POINT('Ctrl Pts',(-15.0629484025602,20.7501688343031,-2.90987189736591));
#82041=CARTESIAN_POINT('Ctrl Pts',(-15.0908730380016,20.6709203017243,-2.76206136256888));
#82042=CARTESIAN_POINT('Ctrl Pts',(-15.1187976734431,20.598001758941,-2.61120949056086));
#82043=CARTESIAN_POINT('Ctrl Pts',(-15.1467285765726,20.5250668495812,-2.46032375983055));
#82044=CARTESIAN_POINT('Ctrl Pts',(-15.1746594797021,20.4584649048534,-2.30639561238042));
#82045=CARTESIAN_POINT('Ctrl Pts',(-15.2025903828316,20.3984280066064,-2.14997469818332));
#82046=CARTESIAN_POINT('Ctrl Pts',(-15.2125634775264,20.3769910459532,-2.09412256256521));
#82047=CARTESIAN_POINT('Ctrl Pts',(-15.2225365722211,20.3563906424098,-2.03795279762032));
#82048=CARTESIAN_POINT('Ctrl Pts',(-15.2325096669158,20.3366358561963,-1.98149099787989));
#82049=CARTESIAN_POINT('Ctrl Pts',(-15.2605103911617,20.2811717963202,-1.82296735668836));
#82050=CARTESIAN_POINT('Ctrl Pts',(-15.2885111154076,20.2323602403577,-1.66209219433237));
#82051=CARTESIAN_POINT('Ctrl Pts',(-15.3165118396535,20.1903798098822,-1.49943764344352));
#82052=CARTESIAN_POINT('Ctrl Pts',(-15.3445078536952,20.1484064412384,-1.33681045385234));
#82053=CARTESIAN_POINT('Ctrl Pts',(-15.3725038677369,20.1132619825743,-1.17240477502853));
#82054=CARTESIAN_POINT('Ctrl Pts',(-15.4004998817785,20.0850746867121,-1.00680610756265));
#82055=CARTESIAN_POINT('Ctrl Pts',(-15.4284955428502,20.0568877462315,-0.841209527942798));
#82056=CARTESIAN_POINT('Ctrl Pts',(-15.4564912039218,20.0356578486871,-0.674420296689421));
#82057=CARTESIAN_POINT('Ctrl Pts',(-15.4844868649934,20.0214619223184,-0.507032990752785));
#82058=CARTESIAN_POINT('Ctrl Pts',(-15.5124804766443,20.0072670351617,-0.339657938394383));
#82059=CARTESIAN_POINT('Ctrl Pts',(-15.5404740882952,20.0001051156435,-0.171685209709194));
#82060=CARTESIAN_POINT('Ctrl Pts',(-15.568467699946,20.0000011493054,-0.00371371286646238));
#82061=CARTESIAN_POINT('Ctrl Pts',(-15.5964640728379,19.9998971727122,0.164274352391451));
#82062=CARTESIAN_POINT('Ctrl Pts',(-15.6244604457297,20.0068525404938,0.332260873623216));
#82063=CARTESIAN_POINT('Ctrl Pts',(-15.6524568186215,20.0208401175802,0.499646975835977));
#82064=CARTESIAN_POINT('Ctrl Pts',(-15.6620740848906,20.0256451062057,0.557147164197301));
#82065=CARTESIAN_POINT('Ctrl Pts',(-15.6716913511596,20.0312794776917,0.614576523478925));
#82066=CARTESIAN_POINT('Ctrl Pts',(-15.6813086174286,20.0377407166053,0.67191088514314));
#82067=CARTESIAN_POINT('Ctrl Pts',(-15.7092296642895,20.0564991194029,0.838365192841986));
#82068=CARTESIAN_POINT('Ctrl Pts',(-15.7371507111504,20.0822345347245,1.00405202747329));
#82069=CARTESIAN_POINT('Ctrl Pts',(-15.7650717580113,20.1148590193363,1.16838163187921));
#82070=CARTESIAN_POINT('Ctrl Pts',(-15.7929896016934,20.147479761178,1.33269238394361));
#82071=CARTESIAN_POINT('Ctrl Pts',(-15.8209074453755,20.1869879332608,1.49564590721416));
#82072=CARTESIAN_POINT('Ctrl Pts',(-15.8488252890575,20.2332444334929,1.65666237844633));
#82073=CARTESIAN_POINT('Ctrl Pts',(-15.8767456944143,20.279505178111,1.81769362416544));
#82074=CARTESIAN_POINT('Ctrl Pts',(-15.904666099771,20.3325154035155,1.97678715868852));
#82075=CARTESIAN_POINT('Ctrl Pts',(-15.9325865051277,20.3920858482281,2.13337733801519));
#82076=CARTESIAN_POINT('Ctrl Pts',(-15.9605067427245,20.4516559350112,2.28996657646851));
#82077=CARTESIAN_POINT('Ctrl Pts',(-15.9884269803213,20.5177860473033,2.44405219594104));
#82078=CARTESIAN_POINT('Ctrl Pts',(-16.016347217918,20.5902383170795,2.59508738465685));
#82079=CARTESIAN_POINT('Ctrl Pts',(-16.044273509623,20.6627062971045,2.74615532321488));
#82080=CARTESIAN_POINT('Ctrl Pts',(-16.072199801328,20.7414990361101,2.89417122539148));
#82081=CARTESIAN_POINT('Ctrl Pts',(-16.1001260930329,20.8263317951561,3.03861108175881));
#82082=CARTESIAN_POINT('Ctrl Pts',(-16.1101199180024,20.8566904175805,3.09030096090228));
#82083=CARTESIAN_POINT('Ctrl Pts',(-16.1201137429719,20.8878221425343,3.14153310276232));
#82084=CARTESIAN_POINT('Ctrl Pts',(-16.1301075679414,20.9197125236784,3.19228431658747));
#82085=CARTESIAN_POINT('Ctrl Pts',(-16.1580655556408,21.0089267020812,3.33426216952963));
#82086=CARTESIAN_POINT('Ctrl Pts',(-16.1860235433401,21.1041101501299,3.47251987290981));
#82087=CARTESIAN_POINT('Ctrl Pts',(-16.2139815310394,21.2049286144706,3.60656213140395));
#82088=CARTESIAN_POINT('Ctrl Pts',(-16.2419342515229,21.3057280848616,3.74057913666768));
#82089=CARTESIAN_POINT('Ctrl Pts',(-16.2698869720064,21.412160264276,3.8703820310855));
#82090=CARTESIAN_POINT('Ctrl Pts',(-16.29783969249,21.5238489995523,3.99550650371025));
#82091=CARTESIAN_POINT('Ctrl Pts',(-16.3257916397405,21.6355346452756,4.12062751512036));
#82092=CARTESIAN_POINT('Ctrl Pts',(-16.3537435869911,21.7524763497601,4.24107012682793));
#82093=CARTESIAN_POINT('Ctrl Pts',(-16.3816955342416,21.874258829291,4.35640445692514));
#82094=CARTESIAN_POINT('Ctrl Pts',(-16.4096453034429,21.996031819385,4.47172980003287));
#82095=CARTESIAN_POINT('Ctrl Pts',(-16.4375950726441,22.1226446022546,4.58194744159069));
#82096=CARTESIAN_POINT('Ctrl Pts',(-16.4655448418454,22.2536460936716,4.68666538260823));
#82097=CARTESIAN_POINT('Ctrl Pts',(-16.4934975117503,22.3846611807822,4.79139419154048));
#82098=CARTESIAN_POINT('Ctrl Pts',(-16.5214501816551,22.5200656411934,4.89062196341714));
#82099=CARTESIAN_POINT('Ctrl Pts',(-16.54940285156,22.6593759004737,4.98399745441991));
#82100=CARTESIAN_POINT('Ctrl Pts',(-16.5592374071914,22.7083892684126,5.01684964578496));
#82101=CARTESIAN_POINT('Ctrl Pts',(-16.5690719628228,22.7578858352419,5.04897780417467));
#82102=CARTESIAN_POINT('Ctrl Pts',(-16.5789065184543,22.8078436787338,5.08036790209136));
#82103=CARTESIAN_POINT('Ctrl Pts',(-16.6068879338741,22.9499844347187,5.1696794483162));
#82104=CARTESIAN_POINT('Ctrl Pts',(-16.634869349294,23.0958888484545,5.25303026571069));
#82105=CARTESIAN_POINT('Ctrl Pts',(-16.6628507647138,23.2450384808978,5.33012073299153));
#82106=CARTESIAN_POINT('Ctrl Pts',(-16.6908293844766,23.3941732116208,5.40720349807049));
#82107=CARTESIAN_POINT('Ctrl Pts',(-16.7188080042394,23.5465522360667,5.47802701828067));
#82108=CARTESIAN_POINT('Ctrl Pts',(-16.7467866240022,23.701633037362,5.54233789163512));
#82109=CARTESIAN_POINT('Ctrl Pts',(-16.7747678577677,23.8567283276367,5.60665477346327));
#82110=CARTESIAN_POINT('Ctrl Pts',(-16.8027490915333,24.0145256112291,5.66445767062608));
#82111=CARTESIAN_POINT('Ctrl Pts',(-16.8307303252988,24.1744622187945,5.7155412525317));
#82112=CARTESIAN_POINT('Ctrl Pts',(-16.8587112697084,24.3343971724438,5.76662430617822));
#82113=CARTESIAN_POINT('Ctrl Pts',(-16.8866922141179,24.4964711071497,5.81098809101212));
#82114=CARTESIAN_POINT('Ctrl Pts',(-16.9146731585274,24.6601057782571,5.84847702180149));
#82115=CARTESIAN_POINT('Ctrl Pts',(-16.942659527978,24.8237721754128,5.88597322107268));
#82116=CARTESIAN_POINT('Ctrl Pts',(-16.9706458974285,24.9889996085543,5.91659183419624));
#82117=CARTESIAN_POINT('Ctrl Pts',(-16.998632266879,25.1551984328592,5.94022813637292));
#82118=CARTESIAN_POINT('Ctrl Pts',(-17.0083233342417,25.2127494490705,5.94841287062382));
#82119=CARTESIAN_POINT('Ctrl Pts',(-17.0180144016044,25.270416867388,5.95576081851139));
#82120=CARTESIAN_POINT('Ctrl Pts',(-17.0277054689671,25.3281759992757,5.96226907410684));
#82121=CARTESIAN_POINT('Ctrl Pts',(-17.0556148056643,25.4945167127237,5.98101222075169));
#82122=CARTESIAN_POINT('Ctrl Pts',(-17.0835241423614,25.6616705311091,5.99279315081194));
#82123=CARTESIAN_POINT('Ctrl Pts',(-17.1114334790586,25.8290438172005,5.9975640041239));
#82124=CARTESIAN_POINT('Ctrl Pts',(-17.1393368213947,25.9963811548955,6.00233383275307));
#82125=CARTESIAN_POINT('Ctrl Pts',(-17.1672401637309,26.1639375501269,6.0000965807107));
#82126=CARTESIAN_POINT('Ctrl Pts',(-17.195143506067,26.3311174488523,5.99085646924258));
#82127=CARTESIAN_POINT('Ctrl Pts',(-17.2230459518635,26.498291976056,5.98161665466098));
#82128=CARTESIAN_POINT('Ctrl Pts',(-17.25094839766,26.6650897149014,5.96537444428861));
#82129=CARTESIAN_POINT('Ctrl Pts',(-17.2788508434566,26.8309176112471,5.94218612324787));
#82130=CARTESIAN_POINT('Ctrl Pts',(-17.299567228971,26.9540378084802,5.92496977592058));
#82131=CARTESIAN_POINT('Ctrl Pts',(-17.3202836144855,27.0766234122808,5.90392551126519));
#82132=CARTESIAN_POINT('Ctrl Pts',(-17.341,27.1984341265848,5.87909479803116));
#82133=CARTESIAN_POINT('',(-17.341,20.0176003675788,-0.459232662172854));
#82134=CARTESIAN_POINT('Origin',(-17.341,26.,7.7715611723761E-15));
#82135=CARTESIAN_POINT('',(-16.6322154976385,21.7573593077119,-4.24264069228803));
#82136=CARTESIAN_POINT('Ctrl Pts',(-17.341,20.0176003675788,-0.459232662172852));
#82137=CARTESIAN_POINT('Ctrl Pts',(-17.2225531007737,20.0719950524366,-1.16782934856558));
#82138=CARTESIAN_POINT('Ctrl Pts',(-17.105980663342,20.2518558191926,-1.86116408950255));
#82139=CARTESIAN_POINT('Ctrl Pts',(-16.8692219591851,20.8456854082936,-3.15245663059683));
#82140=CARTESIAN_POINT('Ctrl Pts',(-16.7506405280734,21.2549246444944,-3.74020601873292));
#82141=CARTESIAN_POINT('Ctrl Pts',(-16.6322155410337,21.7573593128806,-4.24264068711921));
#82142=CARTESIAN_POINT('Ctrl Pts',(-16.6322154482133,21.7573593128807,-4.24264068711927));
#82143=CARTESIAN_POINT('Ctrl Pts',(-16.6040873150048,21.876696875284,-4.36197824952258));
#82144=CARTESIAN_POINT('Ctrl Pts',(-16.5759591817962,22.001078300101,-4.47628330412854));
#82145=CARTESIAN_POINT('Ctrl Pts',(-16.5478310485877,22.1300590992214,-4.58514530025829));
#82146=CARTESIAN_POINT('Ctrl Pts',(-16.5197046961868,22.2590317324958,-4.69400040427467));
#82147=CARTESIAN_POINT('Ctrl Pts',(-16.491578343786,22.3926029250832,-4.79741294130875));
#82148=CARTESIAN_POINT('Ctrl Pts',(-16.4634519913852,22.5302945345852,-4.89501215353657));
#82149=CARTESIAN_POINT('Ctrl Pts',(-16.4353229896715,22.6679991137089,-4.99262055895245));
#82150=CARTESIAN_POINT('Ctrl Pts',(-16.4071939879578,22.8098246372677,-5.08441436719853));
#82151=CARTESIAN_POINT('Ctrl Pts',(-16.3790649862441,22.9552626926979,-5.17006525389408));
#82152=CARTESIAN_POINT('Ctrl Pts',(-16.3509366819145,23.1006971423768,-5.25571401710279));
#82153=CARTESIAN_POINT('Ctrl Pts',(-16.3228083775849,23.2497436806413,-5.33522001016744));
#82154=CARTESIAN_POINT('Ctrl Pts',(-16.2946800732553,23.401867650476,-5.4082999449325));
#82155=CARTESIAN_POINT('Ctrl Pts',(-16.2665481067811,23.5540114259828,-5.48138939428771));
#82156=CARTESIAN_POINT('Ctrl Pts',(-16.2384161403069,23.7092331581346,-5.5480509819099));
#82157=CARTESIAN_POINT('Ctrl Pts',(-16.2102841738328,23.8669757466507,-5.60804846043824));
#82158=CARTESIAN_POINT('Ctrl Pts',(-16.2013282817887,23.917193551183,-5.62714882944768));
#82159=CARTESIAN_POINT('Ctrl Pts',(-16.1923723897446,23.9676666892194,-5.64557416629127));
#82160=CARTESIAN_POINT('Ctrl Pts',(-16.1834164977005,24.0183767844616,-5.66331788191683));
#82161=CARTESIAN_POINT('Ctrl Pts',(-16.1555420242995,24.1762077625514,-5.71854372952689));
#82162=CARTESIAN_POINT('Ctrl Pts',(-16.1276675508985,24.33637074922,-5.76717526848675));
#82163=CARTESIAN_POINT('Ctrl Pts',(-16.0997930774975,24.4982984770211,-5.80903542215768));
#82164=CARTESIAN_POINT('Ctrl Pts',(-16.0719226239925,24.660202852538,-5.85088953899838));
#82165=CARTESIAN_POINT('Ctrl Pts',(-16.0440521704875,24.8238711537045,-5.88597413996263));
#82166=CARTESIAN_POINT('Ctrl Pts',(-16.0161817169824,24.9887227670212,-5.9141625238117));
#82167=CARTESIAN_POINT('Ctrl Pts',(-15.988309486411,25.1535848915505,-5.94235270499893));
#82168=CARTESIAN_POINT('Ctrl Pts',(-15.9604372558396,25.3196301662181,-5.96364573398776));
#82169=CARTESIAN_POINT('Ctrl Pts',(-15.9325650252682,25.4862689201503,-5.97796624092144));
#82170=CARTESIAN_POINT('Ctrl Pts',(-15.9046933029176,25.6529046356006,-5.99228648673578));
#82171=CARTESIAN_POINT('Ctrl Pts',(-15.8768215805669,25.8201334918203,-5.999634440016));
#82172=CARTESIAN_POINT('Ctrl Pts',(-15.8489498582162,25.9873616309338,-5.99998668928751));
#82173=CARTESIAN_POINT('Ctrl Pts',(-15.821072225014,26.154625234691,-6.00033901326173));
#82174=CARTESIAN_POINT('Ctrl Pts',(-15.7931945918118,26.3218878031738,-5.99369266936041));
#82175=CARTESIAN_POINT('Ctrl Pts',(-15.7653169586096,26.4885556433562,-5.98007636935723));
#82176=CARTESIAN_POINT('Ctrl Pts',(-15.7550838214689,26.5497349713554,-5.97507818804572));
#82177=CARTESIAN_POINT('Ctrl Pts',(-15.7448506843283,26.6108341930809,-5.96914136077459));
#82178=CARTESIAN_POINT('Ctrl Pts',(-15.7346175471877,26.6718240929007,-5.96226906372046));
#82179=CARTESIAN_POINT('Ctrl Pts',(-15.7066311888463,26.8386238892982,-5.94347418534225));
#82180=CARTESIAN_POINT('Ctrl Pts',(-15.6786448305049,27.0046583179452,-5.91767274678865));
#82181=CARTESIAN_POINT('Ctrl Pts',(-15.6506584721634,27.1693349785026,-5.88495163175113));
#82182=CARTESIAN_POINT('Ctrl Pts',(-15.6226770670896,27.3339824931617,-5.85223630797928));
#82183=CARTESIAN_POINT('Ctrl Pts',(-15.5946956620157,27.4972724128116,-5.81260381282124));
#82184=CARTESIAN_POINT('Ctrl Pts',(-15.5667142569418,27.6586221159657,-5.7661922163963));
#82185=CARTESIAN_POINT('Ctrl Pts',(-15.5387334249018,27.8199685148236,-5.71978157043898));
#82186=CARTESIAN_POINT('Ctrl Pts',(-15.5107525928619,27.9793744752583,-5.66659218393378));
#82187=CARTESIAN_POINT('Ctrl Pts',(-15.4827717608219,28.1362714456714,-5.60681231275037));
#82188=CARTESIAN_POINT('Ctrl Pts',(-15.4547930658108,28.2931564331184,-5.54703700723933));
#82189=CARTESIAN_POINT('Ctrl Pts',(-15.4268143707998,28.4475325216267,-5.48067233496891));
#82190=CARTESIAN_POINT('Ctrl Pts',(-15.3988356757887,28.5988497756167,-5.40795523685032));
#82191=CARTESIAN_POINT('Ctrl Pts',(-15.3708542344006,28.7501818828451,-5.33523100085181));
#82192=CARTESIAN_POINT('Ctrl Pts',(-15.3428727930126,28.8984542738177,-5.25615322852832));
#82193=CARTESIAN_POINT('Ctrl Pts',(-15.3148913516245,29.0431396447295,-5.17100581151051));
#82194=CARTESIAN_POINT('Ctrl Pts',(-15.3052004333079,29.0932490758935,-5.14151638486731));
#82195=CARTESIAN_POINT('Ctrl Pts',(-15.2955095149914,29.1429284743663,-5.11129932464418));
#82196=CARTESIAN_POINT('Ctrl Pts',(-15.2858185966749,29.1921566655501,-5.08036768576688));
#82197=CARTESIAN_POINT('Ctrl Pts',(-15.2577278232719,29.3348529424569,-4.99070707463563));
#82198=CARTESIAN_POINT('Ctrl Pts',(-15.229637049869,29.4737825802179,-4.89502244371932));
#82199=CARTESIAN_POINT('Ctrl Pts',(-15.201546276466,29.608446748013,-4.79365331107231));
#82200=CARTESIAN_POINT('Ctrl Pts',(-15.1734574449732,29.7431016064979,-4.69229118605549));
#82201=CARTESIAN_POINT('Ctrl Pts',(-15.1453686134805,29.8734913370775,-4.58524552703901));
#82202=CARTESIAN_POINT('Ctrl Pts',(-15.1172797819877,29.9991481915547,-4.47289768963977));
#82203=CARTESIAN_POINT('Ctrl Pts',(-15.0986595620208,30.0824467179217,-4.39842177398193));
#82204=CARTESIAN_POINT('Ctrl Pts',(-15.0800393420538,30.1636660601329,-4.32161671282728));
#82205=CARTESIAN_POINT('Ctrl Pts',(-15.0614191220869,30.2426782484473,-4.24260312545867));
#82206=CARTESIAN_POINT('Origin',(-31.4159265358979,26.,7.7715611723761E-15));
#82207=CARTESIAN_POINT('',(-6.9297288961107,30.2426857292706,-4.24259564448975));
#82208=CARTESIAN_POINT('',(-8.77823372208692,30.2426826788146,-4.24259869500835));
#82209=CARTESIAN_POINT('',(-31.4159265358979,30.2426406871193,-4.24264068711928));
#82210=CARTESIAN_POINT('',(-8.5005252730077,21.7573593180495,-4.24264068195053));
#82211=CARTESIAN_POINT('Ctrl Pts',(-6.92972889611913,30.2426857292348,-4.24259564452553));
#82212=CARTESIAN_POINT('Ctrl Pts',(-6.95781684444987,30.1234985386172,-4.36178536589192));
#82213=CARTESIAN_POINT('Ctrl Pts',(-6.98590479278062,29.9992874203363,-4.47594779443039));
#82214=CARTESIAN_POINT('Ctrl Pts',(-7.01399274111136,29.8704975466977,-4.58467542373584));
#82215=CARTESIAN_POINT('Ctrl Pts',(-7.0420851505798,29.7416872176896,-4.69342032197528));
#82216=CARTESIAN_POINT('Ctrl Pts',(-7.07017756004824,29.6082969145932,-4.79672849740392));
#82217=CARTESIAN_POINT('Ctrl Pts',(-7.09826996951668,29.4708054188974,-4.89423229364448));
#82218=CARTESIAN_POINT('Ctrl Pts',(-7.11688943702581,29.3796769437922,-4.95885717988492));
#82219=CARTESIAN_POINT('Ctrl Pts',(-7.13550890453494,29.2867475157265,-5.02093305892931));
#82220=CARTESIAN_POINT('Ctrl Pts',(-7.15412837204407,29.1921638262116,-5.08036318648836));
#82221=CARTESIAN_POINT('Ctrl Pts',(-7.18210991041342,29.0500224284525,-5.16967542883757));
#82222=CARTESIAN_POINT('Ctrl Pts',(-7.21009144878276,28.9041172855606,-5.25302690670604));
#82223=CARTESIAN_POINT('Ctrl Pts',(-7.23807298715211,28.7549668361744,-5.33011798477098));
#82224=CARTESIAN_POINT('Ctrl Pts',(-7.2660517174012,28.6058313549574,-5.40720132626995));
#82225=CARTESIAN_POINT('Ctrl Pts',(-7.29403044765029,28.4534514951217,-5.47802537878091));
#82226=CARTESIAN_POINT('Ctrl Pts',(-7.32200917789939,28.2983697742659,-5.54233672567274));
#82227=CARTESIAN_POINT('Ctrl Pts',(-7.34999050219416,28.1432736750211,-5.60665403518583));
#82228=CARTESIAN_POINT('Ctrl Pts',(-7.37797182648893,27.9854755021155,-5.66445731054565));
#82229=CARTESIAN_POINT('Ctrl Pts',(-7.40595315078371,27.8255379264614,-5.71554120613708));
#82230=CARTESIAN_POINT('Ctrl Pts',(-7.43393417369507,27.6656020734754,-5.76662455151013));
#82231=CARTESIAN_POINT('Ctrl Pts',(-7.46191519660644,27.5035271624844,-5.81098856932182));
#82232=CARTESIAN_POINT('Ctrl Pts',(-7.4898962195178,27.3398914411849,-5.84847765883048));
#82233=CARTESIAN_POINT('Ctrl Pts',(-7.51788264881145,27.1762241028402,-5.88597399183237));
#82234=CARTESIAN_POINT('Ctrl Pts',(-7.5458690781051,27.0109956566457,-5.91659267356233));
#82235=CARTESIAN_POINT('Ctrl Pts',(-7.57385550739876,26.8447957516834,-5.94022896342705));
#82236=CARTESIAN_POINT('Ctrl Pts',(-7.58354611245147,26.7872472297949,-5.94841328546352));
#82237=CARTESIAN_POINT('Ctrl Pts',(-7.59323671750418,26.7295823093205,-5.9557608948509));
#82238=CARTESIAN_POINT('Ctrl Pts',(-7.60292732255689,26.67182567535,-5.96226888541102));
#82239=CARTESIAN_POINT('Ctrl Pts',(-7.63080398612794,26.5056789543317,-5.98099022039282));
#82240=CARTESIAN_POINT('Ctrl Pts',(-7.65868064969899,26.338720625094,-5.99276560336772));
#82241=CARTESIAN_POINT('Ctrl Pts',(-7.68655731327004,26.1715429512646,-5.99754724999073));
#82242=CARTESIAN_POINT('Ctrl Pts',(-7.71442860956402,26.0043974652504,-6.00232797597192));
#82243=CARTESIAN_POINT('Ctrl Pts',(-7.74229990585801,25.8370330364648,-6.00011764348317));
#82244=CARTESIAN_POINT('Ctrl Pts',(-7.77017120215199,25.6700438745741,-5.99092054322988));
#82245=CARTESIAN_POINT('Ctrl Pts',(-7.79804228889752,25.5030559681801,-5.98172351212437));
#82246=CARTESIAN_POINT('Ctrl Pts',(-7.82591337564304,25.3364436405639,-5.96553983216607));
#82247=CARTESIAN_POINT('Ctrl Pts',(-7.85378446238856,25.1707986121721,-5.94242585636743));
#82248=CARTESIAN_POINT('Ctrl Pts',(-7.88165389348992,25.0051634236989,-5.91931325362322));
#82249=CARTESIAN_POINT('Ctrl Pts',(-7.90952332459129,24.8404957342096,-5.88927122297676));
#82250=CARTESIAN_POINT('Ctrl Pts',(-7.93739275569265,24.6773799389868,-5.85240772453572));
#82251=CARTESIAN_POINT('Ctrl Pts',(-7.96526643215482,24.5142392962743,-5.81553861066426));
#82252=CARTESIAN_POINT('Ctrl Pts',(-7.99314010861698,24.3526513301256,-5.7718460233064));
#82253=CARTESIAN_POINT('Ctrl Pts',(-8.02101378507914,24.1931887960309,-5.72148872874986));
#82254=CARTESIAN_POINT('Ctrl Pts',(-8.031251281076,24.1346210984163,-5.7029934074694));
#82255=CARTESIAN_POINT('Ctrl Pts',(-8.04148877707287,24.0763399740661,-5.68359953185717));
#82256=CARTESIAN_POINT('Ctrl Pts',(-8.05172627306973,24.0183732706507,-5.66331665241563));
#82257=CARTESIAN_POINT('Ctrl Pts',(-8.07985938912929,23.8590780684571,-5.60757835454219));
#82258=CARTESIAN_POINT('Ctrl Pts',(-8.10799250518886,23.7021225204538,-5.54511037539292));
#82259=CARTESIAN_POINT('Ctrl Pts',(-8.13612562124842,23.5480699659983,-5.47613359117183));
#82260=CARTESIAN_POINT('Ctrl Pts',(-8.16425526800264,23.3940364089177,-5.40716531299486));
#82261=CARTESIAN_POINT('Ctrl Pts',(-8.19238491475685,23.2429054092286,-5.33168995691243));
#82262=CARTESIAN_POINT('Ctrl Pts',(-8.22051456151107,23.0952192005546,-5.24997604824758));
#82263=CARTESIAN_POINT('Ctrl Pts',(-8.24864435841876,22.9475322035451,-5.16826170340138));
#82264=CARTESIAN_POINT('Ctrl Pts',(-8.27677415532646,22.8032903026227,-5.08030888503684));
#82265=CARTESIAN_POINT('Ctrl Pts',(-8.30490395223415,22.6630107280007,-4.98643185038779));
#82266=CARTESIAN_POINT('Ctrl Pts',(-8.33303159546407,22.5227418934848,-4.89256200316648));
#82267=CARTESIAN_POINT('Ctrl Pts',(-8.36115923869398,22.386435032278,-4.79276901652899));
#82268=CARTESIAN_POINT('Ctrl Pts',(-8.3892868819239,22.2545783311889,-4.68741042824289));
#82269=CARTESIAN_POINT('Ctrl Pts',(-8.41741608128806,22.1227143352573,-4.58204601109636));
#82270=CARTESIAN_POINT('Ctrl Pts',(-8.44554528065223,21.9953012300267,-4.47111556744834));
#82271=CARTESIAN_POINT('Ctrl Pts',(-8.4736744800164,21.872794662332,-4.35501734792463));
#82272=CARTESIAN_POINT('Ctrl Pts',(-8.48262472787178,21.8338150905857,-4.31807680699938));
#82273=CARTESIAN_POINT('Ctrl Pts',(-8.49157497572716,21.7953319985918,-4.28061337283033));
#82274=CARTESIAN_POINT('Ctrl Pts',(-8.50052522358255,21.7573593128807,-4.24264068711927));
#82275=CARTESIAN_POINT('',(-11.6421179699928,30.2426406871193,4.24264068711929));
#82276=CARTESIAN_POINT('Ctrl Pts',(-8.50052531640296,21.7573593128807,-4.24264068711927));
#82277=CARTESIAN_POINT('Ctrl Pts',(-8.52845069909252,21.6388819480786,-4.12416332231719));
#82278=CARTESIAN_POINT('Ctrl Pts',(-8.55637608178207,21.5253581562297,-4.00070781090067));
#82279=CARTESIAN_POINT('Ctrl Pts',(-8.58430146447163,21.4171941806491,-3.87271104294179));
#82280=CARTESIAN_POINT('Ctrl Pts',(-8.61222392419931,21.3090415266385,-3.74472767245994));
#82281=CARTESIAN_POINT('Ctrl Pts',(-8.64014638392699,21.2062477723132,-3.61220423501525));
#82282=CARTESIAN_POINT('Ctrl Pts',(-8.66806884365467,21.1091794775264,-3.47561140189052));
#82283=CARTESIAN_POINT('Ctrl Pts',(-8.69599421623101,21.0121010566528,-3.33900431951072));
#82284=CARTESIAN_POINT('Ctrl Pts',(-8.72391958880735,20.9207494733936,-3.19832724871925));
#82285=CARTESIAN_POINT('Ctrl Pts',(-8.75184496138369,20.8354489157695,-3.05408122000282));
#82286=CARTESIAN_POINT('Ctrl Pts',(-8.77977035175856,20.7501483037783,-2.90983509934969));
#82287=CARTESIAN_POINT('Ctrl Pts',(-8.80769574213342,20.6708988827886,-2.76202028919063));
#82288=CARTESIAN_POINT('Ctrl Pts',(-8.83562113250829,20.5979797981118,-2.61116405811506));
#82289=CARTESIAN_POINT('Ctrl Pts',(-8.86355279570316,20.5250443337788,-2.46027394053079));
#82290=CARTESIAN_POINT('Ctrl Pts',(-8.89148445889802,20.4584421829795,-2.30634132137571));
#82291=CARTESIAN_POINT('Ctrl Pts',(-8.91941612209289,20.3984054317556,-2.14991588045076));
#82292=CARTESIAN_POINT('Ctrl Pts',(-8.92938550370053,20.3769770878987,-2.09408444274354));
#82293=CARTESIAN_POINT('Ctrl Pts',(-8.93935488530816,20.3563846777811,-2.03793562245308));
#82294=CARTESIAN_POINT('Ctrl Pts',(-8.9493242669158,20.3366372511112,-1.981494984727));
#82295=CARTESIAN_POINT('Ctrl Pts',(-8.97732492365711,20.2811733379547,-1.82297212087967));
#82296=CARTESIAN_POINT('Ctrl Pts',(-9.00532558039843,20.2323618582529,-1.66209773342208));
#82297=CARTESIAN_POINT('Ctrl Pts',(-9.03332623713976,20.190381437133,-1.4994439482659));
#82298=CARTESIAN_POINT('Ctrl Pts',(-9.0613221792703,20.1484080844668,-1.33681754994193));
#82299=CARTESIAN_POINT('Ctrl Pts',(-9.08931812140085,20.1132635727499,-1.17241265378827));
#82300=CARTESIAN_POINT('Ctrl Pts',(-9.1173140635314,20.0850761584985,-1.00681475418157));
#82301=CARTESIAN_POINT('Ctrl Pts',(-9.14530964735303,20.0568891050067,-0.84121897399644));
#82302=CARTESIAN_POINT('Ctrl Pts',(-9.17330523117467,20.0356590264685,-0.674430527827274));
#82303=CARTESIAN_POINT('Ctrl Pts',(-9.2013008149963,20.0214628548888,-0.507043986776435));
#82304=CARTESIAN_POINT('Ctrl Pts',(-9.22929434665013,20.007267723935,-0.339669715706182));
#82305=CARTESIAN_POINT('Ctrl Pts',(-9.25728787830396,20.000105495034,-0.171697748236844));
#82306=CARTESIAN_POINT('Ctrl Pts',(-9.28528140995779,20.0000011575362,-0.00372698713702113));
#82307=CARTESIAN_POINT('Ctrl Pts',(-9.31327769979149,19.9998968097581,0.164260323985088));
#82308=CARTESIAN_POINT('Ctrl Pts',(-9.34127398962519,20.0068517430295,0.332246116553286));
#82309=CARTESIAN_POINT('Ctrl Pts',(-9.3692702794589,20.0208388260907,0.499631520638411));
#82310=CARTESIAN_POINT('Ctrl Pts',(-9.37888792544881,20.0256438489745,0.557133910059677));
#82311=CARTESIAN_POINT('Ctrl Pts',(-9.38850557143871,20.0312783181165,0.614565467986606));
#82312=CARTESIAN_POINT('Ctrl Pts',(-9.39812321742862,20.0377397179013,0.671902022997967));
#82313=CARTESIAN_POINT('Ctrl Pts',(-9.42604429401234,20.0564978670804,0.838356303515164));
#82314=CARTESIAN_POINT('Ctrl Pts',(-9.45396537059607,20.0822330307513,1.00404317010695));
#82315=CARTESIAN_POINT('Ctrl Pts',(-9.48188644717979,20.1148572786045,1.16837286377507));
#82316=CARTESIAN_POINT('Ctrl Pts',(-9.50980430841761,20.1474777695023,1.33268363350215));
#82317=CARTESIAN_POINT('Ctrl Pts',(-9.53772216965544,20.1869856995438,1.49563723290372));
#82318=CARTESIAN_POINT('Ctrl Pts',(-9.56564003089326,20.2332419793214,1.65665383557911));
#82319=CARTESIAN_POINT('Ctrl Pts',(-9.59356043576381,20.2795024735689,1.81768510868707));
#82320=CARTESIAN_POINT('Ctrl Pts',(-9.62148084063436,20.3325124614835,1.97677872842205));
#82321=CARTESIAN_POINT('Ctrl Pts',(-9.64940124550491,20.3920826940288,2.13336904669319));
#82322=CARTESIAN_POINT('Ctrl Pts',(-9.67732147215226,20.4516525463218,2.28995836540765));
#82323=CARTESIAN_POINT('Ctrl Pts',(-9.70524169879962,20.5177824445448,2.44404412074397));
#82324=CARTESIAN_POINT('Ctrl Pts',(-9.73316192544697,20.5902345326086,2.5950794954721));
#82325=CARTESIAN_POINT('Ctrl Pts',(-9.76108819095282,20.6627022913155,2.74614753760182));
#82326=CARTESIAN_POINT('Ctrl Pts',(-9.78901445645868,20.7414948344809,2.89416359684659));
#82327=CARTESIAN_POINT('Ctrl Pts',(-9.81694072196453,20.8263274346028,3.03860365728353));
#82328=CARTESIAN_POINT('Ctrl Pts',(-9.82693453729016,20.8566859993395,3.0902936080694));
#82329=CARTESIAN_POINT('Ctrl Pts',(-9.8369283526158,20.8878176712821,3.14152582759828));
#82330=CARTESIAN_POINT('Ctrl Pts',(-9.84692216794143,20.9197080045832,3.19227712476596));
#82331=CARTESIAN_POINT('Ctrl Pts',(-9.87487991362713,21.0089213629666,3.33425411885685));
#82332=CARTESIAN_POINT('Ctrl Pts',(-9.90283765931282,21.1041039105059,3.47251101870401));
#82333=CARTESIAN_POINT('Ctrl Pts',(-9.93079540499851,21.2049213976204,3.60655253628739));
#82334=CARTESIAN_POINT('Ctrl Pts',(-9.95874788641887,21.3057199014445,3.74056881470723));
#82335=CARTESIAN_POINT('Ctrl Pts',(-9.98670036783922,21.4121510387671,3.87037104399797));
#82336=CARTESIAN_POINT('Ctrl Pts',(-10.0146528492596,21.5238386602809,3.99549492063299));
#82337=CARTESIAN_POINT('Ctrl Pts',(-10.0426045636081,21.6355232168635,4.12061536361926));
#82338=CARTESIAN_POINT('Ctrl Pts',(-10.0705562779566,21.7524637628468,4.2410574739713));
#82339=CARTESIAN_POINT('Ctrl Pts',(-10.0985079923051,21.8742450184155,4.35639137726755));
#82340=CARTESIAN_POINT('Ctrl Pts',(-10.1264575326743,21.996016802296,4.47171631032632));
#82341=CARTESIAN_POINT('Ctrl Pts',(-10.1544070730436,22.1226283148942,4.58193361489443));
#82342=CARTESIAN_POINT('Ctrl Pts',(-10.1823566134128,22.2536284761326,4.68665129971874));
#82343=CARTESIAN_POINT('Ctrl Pts',(-10.2103090618765,22.384642267679,4.79137988021132));
#82344=CARTESIAN_POINT('Ctrl Pts',(-10.2382615103402,22.5200453749241,4.89060750154165));
#82345=CARTESIAN_POINT('Ctrl Pts',(-10.2662139588039,22.6593542278063,4.98398292781231));
#82346=CARTESIAN_POINT('Ctrl Pts',(-10.2760496786874,22.7083732915929,5.016839245855));
#82347=CARTESIAN_POINT('Ctrl Pts',(-10.2858853985708,22.7578756697644,5.04897135862553));
#82348=CARTESIAN_POINT('Ctrl Pts',(-10.2957211184543,22.8078394319699,5.08036523371242));
#82349=CARTESIAN_POINT('Ctrl Pts',(-10.323702586032,22.9499804657511,5.1696771202131));
#82350=CARTESIAN_POINT('Ctrl Pts',(-10.3516840536097,23.0958852012862,5.25302826428355));
#82351=CARTESIAN_POINT('Ctrl Pts',(-10.3796655211874,23.245035200224,5.33011903731945));
#82352=CARTESIAN_POINT('Ctrl Pts',(-10.4076441864509,23.3941702619481,5.40720208979644));
#82353=CARTESIAN_POINT('Ctrl Pts',(-10.4356228517144,23.5465496605457,5.47802587945846));
#82354=CARTESIAN_POINT('Ctrl Pts',(-10.4636015169779,23.7016308792268,5.54233699667174));
#82355=CARTESIAN_POINT('Ctrl Pts',(-10.4915827856967,23.8567265284392,5.60665409812732));
#82356=CARTESIAN_POINT('Ctrl Pts',(-10.5195640544154,24.0145242121799,5.66445719422693));
#82357=CARTESIAN_POINT('Ctrl Pts',(-10.5475453231341,24.1744612607334,5.71554094652789));
#82358=CARTESIAN_POINT('Ctrl Pts',(-10.5755262961688,24.3343966191982,5.766624159016));
#82359=CARTESIAN_POINT('Ctrl Pts',(-10.6035072692035,24.4964709985975,5.81098807718157));
#82360=CARTESIAN_POINT('Ctrl Pts',(-10.6314882422382,24.660106153123,5.84847710768379));
#82361=CARTESIAN_POINT('Ctrl Pts',(-10.6594746305795,24.8237729768308,5.88597339363759));
#82362=CARTESIAN_POINT('Ctrl Pts',(-10.6874610189208,24.9890008741831,5.91659206459093));
#82363=CARTESIAN_POINT('Ctrl Pts',(-10.7154474072621,25.1552001985585,5.94022838748516));
#82364=CARTESIAN_POINT('Ctrl Pts',(-10.7251382944971,25.2127502793841,5.94841297125584));
#82365=CARTESIAN_POINT('Ctrl Pts',(-10.7348291817321,25.2704167621195,5.95576079644968));
#82366=CARTESIAN_POINT('Ctrl Pts',(-10.7445200689671,25.3281749595449,5.96226895695066));
#82367=CARTESIAN_POINT('Ctrl Pts',(-10.7723971906407,25.4943240703769,5.98099054329845));
#82368=CARTESIAN_POINT('Ctrl Pts',(-10.8002743123142,25.6612848310749,5.99276598017385));
#82369=CARTESIAN_POINT('Ctrl Pts',(-10.8281514339878,25.8284649617233,5.99754747631426));
#82370=CARTESIAN_POINT('Ctrl Pts',(-10.856023180526,25.9956128574863,6.00232805050909));
#82371=CARTESIAN_POINT('Ctrl Pts',(-10.8838949270642,26.1629797212672,6.00011736581946));
#82372=CARTESIAN_POINT('Ctrl Pts',(-10.9117666736025,26.3299713264642,5.9909197059977));
#82373=CARTESIAN_POINT('Ctrl Pts',(-10.9396381954146,26.4969615852309,5.9817221203354));
#82374=CARTESIAN_POINT('Ctrl Pts',(-10.9675097172268,26.6635762739584,5.96553768605322));
#82375=CARTESIAN_POINT('Ctrl Pts',(-10.995381239039,26.82922365479,5.94242274921069));
#82376=CARTESIAN_POINT('Ctrl Pts',(-11.0232510954796,26.9948611379049,5.91930919352551));
#82377=CARTESIAN_POINT('Ctrl Pts',(-11.0511209519203,27.1595311140562,5.88926600805049));
#82378=CARTESIAN_POINT('Ctrl Pts',(-11.0789908083609,27.3226491694477,5.85240114607324));
#82379=CARTESIAN_POINT('Ctrl Pts',(-11.1068648930307,27.4857919720246,5.81553069120456));
#82380=CARTESIAN_POINT('Ctrl Pts',(-11.1347389777004,27.6473820734677,5.77183656247926));
#82381=CARTESIAN_POINT('Ctrl Pts',(-11.1626130623701,27.8068466988594,5.72147751955919));
#82382=CARTESIAN_POINT('Ctrl Pts',(-11.1728483814067,27.8654018526975,5.70298576003517));
#82383=CARTESIAN_POINT('Ctrl Pts',(-11.1830837004433,27.9236705575847,5.68359582672217));
#82384=CARTESIAN_POINT('Ctrl Pts',(-11.1933190194799,27.9816249837635,5.66331726320576));
#82385=CARTESIAN_POINT('Ctrl Pts',(-11.2214515954767,28.1409172630754,5.60758004317469));
#82386=CARTESIAN_POINT('Ctrl Pts',(-11.2495841714735,28.2978699939995,5.54511338331285));
#82387=CARTESIAN_POINT('Ctrl Pts',(-11.2777167474703,28.4519198562624,5.47613814822693));
#82388=CARTESIAN_POINT('Ctrl Pts',(-11.3058458529672,28.6059507145766,5.40717142208619));
#82389=CARTESIAN_POINT('Ctrl Pts',(-11.3339749584641,28.7570791405905,5.33169784842252));
#82390=CARTESIAN_POINT('Ctrl Pts',(-11.362104063961,28.9047629194926,5.2499859410803));
#82391=CARTESIAN_POINT('Ctrl Pts',(-11.390233323177,29.0524475054531,5.16827358720107));
#82392=CARTESIAN_POINT('Ctrl Pts',(-11.4183625823931,29.1966871383346,5.08032297713911));
#82393=CARTESIAN_POINT('Ctrl Pts',(-11.4464918416091,29.3369646065521,4.98644835675844));
#82394=CARTESIAN_POINT('Ctrl Pts',(-11.4746189508543,29.4772313531051,4.89258091138735));
#82395=CARTESIAN_POINT('Ctrl Pts',(-11.5027460600994,29.6135362869088,4.79279053100786));
#82396=CARTESIAN_POINT('Ctrl Pts',(-11.5308731693445,29.7453912399233,4.68743474193568));
#82397=CARTESIAN_POINT('Ctrl Pts',(-11.5590018442466,29.8772535324625,4.58207308837832));
#82398=CARTESIAN_POINT('Ctrl Pts',(-11.5871305191486,30.0046651106096,4.47114559753712));
#82399=CARTESIAN_POINT('Ctrl Pts',(-11.6152591940506,30.127170346444,4.3550505084825));
#82400=CARTESIAN_POINT('Ctrl Pts',(-11.6242121193646,30.1661618819794,4.31809922424115));
#82401=CARTESIAN_POINT('Ctrl Pts',(-11.6331650446787,30.2046566419131,4.2806247323255));
#82402=CARTESIAN_POINT('Ctrl Pts',(-11.6421179699928,30.2426406871193,4.24264068711928));
#82403=CARTESIAN_POINT('Ctrl Pts',(-11.6421179699928,30.2426406871193,4.24264068711928));
#82404=CARTESIAN_POINT('Ctrl Pts',(-11.6700431543099,30.3611172102982,4.12416416394038));
#82405=CARTESIAN_POINT('Ctrl Pts',(-11.6979683386269,30.4746402455888,4.00070955009656));
#82406=CARTESIAN_POINT('Ctrl Pts',(-11.725893522944,30.5828035516995,3.87271372638496));
#82407=CARTESIAN_POINT('Ctrl Pts',(-11.7538157803785,30.6909555210438,3.74473131811725));
#82408=CARTESIAN_POINT('Ctrl Pts',(-11.781738037813,30.7937486792756,3.61220889083677));
#82409=CARTESIAN_POINT('Ctrl Pts',(-11.8096602952475,30.8908164682605,3.47561710690225));
#82410=CARTESIAN_POINT('Ctrl Pts',(-11.8375854614852,30.9878943692896,3.33901109350855));
#82411=CARTESIAN_POINT('Ctrl Pts',(-11.865510627723,31.0792455246564,3.19833513191561));
#82412=CARTESIAN_POINT('Ctrl Pts',(-11.8934357939607,31.1645457478722,3.05409024394096));
#82413=CARTESIAN_POINT('Ctrl Pts',(-11.9213609761272,31.2498460197439,2.90984527368792));
#82414=CARTESIAN_POINT('Ctrl Pts',(-11.9492861582937,31.329095194901,2.76203164595643));
#82415=CARTESIAN_POINT('Ctrl Pts',(-11.9772113404601,31.4020141294016,2.61117662094029));
#82416=CARTESIAN_POINT('Ctrl Pts',(-12.0051427941856,31.4749494403542,2.46028771624566));
#82417=CARTESIAN_POINT('Ctrl Pts',(-12.0330742479111,31.5415515340173,2.30635633389469));
#82418=CARTESIAN_POINT('Ctrl Pts',(-12.0610057016366,31.6015883256266,2.1499321454883));
#82419=CARTESIAN_POINT('Ctrl Pts',(-12.0709761079263,31.6230190470833,2.09409499761674));
#82420=CARTESIAN_POINT('Ctrl Pts',(-12.0809465142159,31.6436136628225,2.03794039915355));
#82421=CARTESIAN_POINT('Ctrl Pts',(-12.0909169205055,31.6633631202419,1.98149392335291));
#82422=CARTESIAN_POINT('Ctrl Pts',(-12.1189176009114,31.7188270832263,1.82297082178452));
#82423=CARTESIAN_POINT('Ctrl Pts',(-12.1469182813172,31.7676385913327,1.66209619658588));
#82424=CARTESIAN_POINT('Ctrl Pts',(-12.1749189617231,31.8096190203628,1.49944217569028));
#82425=CARTESIAN_POINT('Ctrl Pts',(-12.2029149287158,31.8515923827395,1.33681553468645));
#82426=CARTESIAN_POINT('Ctrl Pts',(-12.2309108957085,31.8867368830954,1.17241039769987));
#82427=CARTESIAN_POINT('Ctrl Pts',(-12.2589068627012,31.9149242658821,1.00681226098963));
#82428=CARTESIAN_POINT('Ctrl Pts',(-12.2869024727919,31.9431112893265,0.841216235380474));
#82429=CARTESIAN_POINT('Ctrl Pts',(-12.3148980828826,31.9643413170165,0.674427547395076));
#82430=CARTESIAN_POINT('Ctrl Pts',(-12.3428936929732,31.9785374179344,0.507040769917742));
#82431=CARTESIAN_POINT('Ctrl Pts',(-12.3708872516044,31.9927324785918,0.339666258191626));
#82432=CARTESIAN_POINT('Ctrl Pts',(-12.3988808102356,31.9998946170303,0.171694055423287));
#82433=CARTESIAN_POINT('Ctrl Pts',(-12.4268743688668,31.9999988448982,0.00372306604439232));
#82434=CARTESIAN_POINT('Ctrl Pts',(-12.4548706864185,32.0001030830383,-0.16426447780736));
#82435=CARTESIAN_POINT('Ctrl Pts',(-12.4828670039702,31.9931480205866,-0.332250496085683));
#82436=CARTESIAN_POINT('Ctrl Pts',(-12.5108633215219,31.9791607898017,-0.499636117287159));
#82437=CARTESIAN_POINT('Ctrl Pts',(-12.5204808380207,31.9743557856222,-0.557137750157443));
#82438=CARTESIAN_POINT('Ctrl Pts',(-12.5300983545196,31.9687213569753,-0.614568552568057));
#82439=CARTESIAN_POINT('Ctrl Pts',(-12.5397158710184,31.9622600194022,-0.671904354084557));
#82440=CARTESIAN_POINT('Ctrl Pts',(-12.5676369379214,31.9435018047756,-0.838358630535872));
#82441=CARTESIAN_POINT('Ctrl Pts',(-12.5955580048243,31.9177665771291,-1.00404547747855));
#82442=CARTESIAN_POINT('Ctrl Pts',(-12.6234790717273,31.8851422701962,-1.16837513648239));
#82443=CARTESIAN_POINT('Ctrl Pts',(-12.6513969265305,31.8525217164338,-1.33268589064812));
#82444=CARTESIAN_POINT('Ctrl Pts',(-12.6793147813338,31.8130137268255,-1.49563945916178));
#82445=CARTESIAN_POINT('Ctrl Pts',(-12.707232636137,31.7667573941392,-1.65665601654091));
#82446=CARTESIAN_POINT('Ctrl Pts',(-12.7351530394038,31.720496838973,-1.81768727221378));
#82447=CARTESIAN_POINT('Ctrl Pts',(-12.7630734426706,31.6674867944667,-1.97678085943301));
#82448=CARTESIAN_POINT('Ctrl Pts',(-12.7909938459374,31.6079165129524,-2.13337113127463));
#82449=CARTESIAN_POINT('Ctrl Pts',(-12.8189140737873,31.5483466057032,-2.28996041929891));
#82450=CARTESIAN_POINT('Ctrl Pts',(-12.8468343016373,31.4822166588321,-2.44404612952963));
#82451=CARTESIAN_POINT('Ctrl Pts',(-12.8747545294872,31.4097645315886,-2.59508144626834));
#82452=CARTESIAN_POINT('Ctrl Pts',(-12.9026808002997,31.3372967230442,-2.74614945259596));
#82453=CARTESIAN_POINT('Ctrl Pts',(-12.9306070711122,31.2585041376586,-2.89416546225386));
#82454=CARTESIAN_POINT('Ctrl Pts',(-12.9585333419248,31.1736715059612,-3.0386054611294));
#82455=CARTESIAN_POINT('Ctrl Pts',(-12.9685271684603,31.1433129016411,-3.09029543804178));
#82456=CARTESIAN_POINT('Ctrl Pts',(-12.9785209949957,31.112181190035,-3.14152768131535));
#82457=CARTESIAN_POINT('Ctrl Pts',(-12.9885148215312,31.0802908171608,-3.19227899987956));
#82458=CARTESIAN_POINT('Ctrl Pts',(-13.0169030324834,30.9897038303564,-3.33644191209172));
#82459=CARTESIAN_POINT('Ctrl Pts',(-13.0452912434355,30.892967802122,-3.47676099978773));
#82460=CARTESIAN_POINT('Ctrl Pts',(-13.0736794543876,30.7904285700081,-3.61272668709525));
#82461=CARTESIAN_POINT('Ctrl Pts',(-13.1020615285156,30.6879115043224,-3.74866298200747));
#82462=CARTESIAN_POINT('Ctrl Pts',(-13.1304436026435,30.5795939149887,-3.88024752181972));
#82463=CARTESIAN_POINT('Ctrl Pts',(-13.1588256767714,30.4658634811698,-4.00700179280647));
#82464=CARTESIAN_POINT('Ctrl Pts',(-13.176855216554,30.3936169155458,-4.08752167169423));
#82465=CARTESIAN_POINT('Ctrl Pts',(-13.1948847563365,30.3191869158306,-4.16609299770538));
#82466=CARTESIAN_POINT('Ctrl Pts',(-13.2129142961191,30.2426811775992,-4.2426001962529));
#82467=CARTESIAN_POINT('',(-13.4906227946235,30.2426406871193,4.24264068711929));
#82468=CARTESIAN_POINT('Ctrl Pts',(-15.0614191220869,30.2426782484473,-4.24260312545867));
#82469=CARTESIAN_POINT('Ctrl Pts',(-15.0330386320433,30.3631067196343,-4.12217252186706));
#82470=CARTESIAN_POINT('Ctrl Pts',(-15.0046581419997,30.4783899337406,-3.99662567453541));
#82471=CARTESIAN_POINT('Ctrl Pts',(-14.976277651956,30.5881149555321,-3.86641968167225));
#82472=CARTESIAN_POINT('Ctrl Pts',(-14.9478886092434,30.6978730437644,-3.73617445027738));
#82473=CARTESIAN_POINT('Ctrl Pts',(-14.9194995665308,30.8020694046409,-3.60126749182685));
#82474=CARTESIAN_POINT('Ctrl Pts',(-14.8911105238182,30.9003311423157,-3.46218929229054));
#82475=CARTESIAN_POINT('Ctrl Pts',(-14.8730802312661,30.9627385963071,-3.37385871169863));
#82476=CARTESIAN_POINT('Ctrl Pts',(-14.8550499387141,31.0227530197161,-3.28384622751062));
#82477=CARTESIAN_POINT('Ctrl Pts',(-14.837019646162,31.080287834931,-3.19228374588672));
#82478=CARTESIAN_POINT('Ctrl Pts',(-14.8090933737951,31.1694008049856,-3.05046692327928));
#82479=CARTESIAN_POINT('Ctrl Pts',(-14.7811671014282,31.2525866330839,-2.90489286188319));
#82480=CARTESIAN_POINT('Ctrl Pts',(-14.7532408290614,31.3295444076921,-2.75607627006915));
#82481=CARTESIAN_POINT('Ctrl Pts',(-14.7253200369762,31.4064870800239,-2.60728888218287));
#82482=CARTESIAN_POINT('Ctrl Pts',(-14.6973992448909,31.4772039929293,-2.45526051379136));
#82483=CARTESIAN_POINT('Ctrl Pts',(-14.6694784528057,31.5414403126701,-2.30053021304105));
#82484=CARTESIAN_POINT('Ctrl Pts',(-14.6415584660166,31.6056747796963,-2.14580437504755));
#82485=CARTESIAN_POINT('Ctrl Pts',(-14.6136384792275,31.6634289028201,-1.98837705042711));
#82486=CARTESIAN_POINT('Ctrl Pts',(-14.5857184924384,31.7144958357582,-1.82880762878485));
#82487=CARTESIAN_POINT('Ctrl Pts',(-14.5578006231568,31.7655588956783,-1.66925030920596));
#82488=CARTESIAN_POINT('Ctrl Pts',(-14.5298827538752,31.809935683519,-1.5075515179884));
#82489=CARTESIAN_POINT('Ctrl Pts',(-14.5019648845936,31.8474690148528,-1.3442864725705));
#82490=CARTESIAN_POINT('Ctrl Pts',(-14.4740437955224,31.8850066749349,-1.18100259766807));
#82491=CARTESIAN_POINT('Ctrl Pts',(-14.4461227064512,31.9156992309195,-1.01615241518673));
#82492=CARTESIAN_POINT('Ctrl Pts',(-14.4182016173801,31.9394403141167,-0.850322735816167));
#82493=CARTESIAN_POINT('Ctrl Pts',(-14.4082079768031,31.947937828371,-0.790968238274906));
#82494=CARTESIAN_POINT('Ctrl Pts',(-14.3982143362261,31.9555452682394,-0.731488341091311));
#82495=CARTESIAN_POINT('Ctrl Pts',(-14.3882206956492,31.962259361791,-0.671910189486545));
#82496=CARTESIAN_POINT('Ctrl Pts',(-14.3602243452432,31.9810683347855,-0.505006967780993));
#82497=CARTESIAN_POINT('Ctrl Pts',(-14.3322279948373,31.992866437625,-0.337298389795841));
#82498=CARTESIAN_POINT('Ctrl Pts',(-14.3042316444314,31.9976086632807,-0.169382177752417));
#82499=CARTESIAN_POINT('Ctrl Pts',(-14.276238095147,32.0023504144621,-0.00148276624575069));
#82500=CARTESIAN_POINT('Ctrl Pts',(-14.2482445458626,32.0000376891145,0.166623926130821));
#82501=CARTESIAN_POINT('Ctrl Pts',(-14.2202509965782,31.9906775694119,0.334338540022986));
#82502=CARTESIAN_POINT('Ctrl Pts',(-14.192254980999,31.9813166250617,0.502067929951041));
#82503=CARTESIAN_POINT('Ctrl Pts',(-14.1642589654198,31.9649070607109,0.669404860761526));
#82504=CARTESIAN_POINT('Ctrl Pts',(-14.1362629498405,31.9415080128943,0.835752674367886));
#82505=CARTESIAN_POINT('Ctrl Pts',(-14.1082673487604,31.9181093115157,1.00209802508714));
#82506=CARTESIAN_POINT('Ctrl Pts',(-14.0802717476803,31.8877213796004,1.16745397934408));
#82507=CARTESIAN_POINT('Ctrl Pts',(-14.0522761466002,31.8504549319236,1.33123141847328));
#82508=CARTESIAN_POINT('Ctrl Pts',(-14.0242754155985,31.8131816555328,1.49503886822536));
#82509=CARTESIAN_POINT('Ctrl Pts',(-13.9962746845967,31.7690274150913,1.65726692091452));
#82510=CARTESIAN_POINT('Ctrl Pts',(-13.968273953595,31.7181536977392,1.81733824287937));
#82511=CARTESIAN_POINT('Ctrl Pts',(-13.9586565507755,31.7006801170433,1.87231789262844));
#82512=CARTESIAN_POINT('Ctrl Pts',(-13.9490391479559,31.6824142643844,1.92704323551223));
#82513=CARTESIAN_POINT('Ctrl Pts',(-13.9394217451364,31.6633640359077,1.98149130626074));
#82514=CARTESIAN_POINT('Ctrl Pts',(-13.9114908001388,31.6080381965145,2.13961986735324));
#82515=CARTESIAN_POINT('Ctrl Pts',(-13.8835598551412,31.5460761816123,2.29545653429214));
#82516=CARTESIAN_POINT('Ctrl Pts',(-13.8556289101436,31.4776927529954,2.44844483372244));
#82517=CARTESIAN_POINT('Ctrl Pts',(-13.8277036153902,31.4093231578906,2.60140218463854));
#82518=CARTESIAN_POINT('Ctrl Pts',(-13.7997783206368,31.3345348698172,2.75151203023619));
#82519=CARTESIAN_POINT('Ctrl Pts',(-13.7718530258833,31.2535904151959,2.8982387322927));
#82520=CARTESIAN_POINT('Ctrl Pts',(-13.7439288447544,31.1726491885345,3.04495958307862));
#82521=CARTESIAN_POINT('Ctrl Pts',(-13.7160046636256,31.0855524349579,3.18829728220577));
#82522=CARTESIAN_POINT('Ctrl Pts',(-13.6880804824967,30.9926085091711,3.32774101668878));
#82523=CARTESIAN_POINT('Ctrl Pts',(-13.6601586138252,30.8996722802569,3.46717320355674));
#82524=CARTESIAN_POINT('Ctrl Pts',(-13.6322367451537,30.8008900220586,3.60271180823876));
#82525=CARTESIAN_POINT('Ctrl Pts',(-13.6043148764822,30.6966134401082,3.73387495695766));
#82526=CARTESIAN_POINT('Ctrl Pts',(-13.5763901169249,30.5923260619,3.86505168563023));
#82527=CARTESIAN_POINT('Ctrl Pts',(-13.5484653573676,30.4825434194855,3.99185180642084));
#82528=CARTESIAN_POINT('Ctrl Pts',(-13.5205405978103,30.3676579772534,4.11382593138488));
#82529=CARTESIAN_POINT('Ctrl Pts',(-13.510567996748,30.3266296317491,4.15738581542576));
#82530=CARTESIAN_POINT('Ctrl Pts',(-13.5005953956858,30.2849508501425,4.20033052409612));
#82531=CARTESIAN_POINT('Ctrl Pts',(-13.4906227946235,30.2426406871193,4.24264068711928));
#82532=CARTESIAN_POINT('',(-10.3490300976385,21.7573593077119,-4.24264069228803));
#82533=CARTESIAN_POINT('Ctrl Pts',(-13.4906227946235,30.2426406871193,4.24264068711928));
#82534=CARTESIAN_POINT('Ctrl Pts',(-13.4624945102889,30.1233024835425,4.36197889069605));
#82535=CARTESIAN_POINT('Ctrl Pts',(-13.4343662259543,29.9989203714952,4.47628452432291));
#82536=CARTESIAN_POINT('Ctrl Pts',(-13.4062379416198,29.8699388455358,4.58514703491752));
#82537=CARTESIAN_POINT('Ctrl Pts',(-13.3781114359764,29.7409654757192,4.69400266159471));
#82538=CARTESIAN_POINT('Ctrl Pts',(-13.3499849303329,29.6073935062869,4.7974156559258));
#82539=CARTESIAN_POINT('Ctrl Pts',(-13.3218584246895,29.4697010859089,4.89501525783557));
#82540=CARTESIAN_POINT('Ctrl Pts',(-13.2937292681557,29.3319956881806,4.99262405839415));
#82541=CARTESIAN_POINT('Ctrl Pts',(-13.2656001116219,29.1901693115166,5.08441819351467));
#82542=CARTESIAN_POINT('Ctrl Pts',(-13.2374709550881,29.0447303746263,5.17006933665578));
#82543=CARTESIAN_POINT('Ctrl Pts',(-13.2093424954878,28.8992950411596,5.25571835768733));
#82544=CARTESIAN_POINT('Ctrl Pts',(-13.1812140358875,28.7502475906313,5.3352245379556));
#82545=CARTESIAN_POINT('Ctrl Pts',(-13.1530855762872,28.5981226861008,5.40830458720368));
#82546=CARTESIAN_POINT('Ctrl Pts',(-13.124953455114,28.445977978978,5.48139414951888));
#82547=CARTESIAN_POINT('Ctrl Pts',(-13.0968213339409,28.2907552928954,5.54805577763542));
#82548=CARTESIAN_POINT('Ctrl Pts',(-13.0686892127677,28.1330117341137,5.60805322212025));
#82549=CARTESIAN_POINT('Ctrl Pts',(-13.059734089882,28.0827982097007,5.62715183487265));
#82550=CARTESIAN_POINT('Ctrl Pts',(-13.0507789669963,28.0323293967946,5.64557553127911));
#82551=CARTESIAN_POINT('Ctrl Pts',(-13.0418238441107,27.9816236668424,5.66331772400333));
#82552=CARTESIAN_POINT('Ctrl Pts',(-13.0139494836753,27.8237933600043,5.71854335085626));
#82553=CARTESIAN_POINT('Ctrl Pts',(-12.98607512324,27.6636310460951,5.76717473111242));
#82554=CARTESIAN_POINT('Ctrl Pts',(-12.9582007628047,27.5017039866551,5.80903478526892));
#82555=CARTESIAN_POINT('Ctrl Pts',(-12.9303304260567,27.339800301522,5.85088879689147));
#82556=CARTESIAN_POINT('Ctrl Pts',(-12.9024600893088,27.1761326868282,5.88597335365304));
#82557=CARTESIAN_POINT('Ctrl Pts',(-12.8745897525608,27.0112817505993,5.91416175133085));
#82558=CARTESIAN_POINT('Ctrl Pts',(-12.8467176433771,26.8464203305474,5.94235194167167));
#82559=CARTESIAN_POINT('Ctrl Pts',(-12.8188455341935,26.6803757513683,5.96364504013599));
#82560=CARTESIAN_POINT('Ctrl Pts',(-12.7909734250098,26.5137376787702,5.97796567382349));
#82561=CARTESIAN_POINT('Ctrl Pts',(-12.7631018264686,26.3471026591335,5.99228604514393));
#82562=CARTESIAN_POINT('Ctrl Pts',(-12.7352302279274,26.1798744846817,5.99963418241472));
#82563=CARTESIAN_POINT('Ctrl Pts',(-12.7073586293862,26.0126470084994,5.99998667108321));
#82564=CARTESIAN_POINT('Ctrl Pts',(-12.6794811226982,25.845384083885,6.00033923447129));
#82565=CARTESIAN_POINT('Ctrl Pts',(-12.6516036160103,25.6781221757056,5.99369318675545));
#82566=CARTESIAN_POINT('Ctrl Pts',(-12.6237261093223,25.5114549724733,5.98007723663156));
#82567=CARTESIAN_POINT('Ctrl Pts',(-12.6134923707475,25.45027200493,5.97507886731628));
#82568=CARTESIAN_POINT('Ctrl Pts',(-12.6032586321727,25.3891691506621,5.9691417404092));
#82569=CARTESIAN_POINT('Ctrl Pts',(-12.5930248935979,25.3281756306373,5.96226903256893));
#82570=CARTESIAN_POINT('Ctrl Pts',(-12.565038533079,25.161375723814,5.94347413391556));
#82571=CARTESIAN_POINT('Ctrl Pts',(-12.53705217256,24.9953411938198,5.91767266664919));
#82572=CARTESIAN_POINT('Ctrl Pts',(-12.5090658120411,24.8306644414388,5.88495151649395));
#82573=CARTESIAN_POINT('Ctrl Pts',(-12.4810844029258,24.6660168240021,5.85223615543083));
#82574=CARTESIAN_POINT('Ctrl Pts',(-12.4531029938104,24.5027268112747,5.81260361565926));
#82575=CARTESIAN_POINT('Ctrl Pts',(-12.425121584695,24.3413770249947,5.76619196929694));
#82576=CARTESIAN_POINT('Ctrl Pts',(-12.3971407460117,24.1800305280088,5.71978126908746));
#82577=CARTESIAN_POINT('Ctrl Pts',(-12.3691599073283,24.0206244797569,5.66659182174747));
#82578=CARTESIAN_POINT('Ctrl Pts',(-12.341179068645,23.8637274319567,5.60681188511132));
#82579=CARTESIAN_POINT('Ctrl Pts',(-12.313200365528,23.7068423589246,5.54703651102683));
#82580=CARTESIAN_POINT('Ctrl Pts',(-12.285221662411,23.5524661955205,5.48067176487843));
#82581=CARTESIAN_POINT('Ctrl Pts',(-12.2572429592941,23.4011488772566,5.40795458947422));
#82582=CARTESIAN_POINT('Ctrl Pts',(-12.229261507797,23.2498166949191,5.33523027097856));
#82583=CARTESIAN_POINT('Ctrl Pts',(-12.2012800563,23.1015442398978,5.25615241184179));
#82584=CARTESIAN_POINT('Ctrl Pts',(-12.1732986048029,22.956858815793,5.1710049055269));
#82585=CARTESIAN_POINT('Ctrl Pts',(-12.1636077175636,22.9067495450027,5.14151555317889));
#82586=CARTESIAN_POINT('Ctrl Pts',(-12.1539168303243,22.8570703051347,5.11129857214482));
#82587=CARTESIAN_POINT('Ctrl Pts',(-12.144225943085,22.8078422705457,5.08036701728184));
#82588=CARTESIAN_POINT('Ctrl Pts',(-12.1162733741538,22.6658480448137,4.99114748576642));
#82589=CARTESIAN_POINT('Ctrl Pts',(-12.0883208052225,22.5275823738739,4.89596231205403));
#82590=CARTESIAN_POINT('Ctrl Pts',(-12.0603682362912,22.3935393131819,4.79514768431963));
#82591=CARTESIAN_POINT('Ctrl Pts',(-12.0324186026479,22.2595103282974,4.69434364308838));
#82592=CARTESIAN_POINT('Ctrl Pts',(-12.0044689690045,22.1297033193408,4.58791151666546));
#82593=CARTESIAN_POINT('Ctrl Pts',(-11.9765193353612,22.0045811655867,4.47622925436303));
#82594=CARTESIAN_POINT('Ctrl Pts',(-11.9485670282336,21.8794470434428,4.3645363092454));
#82595=CARTESIAN_POINT('Ctrl Pts',(-11.9206147211059,21.758998907872,4.24759243207913));
#82596=CARTESIAN_POINT('Ctrl Pts',(-11.8926624139783,21.6436650824415,4.12581459666584));
#82597=CARTESIAN_POINT('Ctrl Pts',(-11.8647102876227,21.5283320028931,4.00403754880902));
#82598=CARTESIAN_POINT('Ctrl Pts',(-11.8367581612671,21.4181133811633,3.87742683525044));
#82599=CARTESIAN_POINT('Ctrl Pts',(-11.8088060349114,21.3133994780108,3.74643504511826));
#82600=CARTESIAN_POINT('Ctrl Pts',(-11.7808481081224,21.2086638453477,3.61541607246872));
#82601=CARTESIAN_POINT('Ctrl Pts',(-11.7528901813333,21.1094354088864,3.48001445278672));
#82602=CARTESIAN_POINT('Ctrl Pts',(-11.7249322545442,21.0160635480069,3.34071510944811));
#82603=CARTESIAN_POINT('Ctrl Pts',(-11.7150971672202,20.9832170350203,3.29171214809656));
#82604=CARTESIAN_POINT('Ctrl Pts',(-11.7052620798962,20.9510948904246,3.24222711380554));
#82605=CARTESIAN_POINT('Ctrl Pts',(-11.6954269925722,20.9197110486641,3.19228196920867));
#82606=CARTESIAN_POINT('Ctrl Pts',(-11.6675007278284,20.8305981160787,3.05046509613738));
#82607=CARTESIAN_POINT('Ctrl Pts',(-11.6395744630847,20.747412334659,2.90489099532772));
#82608=CARTESIAN_POINT('Ctrl Pts',(-11.611648198341,20.670454613249,2.75607437681959));
#82609=CARTESIAN_POINT('Ctrl Pts',(-11.5837274109289,20.5935119859795,2.60728694653193));
#82610=CARTESIAN_POINT('Ctrl Pts',(-11.5558066235168,20.5227951259649,2.45525854777079));
#82611=CARTESIAN_POINT('Ctrl Pts',(-11.5278858361047,20.4585588640983,2.30052823006726));
#82612=CARTESIAN_POINT('Ctrl Pts',(-11.4999658496265,20.3943244449088,2.14580235094729));
#82613=CARTESIAN_POINT('Ctrl Pts',(-11.4720458631482,20.3365703766266,1.98837499777321));
#82614=CARTESIAN_POINT('Ctrl Pts',(-11.44412587667,20.2855035025929,1.82880556132206));
#82615=CARTESIAN_POINT('Ctrl Pts',(-11.4162080051734,20.2344404969532,1.66924821250002));
#82616=CARTESIAN_POINT('Ctrl Pts',(-11.3882901336769,20.1900637686612,1.50754940539573));
#82617=CARTESIAN_POINT('Ctrl Pts',(-11.3603722621804,20.1525304990906,1.34428435828654));
#82618=CARTESIAN_POINT('Ctrl Pts',(-11.3324511672218,20.1149928958417,1.1810004602169));
#82619=CARTESIAN_POINT('Ctrl Pts',(-11.3045300722631,20.0843004007024,1.01615026835585));
#82620=CARTESIAN_POINT('Ctrl Pts',(-11.2766089773045,20.0605593792441,0.850320593961511));
#82621=CARTESIAN_POINT('Ctrl Pts',(-11.2666153322228,20.052061885049,0.790966083962213));
#82622=CARTESIAN_POINT('Ctrl Pts',(-11.2566216871411,20.0444544657807,0.731486176094842));
#82623=CARTESIAN_POINT('Ctrl Pts',(-11.2466280420594,20.0377403932269,0.671908015610335));
#82624=CARTESIAN_POINT('Ctrl Pts',(-11.2186317076778,20.0189314982998,0.505004939793092));
#82625=CARTESIAN_POINT('Ctrl Pts',(-11.1906353732962,20.007133461194,0.337296513475724));
#82626=CARTESIAN_POINT('Ctrl Pts',(-11.1626390389146,20.0023912881466,0.169380457846953));
#82627=CARTESIAN_POINT('Ctrl Pts',(-11.1346455050256,19.997649589462,0.00148119897672991));
#82628=CARTESIAN_POINT('Ctrl Pts',(-11.1066519711366,19.9999623544989,-0.166625336025476));
#82629=CARTESIAN_POINT('Ctrl Pts',(-11.0786584372476,20.0093225002884,-0.33433978891192));
#82630=CARTESIAN_POINT('Ctrl Pts',(-11.0506624358882,20.0186834711215,-0.502069024871426));
#82631=CARTESIAN_POINT('Ctrl Pts',(-11.0226664345287,20.0350930489421,-0.669405798047149));
#82632=CARTESIAN_POINT('Ctrl Pts',(-10.9946704331693,20.0584920964223,-0.835753451517604));
#82633=CARTESIAN_POINT('Ctrl Pts',(-10.9666748455537,20.0818907980955,-1.00209864658985));
#82634=CARTESIAN_POINT('Ctrl Pts',(-10.9386792579381,20.1122787168752,-1.16745444264423));
#82635=CARTESIAN_POINT('Ctrl Pts',(-10.9106836703225,20.1495451372064,-1.33123172228389));
#82636=CARTESIAN_POINT('Ctrl Pts',(-10.8826829514969,20.1868183879651,-1.49503902006914));
#82637=CARTESIAN_POINT('Ctrl Pts',(-10.8546822326712,20.2309725891922,-1.65726691935743));
#82638=CARTESIAN_POINT('Ctrl Pts',(-10.8266815138456,20.2818462529875,-1.81733808784359));
#82639=CARTESIAN_POINT('Ctrl Pts',(-10.8170640397459,20.2993199523933,-1.87231811627087));
#82640=CARTESIAN_POINT('Ctrl Pts',(-10.8074465656462,20.3175859345044,-1.92704383383409));
#82641=CARTESIAN_POINT('Ctrl Pts',(-10.7978290915466,20.336636302958,-1.9814922747834));
#82642=CARTESIAN_POINT('Ctrl Pts',(-10.769897967176,20.3919624941248,-2.13962175453832));
#82643=CARTESIAN_POINT('Ctrl Pts',(-10.7419668428055,20.4539249378764,-2.29545931101644));
#82644=CARTESIAN_POINT('Ctrl Pts',(-10.714035718435,20.522308869905,-2.44844846449311));
#82645=CARTESIAN_POINT('Ctrl Pts',(-10.6861102453204,20.5906789659313,-2.60140666393984));
#82646=CARTESIAN_POINT('Ctrl Pts',(-10.6581847722058,20.6654678290136,-2.75151732279546));
#82647=CARTESIAN_POINT('Ctrl Pts',(-10.6302592990912,20.7464129302101,-2.89824479644781));
#82648=CARTESIAN_POINT('Ctrl Pts',(-10.6023349425737,20.8273547948253,-3.04496640321761));
#82649=CARTESIAN_POINT('Ctrl Pts',(-10.5744105860562,20.9144522566137,-3.18830481739469));
#82650=CARTESIAN_POINT('Ctrl Pts',(-10.5464862295387,21.0073969583467,-3.32774921958888));
#82651=CARTESIAN_POINT('Ctrl Pts',(-10.5185641876098,21.1003339560975,-3.46718206354282));
#82652=CARTESIAN_POINT('Ctrl Pts',(-10.4906421456808,21.1991170499757,-3.60272127857529));
#82653=CARTESIAN_POINT('Ctrl Pts',(-10.4627201037519,21.3033945318271,-3.73388498434647));
#82654=CARTESIAN_POINT('Ctrl Pts',(-10.4347951752472,21.4076827938663,-3.86506224979871));
#82655=CARTESIAN_POINT('Ctrl Pts',(-10.4068702467424,21.5174663826501,-3.99186285542055));
#82656=CARTESIAN_POINT('Ctrl Pts',(-10.3789453182376,21.6323528310669,-4.1138374065719));
#82657=CARTESIAN_POINT('Ctrl Pts',(-10.368973592503,21.6733776864767,-4.15739335589082));
#82658=CARTESIAN_POINT('Ctrl Pts',(-10.3590018667683,21.7150528635581,-4.20033423779668));
#82659=CARTESIAN_POINT('Ctrl Pts',(-10.3490301410337,21.7573593128807,-4.24264068711927));
#82660=CARTESIAN_POINT('Ctrl Pts',(-10.3490300482133,21.7573593128807,-4.24264068711927));
#82661=CARTESIAN_POINT('Ctrl Pts',(-10.3209012858048,21.8766995447535,-4.36198091899205));
#82662=CARTESIAN_POINT('Ctrl Pts',(-10.2927725233962,22.0010838302075,-4.47628838371058));
#82663=CARTESIAN_POINT('Ctrl Pts',(-10.2646437609877,22.1300676541458,-4.5851525207469));
#82664=CARTESIAN_POINT('Ctrl Pts',(-10.2365167703473,22.2590433536801,-4.69400980067342));
#82665=CARTESIAN_POINT('Ctrl Pts',(-10.208389779707,22.3926177796726,-4.79742424096074));
#82666=CARTESIAN_POINT('Ctrl Pts',(-10.1802627890666,22.5303127634901,-4.89502507458337));
#82667=CARTESIAN_POINT('Ctrl Pts',(-10.1521331422088,22.6680207507538,-4.99263512529695));
#82668=CARTESIAN_POINT('Ctrl Pts',(-10.1240034953511,22.8098498254159,-5.08443029412364));
#82669=CARTESIAN_POINT('Ctrl Pts',(-10.0958738484933,22.9552915492135,-5.17008224786698));
#82670=CARTESIAN_POINT('Ctrl Pts',(-10.067744896948,23.100729677963,-5.25573208445378));
#82671=CARTESIAN_POINT('Ctrl Pts',(-10.0396159454026,23.2497800131169,-5.3352388564859));
#82672=CARTESIAN_POINT('Ctrl Pts',(-10.0114869938573,23.4019078724027,-5.40831926725084));
#82673=CARTESIAN_POINT('Ctrl Pts',(-9.98335438226454,23.554055526069,-5.48140918700032));
#82674=CARTESIAN_POINT('Ctrl Pts',(-9.95522177067182,23.7092812285162,-5.54807094298151));
#82675=CARTESIAN_POINT('Ctrl Pts',(-9.9270891590791,23.8670278544895,-5.60806827940568));
#82676=CARTESIAN_POINT('Ctrl Pts',(-9.91813647195288,23.9172278219863,-5.62716133017494));
#82677=CARTESIAN_POINT('Ctrl Pts',(-9.90918378482667,23.967682935363,-5.64557983134726));
#82678=CARTESIAN_POINT('Ctrl Pts',(-9.90023109770045,24.01837483853,-5.66331720102528));
#82679=CARTESIAN_POINT('Ctrl Pts',(-9.8723571003697,24.1762029803656,-5.7185421170856));
#82680=CARTESIAN_POINT('Ctrl Pts',(-9.84448310303895,24.336363124577,-5.76717298671253));
#82681=CARTESIAN_POINT('Ctrl Pts',(-9.8166091057082,24.4982880286785,-5.80903272113263));
#82682=CARTESIAN_POINT('Ctrl Pts',(-9.78873914432011,24.6601894872864,-5.85088639458181));
#82683=CARTESIAN_POINT('Ctrl Pts',(-9.76086918293202,24.82385488824,-5.88597080996578));
#82684=CARTESIAN_POINT('Ctrl Pts',(-9.73299922154392,24.9887036411706,-5.91415925340351));
#82685=CARTESIAN_POINT('Ctrl Pts',(-9.70512750269832,25.1535627893319,-5.94234947438196));
#82686=CARTESIAN_POINT('Ctrl Pts',(-9.67725578385272,25.3196051257821,-5.96364279802991));
#82687=CARTESIAN_POINT('Ctrl Pts',(-9.64938406500712,25.4862410014732,-5.97796384159628));
#82688=CARTESIAN_POINT('Ctrl Pts',(-9.62151286463947,25.6528737773544,-5.99228461875837));
#82689=CARTESIAN_POINT('Ctrl Pts',(-9.59364166427182,25.8200997535212,-5.99963335046843));
#82690=CARTESIAN_POINT('Ctrl Pts',(-9.56577046390418,25.9873250923379,-5.99998661221137));
#82691=CARTESIAN_POINT('Ctrl Pts',(-9.53789336415152,26.1545858270703,-6.00033994872781));
#82692=CARTESIAN_POINT('Ctrl Pts',(-9.51001626439885,26.3218456062963,-5.99369485719773));
#82693=CARTESIAN_POINT('Ctrl Pts',(-9.48213916464618,26.4885107560557,-5.98008003635552));
#82694=CARTESIAN_POINT('Ctrl Pts',(-9.47190349216001,26.5497054249033,-5.9750810641405));
#82695=CARTESIAN_POINT('Ctrl Pts',(-9.46166781967383,26.6108199580132,-5.96914297538562));
#82696=CARTESIAN_POINT('Ctrl Pts',(-9.45143214718766,26.6718251172582,-5.96226894829653));
#82697=CARTESIAN_POINT('Ctrl Pts',(-9.42344576703072,26.8386254501595,-5.9434739804442));
#82698=CARTESIAN_POINT('Ctrl Pts',(-9.39545938687379,27.004660375534,-5.91767241102094));
#82699=CARTESIAN_POINT('Ctrl Pts',(-9.36747300671686,27.1693374907124,-5.88495113257657));
#82700=CARTESIAN_POINT('Ctrl Pts',(-9.3394915717959,27.333985507194,-5.8522356360319));
#82701=CARTESIAN_POINT('Ctrl Pts',(-9.31151013687494,27.4972758858009,-5.81260293161189));
#82702=CARTESIAN_POINT('Ctrl Pts',(-9.28352870195398,27.6586260035525,-5.76619109814611));
#82703=CARTESIAN_POINT('Ctrl Pts',(-9.25554782894945,27.8199728811099,-5.71978019671158));
#82704=CARTESIAN_POINT('Ctrl Pts',(-9.22756695594493,27.9793792743505,-5.66659052157172));
#82705=CARTESIAN_POINT('Ctrl Pts',(-9.19958608294041,28.1362766307547,-5.60681033716064));
#82706=CARTESIAN_POINT('Ctrl Pts',(-9.17160734074356,28.2931620390651,-5.54703470514777));
#82707=CARTESIAN_POINT('Ctrl Pts',(-9.14362859854671,28.4475385005199,-5.48066967886209));
#82708=CARTESIAN_POINT('Ctrl Pts',(-9.11564985634986,28.5988560794148,-5.40795220748931));
#82709=CARTESIAN_POINT('Ctrl Pts',(-9.08766835933929,28.7501885571833,-5.33522757628474));
#82710=CARTESIAN_POINT('Ctrl Pts',(-9.05968686232871,28.8984612688081,-5.25614938568914));
#82711=CARTESIAN_POINT('Ctrl Pts',(-9.03170536531814,29.0431469109443,-5.17100153533239));
#82712=CARTESIAN_POINT('Ctrl Pts',(-9.02201464243703,29.0932553258832,-5.14151261194071));
#82713=CARTESIAN_POINT('Ctrl Pts',(-9.01232391955593,29.1429337212672,-5.11129608540006));
#82714=CARTESIAN_POINT('Ctrl Pts',(-9.00263319667482,29.1921609239478,-5.08036501007758));
#82715=CARTESIAN_POINT('Ctrl Pts',(-8.97454195866122,29.3348595733893,-4.99070274137374));
#82716=CARTESIAN_POINT('Ctrl Pts',(-8.94645072064762,29.473791457817,-4.89501624427522));
#82717=CARTESIAN_POINT('Ctrl Pts',(-8.91835948263403,29.6084577278052,-4.79364504595855));
#82718=CARTESIAN_POINT('Ctrl Pts',(-8.8902701958346,29.7431146438897,-4.69228088887367));
#82719=CARTESIAN_POINT('Ctrl Pts',(-8.86218090903517,29.8735062904475,-4.58523300206302));
#82720=CARTESIAN_POINT('Ctrl Pts',(-8.83409162223575,29.9991649005209,-4.47288275035703));
#82721=CARTESIAN_POINT('Ctrl Pts',(-8.81547232218614,30.0824591251654,-4.39841012091293));
#82722=CARTESIAN_POINT('Ctrl Pts',(-8.79685302213653,30.1636743680789,-4.3216085697427));
#82723=CARTESIAN_POINT('Ctrl Pts',(-8.77823372208692,30.2426826788146,-4.24259869500835));
#82724=CARTESIAN_POINT('Origin',(-31.4159265358979,26.,7.7715611723761E-15));
#82725=CARTESIAN_POINT('',(-0.646543496119136,30.2426884810913,-4.2425928926089));
#82726=CARTESIAN_POINT('',(-2.4950483220781,30.2426872863809,-4.24259408734582));
#82727=CARTESIAN_POINT('',(-31.4159265358979,30.2426406871193,-4.24264068711928));
#82728=CARTESIAN_POINT('',(-2.21733987300771,21.7573593180495,-4.24264068195053));
#82729=CARTESIAN_POINT('Ctrl Pts',(-0.646543496119133,30.2426884810913,
-4.24259289260889));
#82730=CARTESIAN_POINT('Ctrl Pts',(-0.674631828671807,30.1234996154242,
-4.36178444368155));
#82731=CARTESIAN_POINT('Ctrl Pts',(-0.702720161224486,29.9992866956845,
-4.47594853295759));
#82732=CARTESIAN_POINT('Ctrl Pts',(-0.730808493777161,29.8704949120925,
-4.58467764793407));
#82733=CARTESIAN_POINT('Ctrl Pts',(-0.758901295988709,29.7416826340358,
-4.69342406482951));
#82734=CARTESIAN_POINT('Ctrl Pts',(-0.78699409820026,29.6082902705929,-4.79673358053653));
#82735=CARTESIAN_POINT('Ctrl Pts',(-0.81508690041181,29.470796620725,-4.89423853296546));
#82736=CARTESIAN_POINT('Ctrl Pts',(-0.8337055909559,29.3796717945368,-4.95886058533744));
#82737=CARTESIAN_POINT('Ctrl Pts',(-0.852324281499978,29.2867461748589,
-5.02093383373948));
#82738=CARTESIAN_POINT('Ctrl Pts',(-0.870942972044066,29.1921664334504,
-5.0803615482712));
#82739=CARTESIAN_POINT('Ctrl Pts',(-0.898924591431005,29.0500246260263,
-5.16967414977368));
#82740=CARTESIAN_POINT('Ctrl Pts',(-0.926906210817951,28.9041190310538,
-5.25302596012802));
#82741=CARTESIAN_POINT('Ctrl Pts',(-0.954887830204889,28.7549680880225,
-5.33011733773072));
#82742=CARTESIAN_POINT('Ctrl Pts',(-0.982866636230461,28.6058321411033,
-5.40720096432014));
#82743=CARTESIAN_POINT('Ctrl Pts',(-1.01084544225603,28.4534517752157,-5.47802527131782));
#82744=CARTESIAN_POINT('Ctrl Pts',(-1.0388242482816,28.2983695092723,-5.54233683556378));
#82745=CARTESIAN_POINT('Ctrl Pts',(-1.06680563972006,28.1432729127786,-5.6066543425918));
#82746=CARTESIAN_POINT('Ctrl Pts',(-1.09478703115852,27.9854742052433,-5.66445778234588));
#82747=CARTESIAN_POINT('Ctrl Pts',(-1.12276842259697,27.8255360592375,-5.71554180252613));
#82748=CARTESIAN_POINT('Ctrl Pts',(-1.15074950738818,27.6655996659891,-5.7666252628781));
#82749=CARTESIAN_POINT('Ctrl Pts',(-1.17873059217939,27.5035241798124,-5.81098935838577));
#82750=CARTESIAN_POINT('Ctrl Pts',(-1.2067116769706,27.3398878506923,-5.84847848141439));
#82751=CARTESIAN_POINT('Ctrl Pts',(-1.23469815980102,27.1762199532706,-5.88597483674862));
#82752=CARTESIAN_POINT('Ctrl Pts',(-1.26268464263146,27.0109909162775,-5.91659350071789));
#82753=CARTESIAN_POINT('Ctrl Pts',(-1.29067112546188,26.8447903916065,-5.94022972571342));
#82754=CARTESIAN_POINT('Ctrl Pts',(-1.30036139116022,26.7872437805148,-5.94841372302741));
#82755=CARTESIAN_POINT('Ctrl Pts',(-1.31005165685856,26.7295807759789,-5.95576106384891));
#82756=CARTESIAN_POINT('Ctrl Pts',(-1.3197419225569,26.6718260604999,-5.9622688420125));
#82757=CARTESIAN_POINT('Ctrl Pts',(-1.34761817735919,26.5056814763528,-5.98098994708151));
#82758=CARTESIAN_POINT('Ctrl Pts',(-1.37549443216149,26.3387253218434,-5.99276527668446));
#82759=CARTESIAN_POINT('Ctrl Pts',(-1.4033706869638,26.1715498460393,-5.99754705278115));
#82760=CARTESIAN_POINT('Ctrl Pts',(-1.43124158161395,26.0044065153706,-6.00232790941976));
#82761=CARTESIAN_POINT('Ctrl Pts',(-1.45911247626411,25.8370442651252,-6.0001178868363));
#82762=CARTESIAN_POINT('Ctrl Pts',(-1.48698337091426,25.6700572898176,-5.99092128207319));
#82763=CARTESIAN_POINT('Ctrl Pts',(-1.51485406973379,25.5030714878188,-5.98172474192863));
#82764=CARTESIAN_POINT('Ctrl Pts',(-1.54272476855332,25.3364612730271,-5.96554173164693));
#82765=CARTESIAN_POINT('Ctrl Pts',(-1.57059546737285,25.1708183503036,-5.94242861057722));
#82766=CARTESIAN_POINT('Ctrl Pts',(-1.59846451933102,25.0051852153121,-5.91931685524672));
#82767=CARTESIAN_POINT('Ctrl Pts',(-1.62633357128919,24.8405195727728,-5.88927585270327));
#82768=CARTESIAN_POINT('Ctrl Pts',(-1.65420262324735,24.6774058013829,-5.85241356927074));
#82769=CARTESIAN_POINT('Ctrl Pts',(-1.68207593600995,24.514267092084,-5.81554565008924));
#82770=CARTESIAN_POINT('Ctrl Pts',(-1.70994924877255,24.3526810379655,-5.7718544368111));
#82771=CARTESIAN_POINT('Ctrl Pts',(-1.73782256153514,24.1932203771043,-5.72149870176414));
#82772=CARTESIAN_POINT('Ctrl Pts',(-1.74806199871334,24.134641497974,-5.70300020501327));
#82773=CARTESIAN_POINT('Ctrl Pts',(-1.75830143589153,24.0763493030335,-5.68360281467021));
#82774=CARTESIAN_POINT('Ctrl Pts',(-1.76854087306972,24.0183716559267,-5.66331608741428));
#82775=CARTESIAN_POINT('Ctrl Pts',(-1.79667445855355,23.8590739267015,-5.60757685433833));
#82776=CARTESIAN_POINT('Ctrl Pts',(-1.82480804403738,23.7021159420866,-5.54510773076916));
#82777=CARTESIAN_POINT('Ctrl Pts',(-1.85294162952121,23.5480610580687,-5.47612960265194));
#82778=CARTESIAN_POINT('Ctrl Pts',(-1.88107174638236,23.3940251676578,-5.40715997892888));
#82779=CARTESIAN_POINT('Ctrl Pts',(-1.90920186324351,23.242891941793,-5.33168307752339));
#82780=CARTESIAN_POINT('Ctrl Pts',(-1.93733198010466,23.0952036305205,-5.24996743340936));
#82781=CARTESIAN_POINT('Ctrl Pts',(-1.96546224351292,22.9475145498487,-5.16825136358818));
#82782=CARTESIAN_POINT('Ctrl Pts',(-1.9935925069212,22.803270687939,-5.08029663171037));
#82783=CARTESIAN_POINT('Ctrl Pts',(-2.02172277032946,22.662989291288,-4.98641750457591));
#82784=CARTESIAN_POINT('Ctrl Pts',(-2.04985087654862,22.5227186522149,-4.89254557662859));
#82785=CARTESIAN_POINT('Ctrl Pts',(-2.07797898276777,22.3864101243919,-4.79275033176879));
#82786=CARTESIAN_POINT('Ctrl Pts',(-2.10610708898693,22.2545519110613,-4.68738931742023));
#82787=CARTESIAN_POINT('Ctrl Pts',(-2.13423674266047,22.1226864436138,-4.58202250668559));
#82788=CARTESIAN_POINT('Ctrl Pts',(-2.162366396334,21.99527201849,-4.47108950501785));
#82789=CARTESIAN_POINT('Ctrl Pts',(-2.19049605000754,21.8727642991052,-4.3549885728047));
#82790=CARTESIAN_POINT('Ctrl Pts',(-2.19944397453254,21.8337951088156,-4.31805735456851));
#82791=CARTESIAN_POINT('Ctrl Pts',(-2.20839189905755,21.7953221415358,-4.28060351577433));
#82792=CARTESIAN_POINT('Ctrl Pts',(-2.21733982358255,21.7573593128807,-4.24264068711927));
#82793=CARTESIAN_POINT('',(-5.35893256999276,30.2426406871193,4.24264068711929));
#82794=CARTESIAN_POINT('Ctrl Pts',(-2.21733991640297,21.7573593128807,-4.24264068711927));
#82795=CARTESIAN_POINT('Ctrl Pts',(-2.24526622497855,21.6388780198769,-4.12415939411543));
#82796=CARTESIAN_POINT('Ctrl Pts',(-2.27319253355414,21.5253506939012,-4.00069969038654));
#82797=CARTESIAN_POINT('Ctrl Pts',(-2.30111884212972,21.4171835885019,-3.87269850859888));
#82798=CARTESIAN_POINT('Ctrl Pts',(-2.329042244992,21.309027737816,-3.74471064524665));
#82799=CARTESIAN_POINT('Ctrl Pts',(-2.35696564785428,21.206231197651,-3.61218248780336));
#82800=CARTESIAN_POINT('Ctrl Pts',(-2.38488905071656,21.1091605367417,-3.47558474859055));
#82801=CARTESIAN_POINT('Ctrl Pts',(-2.4128153837417,21.012079689651,-3.33897267539329));
#82802=CARTESIAN_POINT('Ctrl Pts',(-2.44074171676684,20.9207261070017,-3.19829042261256));
#82803=CARTESIAN_POINT('Ctrl Pts',(-2.46866804979198,20.8354239848706,-3.0540390606458));
#82804=CARTESIAN_POINT('Ctrl Pts',(-2.49659440842889,20.7501217845073,-2.90978756638336));
#82805=CARTESIAN_POINT('Ctrl Pts',(-2.52452076706581,20.6708712133814,-2.76196722932661));
#82806=CARTESIAN_POINT('Ctrl Pts',(-2.55244712570272,20.5979514241649,-2.61110535680167));
#82807=CARTESIAN_POINT('Ctrl Pts',(-2.58037976170836,20.5250152438246,-2.46020957310296));
#82808=CARTESIAN_POINT('Ctrl Pts',(-2.608312397714,20.4584128247526,-2.30627117225125));
#82809=CARTESIAN_POINT('Ctrl Pts',(-2.63624503371964,20.3983762599628,-2.14983987195589));
#82810=CARTESIAN_POINT('Ctrl Pts',(-2.64620964478503,20.3769589824201,-2.09403500393051));
#82811=CARTESIAN_POINT('Ctrl Pts',(-2.65617425585041,20.3563768384129,-2.03791306921283));
#82812=CARTESIAN_POINT('Ctrl Pts',(-2.6661388669158,20.3366388642348,-1.98149959523188));
#82813=CARTESIAN_POINT('Ctrl Pts',(-2.69413936958568,20.2811752645975,-1.82297804145962));
#82814=CARTESIAN_POINT('Ctrl Pts',(-2.72213987225557,20.232363981333,-1.66210497024651));
#82815=CARTESIAN_POINT('Ctrl Pts',(-2.75014037492545,20.1903836434445,-1.49945249662752));
#82816=CARTESIAN_POINT('Ctrl Pts',(-2.77813615756997,20.1484103821525,-1.33682744122351));
#82817=CARTESIAN_POINT('Ctrl Pts',(-2.80613194021447,20.1132658459979,-1.17242388398358));
#82818=CARTESIAN_POINT('Ctrl Pts',(-2.83412772285899,20.0850782955521,-1.0068273090513));
#82819=CARTESIAN_POINT('Ctrl Pts',(-2.86212314122732,20.0568911118777,-0.841232888832398));
#82820=CARTESIAN_POINT('Ctrl Pts',(-2.89011855959567,20.0356607884437,-0.674445788908477));
#82821=CARTESIAN_POINT('Ctrl Pts',(-2.918113977964,20.021464261399,-0.507060570613027));
#82822=CARTESIAN_POINT('Ctrl Pts',(-2.94610734130233,20.0072687764636,-0.339687639386882));
#82823=CARTESIAN_POINT('Ctrl Pts',(-2.97410070464067,20.0001060815898,-0.171716988407973));
#82824=CARTESIAN_POINT('Ctrl Pts',(-3.002094067979,20.0000011703201,-0.00374751118958749));
#82825=CARTESIAN_POINT('Ctrl Pts',(-3.030090186961,19.9998962487231,0.164238500805971));
#82826=CARTESIAN_POINT('Ctrl Pts',(-3.05808630594298,20.0068504990882,0.332223026852808));
#82827=CARTESIAN_POINT('Ctrl Pts',(-3.08608242492498,20.0208367943488,0.499607205900024));
#82828=CARTESIAN_POINT('Ctrl Pts',(-3.09570088909286,20.0256419846644,0.55711441714853));
#82829=CARTESIAN_POINT('Ctrl Pts',(-3.10531935326074,20.0312767601218,0.614550788877512));
#82830=CARTESIAN_POINT('Ctrl Pts',(-3.11493781742862,20.0377386045537,0.67189214340621));
#82831=CARTESIAN_POINT('Ctrl Pts',(-3.14285895277454,20.0564964883302,0.838346547432625));
#82832=CARTESIAN_POINT('Ctrl Pts',(-3.17078008812047,20.0822314018542,1.00403360360904));
#82833=CARTESIAN_POINT('Ctrl Pts',(-3.19870122346638,20.1148554295047,1.16836354974373));
#82834=CARTESIAN_POINT('Ctrl Pts',(-3.22661912933023,20.1474756837158,1.33267448874964));
#82835=CARTESIAN_POINT('Ctrl Pts',(-3.25453703519406,20.1869834000549,1.49562832166912));
#82836=CARTESIAN_POINT('Ctrl Pts',(-3.28245494105791,20.2332395035258,1.65664521739113));
#82837=CARTESIAN_POINT('Ctrl Pts',(-3.31037536935724,20.279499786323,1.81767666129358));
#82838=CARTESIAN_POINT('Ctrl Pts',(-3.33829579765657,20.3325095899557,1.97677051430215));
#82839=CARTESIAN_POINT('Ctrl Pts',(-3.3662162259559,20.3920796795207,2.1333611225378));
#82840=CARTESIAN_POINT('Ctrl Pts',(-3.39413646367448,20.4516493624691,2.28995066190891));
#82841=CARTESIAN_POINT('Ctrl Pts',(-3.42205670139307,20.5177791268602,2.44403669680262));
#82842=CARTESIAN_POINT('Ctrl Pts',(-3.44997693911165,20.590231130146,2.59507240260436));
#82843=CARTESIAN_POINT('Ctrl Pts',(-3.47790319748545,20.6626987568135,2.74614067739491));
#82844=CARTESIAN_POINT('Ctrl Pts',(-3.50582945585924,20.7414912087847,2.89415702481168));
#82845=CARTESIAN_POINT('Ctrl Pts',(-3.53375571423304,20.8263237715149,3.03859742032546));
#82846=CARTESIAN_POINT('Ctrl Pts',(-3.54374939880251,20.8566819334211,3.09028682792646));
#82847=CARTESIAN_POINT('Ctrl Pts',(-3.55374308337198,20.8878131895755,3.14151852200135));
#82848=CARTESIAN_POINT('Ctrl Pts',(-3.56373676794145,20.9197030952441,3.19226931187323));
#82849=CARTESIAN_POINT('Ctrl Pts',(-3.59169420490673,21.0089154394363,3.33424517662241));
#82850=CARTESIAN_POINT('Ctrl Pts',(-3.61965164187199,21.104096867155,3.47250101481236));
#82851=CARTESIAN_POINT('Ctrl Pts',(-3.64760907883727,21.2049131331077,3.60654154820884));
#82852=CARTESIAN_POINT('Ctrl Pts',(-3.67556125585628,21.3057104313651,3.74055686305599));
#82853=CARTESIAN_POINT('Ctrl Pts',(-3.7035134328753,21.4121402635245,3.87035820492312));
#82854=CARTESIAN_POINT('Ctrl Pts',(-3.73146560989431,21.523826484711,3.99548128027463));
#82855=CARTESIAN_POINT('Ctrl Pts',(-3.75941702854489,21.6355096757468,4.12060096092133));
#82856=CARTESIAN_POINT('Ctrl Pts',(-3.78736844719548,21.7524487642828,4.24104239215249));
#82857=CARTESIAN_POINT('Ctrl Pts',(-3.81531986584607,21.8742284750283,4.35637570966201));
#82858=CARTESIAN_POINT('Ctrl Pts',(-3.8432691162056,21.9959987388882,4.47170008035548));
#82859=CARTESIAN_POINT('Ctrl Pts',(-3.87121836656512,22.1226086460514,4.58191691380431));
#82860=CARTESIAN_POINT('Ctrl Pts',(-3.89916761692465,22.2536071213404,4.6866342292448));
#82861=CARTESIAN_POINT('Ctrl Pts',(-3.92711978554461,22.3846192745514,4.79136247851691));
#82862=CARTESIAN_POINT('Ctrl Pts',(-3.95507195416456,22.5200206661178,4.89058986636883));
#82863=CARTESIAN_POINT('Ctrl Pts',(-3.98302412278452,22.6593277312072,4.98396516766709));
#82864=CARTESIAN_POINT('Ctrl Pts',(-3.9928613213411,22.7083540260272,5.0168267102415));
#82865=CARTESIAN_POINT('Ctrl Pts',(-4.00269851989769,22.7578637813317,5.04896382869954));
#82866=CARTESIAN_POINT('Ctrl Pts',(-4.01253571845427,22.8078350564425,5.08036248442202));
#82867=CARTESIAN_POINT('Ctrl Pts',(-4.04051728858883,22.9499766154631,5.16967487170139));
#82868=CARTESIAN_POINT('Ctrl Pts',(-4.06849885872339,23.0958819368552,5.25302648415614));
#82869=CARTESIAN_POINT('Ctrl Pts',(-4.09648042885795,23.2450325816891,5.3301176838833));
#82870=CARTESIAN_POINT('Ctrl Pts',(-4.12445918870059,23.3941682467756,5.40720114105794));
#82871=CARTESIAN_POINT('Ctrl Pts',(-4.15243794854322,23.546548306925,5.47802529729181));
#82872=CARTESIAN_POINT('Ctrl Pts',(-4.18041670838586,23.7016302440552,5.54233673327037));
#82873=CARTESIAN_POINT('Ctrl Pts',(-4.20839805871158,23.8567265398323,5.60665412368324));
#82874=CARTESIAN_POINT('Ctrl Pts',(-4.23637940903731,24.014524924548,5.66445746696233));
#82875=CARTESIAN_POINT('Ctrl Pts',(-4.26436075936304,24.1744627266629,5.71554141474429));
#82876=CARTESIAN_POINT('Ctrl Pts',(-4.29234180613671,24.3343987937134,5.76662480834867));
#82877=CARTESIAN_POINT('Ctrl Pts',(-4.32032285291038,24.4964739330904,5.81098885970217));
#82878=CARTESIAN_POINT('Ctrl Pts',(-4.34830389968406,24.6601098962103,5.84847796522877));
#82879=CARTESIAN_POINT('Ctrl Pts',(-4.3762903494129,24.8237774563529,5.88597430965383));
#82880=CARTESIAN_POINT('Ctrl Pts',(-4.40427679914175,24.9890061374045,5.91659298696035));
#82881=CARTESIAN_POINT('Ctrl Pts',(-4.4322632488706,25.1552062891796,5.94022925367014));
#82882=CARTESIAN_POINT('Ctrl Pts',(-4.4419537222361,25.212754072472,5.94841345049504));
#82883=CARTESIAN_POINT('Ctrl Pts',(-4.4516441956016,25.2704182524461,5.95576095638831));
#82884=CARTESIAN_POINT('Ctrl Pts',(-4.4613346689671,25.3281741450144,5.96226886516979));
#82885=CARTESIAN_POINT('Ctrl Pts',(-4.48921116242423,25.4943199771698,5.98099010506423));
#82886=CARTESIAN_POINT('Ctrl Pts',(-4.51708765588136,25.6612774018721,5.9927654663902));
#82887=CARTESIAN_POINT('Ctrl Pts',(-4.54496414933848,25.8284541615509,5.99754716741027));
#82888=CARTESIAN_POINT('Ctrl Pts',(-4.57283527846951,25.9955987510912,6.00232794827861));
#82889=CARTESIAN_POINT('Ctrl Pts',(-4.60070640760054,26.1629622738299,6.00011774523284));
#82890=CARTESIAN_POINT('Ctrl Pts',(-4.62857753673157,26.3299505264023,5.99092085159927));
#82891=CARTESIAN_POINT('Ctrl Pts',(-4.65644846200135,26.4969375575519,5.98172402523568));
#82892=CARTESIAN_POINT('Ctrl Pts',(-4.68431938727114,26.663549006492,5.96554062434815));
#82893=CARTESIAN_POINT('Ctrl Pts',(-4.71219031254093,26.8291931592569,5.9424270045699));
#82894=CARTESIAN_POINT('Ctrl Pts',(-4.74005958580881,26.9948274937451,5.91931475481234));
#82895=CARTESIAN_POINT('Ctrl Pts',(-4.76792885907669,27.1594943320396,5.88927315229279));
#82896=CARTESIAN_POINT('Ctrl Pts',(-4.79579813234457,27.3226092857528,5.85241015968981));
#82897=CARTESIAN_POINT('Ctrl Pts',(-4.82367165738117,27.485749124473,5.81554154322584));
#82898=CARTESIAN_POINT('Ctrl Pts',(-4.85154518241778,27.6473362955952,5.77184952786816));
#82899=CARTESIAN_POINT('Ctrl Pts',(-4.87941870745439,27.8067980508674,5.72149288240244));
#82900=CARTESIAN_POINT('Ctrl Pts',(-4.8896570114629,27.8653704031646,5.70299623928142));
#82901=CARTESIAN_POINT('Ctrl Pts',(-4.89989531547142,27.9236561360343,5.68360090060498));
#82902=CARTESIAN_POINT('Ctrl Pts',(-4.91013361947993,27.9816273951573,5.66331641944561));
#82903=CARTESIAN_POINT('Ctrl Pts',(-4.93826693235807,28.1409236584338,5.60757772927263));
#82904=CARTESIAN_POINT('Ctrl Pts',(-4.96640024523622,28.2978802294315,5.5451092700294));
#82905=CARTESIAN_POINT('Ctrl Pts',(-4.99453355811436,28.4519337618254,5.47613192204322));
#82906=CARTESIAN_POINT('Ctrl Pts',(-5.02266340201436,28.6059682986485,5.40716307930892));
#82907=CARTESIAN_POINT('Ctrl Pts',(-5.05079324591437,28.7571002329714,5.33168707485302));
#82908=CARTESIAN_POINT('Ctrl Pts',(-5.07892308981437,28.9047873242932,5.24997243808246));
#82909=CARTESIAN_POINT('Ctrl Pts',(-5.10705308241398,29.0524751963166,5.16825736935306));
#82910=CARTESIAN_POINT('Ctrl Pts',(-5.1351830750136,29.196717920631,5.08030374801303));
#82911=CARTESIAN_POINT('Ctrl Pts',(-5.16331306761321,29.3369982602062,4.98642583534348));
#82912=CARTESIAN_POINT('Ctrl Pts',(-5.19144090509611,29.4772678525157,4.89255511492108));
#82913=CARTESIAN_POINT('Ctrl Pts',(-5.21956874257901,29.6135754134946,4.79276118064227));
#82914=CARTESIAN_POINT('Ctrl Pts',(-5.24769658006191,29.7454327494578,4.68740157435749));
#82915=CARTESIAN_POINT('Ctrl Pts',(-5.27582597008618,29.8772973634057,4.58203615265417));
#82916=CARTESIAN_POINT('Ctrl Pts',(-5.30395536011045,30.0047110228937,4.47110463550279));
#82917=CARTESIAN_POINT('Ctrl Pts',(-5.33208475013472,30.1272180741514,4.35500527765449));
#82918=CARTESIAN_POINT('Ctrl Pts',(-5.34103402342074,30.1661932911832,4.31806864728964));
#82919=CARTESIAN_POINT('Ctrl Pts',(-5.34998329670675,30.2046721361559,4.28060923808268));
#82920=CARTESIAN_POINT('Ctrl Pts',(-5.35893256999276,30.2426406871193,4.24264068711928));
#82921=CARTESIAN_POINT('Ctrl Pts',(-5.35893256999276,30.2426406871193,4.24264068711928));
#82922=CARTESIAN_POINT('Ctrl Pts',(-5.38685862009565,30.3611208835163,4.12416049072224));
#82923=CARTESIAN_POINT('Ctrl Pts',(-5.41478467019854,30.4746472224472,4.00070195778111));
#82924=CARTESIAN_POINT('Ctrl Pts',(-5.44271072030143,30.5828134533402,3.87270200917711));
#82925=CARTESIAN_POINT('Ctrl Pts',(-5.47063386003537,30.6909684114738,3.74471540034279));
#82926=CARTESIAN_POINT('Ctrl Pts',(-5.4985569997693,30.7937641733863,3.61218856132808));
#82927=CARTESIAN_POINT('Ctrl Pts',(-5.52648013950324,30.8908341729529,3.47559219309117));
#82928=CARTESIAN_POINT('Ctrl Pts',(-5.55440620480455,30.987914342752,3.33898151335911));
#82929=CARTESIAN_POINT('Ctrl Pts',(-5.58233227010586,31.0792673669068,3.19830070794058));
#82930=CARTESIAN_POINT('Ctrl Pts',(-5.61025833540717,31.1645690517271,3.05405083617519));
#82931=CARTESIAN_POINT('Ctrl Pts',(-5.6381844242778,31.2498708085412,2.90980084266435));
#82932=CARTESIAN_POINT('Ctrl Pts',(-5.66611051314844,31.3291210581777,2.76198204972899));
#82933=CARTESIAN_POINT('Ctrl Pts',(-5.69403660201908,31.4020406501665,2.61112175394955));
#82934=CARTESIAN_POINT('Ctrl Pts',(-5.7219689671916,31.4749766306075,2.46022755278642));
#82935=CARTESIAN_POINT('Ctrl Pts',(-5.74990133236411,31.5415789745469,2.30629076733826));
#82936=CARTESIAN_POINT('Ctrl Pts',(-5.77783369753662,31.6016155910704,2.14986110478715));
#82937=CARTESIAN_POINT('Ctrl Pts',(-5.78779963852627,31.623035953213,2.09404883194927));
#82938=CARTESIAN_POINT('Ctrl Pts',(-5.79776557951593,31.643620958814,2.03791940446808));
#82939=CARTESIAN_POINT('Ctrl Pts',(-5.80773152050558,31.6633615678493,1.98149836028398));
#82940=CARTESIAN_POINT('Ctrl Pts',(-5.83573207289206,31.7188252674645,1.82297640987132));
#82941=CARTESIAN_POINT('Ctrl Pts',(-5.86373262527855,31.7676366153877,1.66210293936009));
#82942=CARTESIAN_POINT('Ctrl Pts',(-5.89173317766504,31.8096169836266,1.49945006704371));
#82943=CARTESIAN_POINT('Ctrl Pts',(-5.91972901151066,31.8515902775021,1.33682460433745));
#82944=CARTESIAN_POINT('Ctrl Pts',(-5.94772484535629,31.8867348112181,1.17242064020356));
#82945=CARTESIAN_POINT('Ctrl Pts',(-5.97572067920192,31.9149223252641,1.00682366186531));
#82946=CARTESIAN_POINT('Ctrl Pts',(-6.00371615034491,31.9431094741242,0.841228828934126));
#82947=CARTESIAN_POINT('Ctrl Pts',(-6.03171162148791,31.9643397280031,0.674441319648803));
#82948=CARTESIAN_POINT('Ctrl Pts',(-6.0597070926309,31.9785361518375,0.507055698293729));
#82949=CARTESIAN_POINT('Ctrl Pts',(-6.08770050947458,31.9927315339425,0.33968235964562));
#82950=CARTESIAN_POINT('Ctrl Pts',(-6.11569392631826,31.9998940919681,0.171711307511174));
#82951=CARTESIAN_POINT('Ctrl Pts',(-6.14368734316193,31.9999988334699,0.00374143821752759));
#82952=CARTESIAN_POINT('Ctrl Pts',(-6.17168351621534,32.0001035852844,-0.164244969256905));
#82953=CARTESIAN_POINT('Ctrl Pts',(-6.19967968926875,31.9931491319286,-0.332229881703685));
#82954=CARTESIAN_POINT('Ctrl Pts',(-6.22767586232215,31.9791626015674,-0.499614435357538));
#82955=CARTESIAN_POINT('Ctrl Pts',(-6.23729406522091,31.9743574702873,-0.5571201021531));
#82956=CARTESIAN_POINT('Ctrl Pts',(-6.24691226811966,31.9687227983511,-0.61455493216058));
#82957=CARTESIAN_POINT('Ctrl Pts',(-6.25653047101842,31.9622611017402,-0.671894749700876));
#82958=CARTESIAN_POINT('Ctrl Pts',(-6.28445158780701,31.9435031500081,-0.838349102871839));
#82959=CARTESIAN_POINT('Ctrl Pts',(-6.3123727045956,31.9177681741016,-1.00403609077342));
#82960=CARTESIAN_POINT('Ctrl Pts',(-6.34029382138419,31.8851440935428,-1.16836595219074));
#82961=CARTESIAN_POINT('Ctrl Pts',(-6.3682117124807,31.8525237820036,-1.33267682878248));
#82962=CARTESIAN_POINT('Ctrl Pts',(-6.39612960357722,31.8130160159444,-1.49563058248121));
#82963=CARTESIAN_POINT('Ctrl Pts',(-6.42404749467373,31.7667598741885,-1.65664738355812));
#82964=CARTESIAN_POINT('Ctrl Pts',(-6.45196791391568,31.72049954364,-1.81767876574686));
#82965=CARTESIAN_POINT('Ctrl Pts',(-6.47988833315764,31.6674897009362,-1.97677254082257));
#82966=CARTESIAN_POINT('Ctrl Pts',(-6.50780875239959,31.6079195847332,-2.13336305657655));
#82967=CARTESIAN_POINT('Ctrl Pts',(-6.53572898439683,31.5483498680295,-2.28995252217631));
#82968=CARTESIAN_POINT('Ctrl Pts',(-6.56364921639407,31.4822200807533,-2.44403846815317));
#82969=CARTESIAN_POINT('Ctrl Pts',(-6.59156944839131,31.4097680690463,-2.59507407199231));
#82970=CARTESIAN_POINT('Ctrl Pts',(-6.61949570597962,31.3373004211442,-2.74614227150561));
#82971=CARTESIAN_POINT('Ctrl Pts',(-6.64742196356792,31.2585079601768,-2.89415852951629));
#82972=CARTESIAN_POINT('Ctrl Pts',(-6.67534822115623,31.173675404125,-3.03859882392392));
#82973=CARTESIAN_POINT('Ctrl Pts',(-6.68534195461456,31.1433170952435,-3.09028844966017));
#82974=CARTESIAN_POINT('Ctrl Pts',(-6.6953356880729,31.1121856865101,-3.14152035587315));
#82975=CARTESIAN_POINT('Ctrl Pts',(-6.70532942153124,31.0802956230202,-3.19227135167446));
#82976=CARTESIAN_POINT('Ctrl Pts',(-6.73371647244484,30.9897123730567,-3.33642879871208));
#82977=CARTESIAN_POINT('Ctrl Pts',(-6.76210352335846,30.8929805450667,-3.47674274232387));
#82978=CARTESIAN_POINT('Ctrl Pts',(-6.79049057427206,30.7904459474236,-3.61270364475314));
#82979=CARTESIAN_POINT('Ctrl Pts',(-6.81887149804735,30.6879334811271,-3.74863520101128));
#82980=CARTESIAN_POINT('Ctrl Pts',(-6.84725242182265,30.5796209213999,-3.88021535828063));
#82981=CARTESIAN_POINT('Ctrl Pts',(-6.87563334559794,30.4658959184947,-4.00696564062785));
#82982=CARTESIAN_POINT('Ctrl Pts',(-6.89366519576886,30.3936406166832,-4.08749656761606));
#82983=CARTESIAN_POINT('Ctrl Pts',(-6.91169704593979,30.3192013059224,-4.16607844315121));
#82984=CARTESIAN_POINT('Ctrl Pts',(-6.92972889611071,30.2426857292706,-4.24259564448975));
#82985=CARTESIAN_POINT('',(-7.20743739462351,30.2426406871193,4.24264068711929));
#82986=CARTESIAN_POINT('Ctrl Pts',(-8.77823372208692,30.2426826788146,-4.24259869500835));
#82987=CARTESIAN_POINT('Ctrl Pts',(-8.74985421405489,30.3631070225411,-4.12217196743755));
#82988=CARTESIAN_POINT('Ctrl Pts',(-8.72147470602285,30.4783864730919,-3.99662931378174));
#82989=CARTESIAN_POINT('Ctrl Pts',(-8.69309519799082,30.5881081168997,-3.86642779677049));
#82990=CARTESIAN_POINT('Ctrl Pts',(-8.66470714486868,30.6978627979726,-3.7361870759896));
#82991=CARTESIAN_POINT('Ctrl Pts',(-8.63631909174654,30.8020561403102,-3.60128491292457));
#82992=CARTESIAN_POINT('Ctrl Pts',(-8.6079310386244,30.9003152694159,-3.46221175844709));
#82993=CARTESIAN_POINT('Ctrl Pts',(-8.58989877447026,30.9627300663717,-3.37387164412164));
#82994=CARTESIAN_POINT('Ctrl Pts',(-8.57186651031613,31.0227513077197,-3.28384924170612));
#82995=CARTESIAN_POINT('Ctrl Pts',(-8.55383424616199,31.080292384334,-3.19227650583059));
#82996=CARTESIAN_POINT('Ctrl Pts',(-8.52590799899587,31.1694052275134,-3.0504594364998));
#82997=CARTESIAN_POINT('Ctrl Pts',(-8.49798175182974,31.2525908867869,-2.90488517280906));
#82998=CARTESIAN_POINT('Ctrl Pts',(-8.47005550466362,31.3295484618057,-2.75606843043945));
#82999=CARTESIAN_POINT('Ctrl Pts',(-8.44213472535204,31.4064909688196,-2.60728082583033));
#83000=CARTESIAN_POINT('Ctrl Pts',(-8.41421394604047,31.4772076801296,-2.4552522895582));
#83001=CARTESIAN_POINT('Ctrl Pts',(-8.38629316672889,31.5414437738368,-2.3005218758806));
#83002=CARTESIAN_POINT('Ctrl Pts',(-8.35837317440489,31.6056780569567,-2.14579582350367));
#83003=CARTESIAN_POINT('Ctrl Pts',(-8.33045318208088,31.6634319632521,-1.98836833591238));
#83004=CARTESIAN_POINT('Ctrl Pts',(-8.30253318975688,31.714498658686,-1.82879880792706));
#83005=CARTESIAN_POINT('Ctrl Pts',(-8.27461530435817,31.765561500476,-1.66924132153077));
#83006=CARTESIAN_POINT('Ctrl Pts',(-8.24669741895945,31.8099380444609,-1.50754241849642));
#83007=CARTESIAN_POINT('Ctrl Pts',(-8.21877953356073,31.8474711189296,-1.34427732008116));
#83008=CARTESIAN_POINT('Ctrl Pts',(-8.19085841304085,31.8850085427264,-1.18099330252613));
#83009=CARTESIAN_POINT('Ctrl Pts',(-8.16293729252096,31.9157008419118,-1.01614303450835));
#83010=CARTESIAN_POINT('Ctrl Pts',(-8.13501617200108,31.9394416607826,-0.850313329402882));
#83011=CARTESIAN_POINT('Ctrl Pts',(-8.12502254655044,31.9479390579955,-0.790958979342547));
#83012=CARTESIAN_POINT('Ctrl Pts',(-8.11502892109981,31.9555463845614,-0.731479237943481));
#83013=CARTESIAN_POINT('Ctrl Pts',(-8.10503529564917,31.9622603691794,-0.671901250268776));
#83014=CARTESIAN_POINT('Ctrl Pts',(-8.07703903409974,31.981069005778,-0.504998764902671));
#83015=CARTESIAN_POINT('Ctrl Pts',(-8.04904277255031,31.9928668345532,-0.337290946922631));
#83016=CARTESIAN_POINT('Ctrl Pts',(-8.02104651100088,31.9976088514911,-0.169375513328665));
#83017=CARTESIAN_POINT('Ctrl Pts',(-7.99305304819962,32.0023503943761,-0.00147686601206276));
#83018=CARTESIAN_POINT('Ctrl Pts',(-7.96505958539836,32.0000375248769,0.166629043762389));
#83019=CARTESIAN_POINT('Ctrl Pts',(-7.93706612259709,31.990677328194,0.334342862137911));
#83020=CARTESIAN_POINT('Ctrl Pts',(-7.90907018876753,31.9813163052714,0.502071484883777));
#83021=CARTESIAN_POINT('Ctrl Pts',(-7.88107425493798,31.9649067271477,0.66940763545621));
#83022=CARTESIAN_POINT('Ctrl Pts',(-7.85307832110842,31.9415077333789,0.835754661488181));
#83023=CARTESIAN_POINT('Ctrl Pts',(-7.82508279866994,31.9181090834506,1.0020992431051));
#83024=CARTESIAN_POINT('Ctrl Pts',(-7.79708727623145,31.8877212692587,1.16745442069838));
#83025=CARTESIAN_POINT('Ctrl Pts',(-7.76909175379297,31.8504550085453,1.33123108173894));
#83026=CARTESIAN_POINT('Ctrl Pts',(-7.74109109595693,31.8131819118435,1.49503778537888));
#83027=CARTESIAN_POINT('Ctrl Pts',(-7.7130904381209,31.7690279176645,1.65726508990603));
#83028=CARTESIAN_POINT('Ctrl Pts',(-7.68508978028486,31.7181545160358,1.81733566815265));
#83029=CARTESIAN_POINT('Ctrl Pts',(-7.67547196856869,31.7006802552133,1.87231754364606));
#83030=CARTESIAN_POINT('Ctrl Pts',(-7.66585415685251,31.6824136591051,1.9270450898491));
#83031=CARTESIAN_POINT('Ctrl Pts',(-7.65623634513634,31.6633626250509,1.98149533867154));
#83032=CARTESIAN_POINT('Ctrl Pts',(-7.62830462513129,31.6080352632026,2.13962788994163));
#83033=CARTESIAN_POINT('Ctrl Pts',(-7.60037290512624,31.5460713918224,2.29546841885858));
#83034=CARTESIAN_POINT('Ctrl Pts',(-7.57244118512119,31.4776857840826,2.44846042460541));
#83035=CARTESIAN_POINT('Ctrl Pts',(-7.54451511922803,31.4093140193814,2.6014214607622));
#83036=CARTESIAN_POINT('Ctrl Pts',(-7.51658905333486,31.3345232408874,2.75153483678904));
#83037=CARTESIAN_POINT('Ctrl Pts',(-7.4886629874417,31.2535759864111,2.89826488696343));
#83038=CARTESIAN_POINT('Ctrl Pts',(-7.46073804729851,31.1726319950643,3.04498902218538));
#83039=CARTESIAN_POINT('Ctrl Pts',(-7.43281310715533,31.0855321727043,3.18832982641012));
#83040=CARTESIAN_POINT('Ctrl Pts',(-7.40488816701215,30.9925848854212,3.32777645911853));
#83041=CARTESIAN_POINT('Ctrl Pts',(-7.37696554812668,30.8996453243716,3.46721150034027));
#83042=CARTESIAN_POINT('Ctrl Pts',(-7.34904292924121,30.8008594450044,3.60275275499733));
#83043=CARTESIAN_POINT('Ctrl Pts',(-7.32112031035573,30.6965789646336,3.73391832114218));
#83044=CARTESIAN_POINT('Ctrl Pts',(-7.29319481863296,30.5922877552959,3.86509738234394));
#83045=CARTESIAN_POINT('Ctrl Pts',(-7.26526932691019,30.4825010115459,3.99189960876678));
#83046=CARTESIAN_POINT('Ctrl Pts',(-7.23734383518741,30.3676112099624,4.1138755837544));
#83047=CARTESIAN_POINT('Ctrl Pts',(-7.22737502166611,30.3265979659038,4.15741844275942));
#83048=CARTESIAN_POINT('Ctrl Pts',(-7.21740620814481,30.2849347809671,4.20034659327151));
#83049=CARTESIAN_POINT('Ctrl Pts',(-7.20743739462351,30.2426406871193,4.24264068711928));
#83050=CARTESIAN_POINT('',(-4.06584469763847,21.7573593077119,-4.24264069228803));
#83051=CARTESIAN_POINT('Ctrl Pts',(-7.20743739462351,30.2426406871193,4.24264068711928));
#83052=CARTESIAN_POINT('Ctrl Pts',(-7.17930845867346,30.1232997189722,4.36198165526634));
#83053=CARTESIAN_POINT('Ctrl Pts',(-7.15117952272342,29.9989146447901,4.47628978445081));
#83054=CARTESIAN_POINT('Ctrl Pts',(-7.12305058677337,29.8699299871777,4.58515451150155));
#83055=CARTESIAN_POINT('Ctrl Pts',(-7.09492341999255,29.7409534420544,4.69401239150605));
#83056=CARTESIAN_POINT('Ctrl Pts',(-7.06679625321173,29.6073781246749,4.79742735642718));
#83057=CARTESIAN_POINT('Ctrl Pts',(-7.03866908643091,29.4696822109658,4.89502863678119));
#83058=CARTESIAN_POINT('Ctrl Pts',(-7.0105392613718,29.3319732837149,4.99263914136195));
#83059=CARTESIAN_POINT('Ctrl Pts',(-6.98240943631269,29.190143229949,5.08443468530025));
#83060=CARTESIAN_POINT('Ctrl Pts',(-6.95427961125358,29.0447004950714,5.17008693305169));
#83061=CARTESIAN_POINT('Ctrl Pts',(-6.92615048084451,28.8992613518196,5.25573706566954));
#83062=CARTESIAN_POINT('Ctrl Pts',(-6.89802135043545,28.7502099700108,5.33524405234749));
#83063=CARTESIAN_POINT('Ctrl Pts',(-6.86989222002639,28.5980810389268,5.40832459410204));
#83064=CARTESIAN_POINT('Ctrl Pts',(-6.84175943001676,28.4459323158652,5.48141464363687));
#83065=CARTESIAN_POINT('Ctrl Pts',(-6.81362664000713,28.2907055189682,5.5480764459443));
#83066=CARTESIAN_POINT('Ctrl Pts',(-6.7854938499975,28.1329577804145,5.60807374300387));
#83067=CARTESIAN_POINT('Ctrl Pts',(-6.77654204803523,28.0827627405679,5.62716477241705));
#83068=CARTESIAN_POINT('Ctrl Pts',(-6.76759024607297,28.0323126066951,5.64558138550073));
#83069=CARTESIAN_POINT('Ctrl Pts',(-6.7586384441107,27.9816257293069,5.66331700233609));
#83070=CARTESIAN_POINT('Ctrl Pts',(-6.73076458085901,27.8237983896352,5.71854165547708));
#83071=CARTESIAN_POINT('Ctrl Pts',(-6.70289071760731,27.6636390492527,5.76717233636074));
#83072=CARTESIAN_POINT('Ctrl Pts',(-6.67501685435562,27.5017149435815,5.80903195276322));
#83073=CARTESIAN_POINT('Ctrl Pts',(-6.64714703160113,27.3398143098593,5.85088550134291));
#83074=CARTESIAN_POINT('Ctrl Pts',(-6.61927720884665,27.1761497289779,5.88596986477678));
#83075=CARTESIAN_POINT('Ctrl Pts',(-6.59140738609216,27.0113017847623,5.91415832558926));
#83076=CARTESIAN_POINT('Ctrl Pts',(-6.56353581145049,26.8464434782633,5.9423485583184));
#83077=CARTESIAN_POINT('Ctrl Pts',(-6.53566423680882,26.6804019725943,5.96364196579702));
#83078=CARTESIAN_POINT('Ctrl Pts',(-6.50779266216716,26.5137669106297,5.97796316160799));
#83079=CARTESIAN_POINT('Ctrl Pts',(-6.47992160891878,26.3471349659057,5.99228408951247));
#83080=CARTESIAN_POINT('Ctrl Pts',(-6.45205055567041,26.1799098039722,5.99963304183077));
#83081=CARTESIAN_POINT('Ctrl Pts',(-6.42417950242203,26.0126852567424,5.99998659034014));
#83082=CARTESIAN_POINT('Ctrl Pts',(-6.39630255305344,25.8454253331661,6.00034021364268));
#83083=CARTESIAN_POINT('Ctrl Pts',(-6.36842560368486,25.6781663424463,5.99369547670465));
#83084=CARTESIAN_POINT('Ctrl Pts',(-6.34054865431628,25.5115019531542,5.98008107455308));
#83085=CARTESIAN_POINT('Ctrl Pts',(-6.33031226741014,25.4503029621989,5.97508188019804));
#83086=CARTESIAN_POINT('Ctrl Pts',(-6.32007588050399,25.3891841152585,5.96914343670092));
#83087=CARTESIAN_POINT('Ctrl Pts',(-6.30983949359785,25.3281746568008,5.96226892283763));
#83088=CARTESIAN_POINT('Ctrl Pts',(-6.28185310161256,25.1613741406751,5.9434739279385));
#83089=CARTESIAN_POINT('Ctrl Pts',(-6.25386670962727,24.995339043989,5.91767231717653));
#83090=CARTESIAN_POINT('Ctrl Pts',(-6.22588031764197,24.8306617702719,5.88495098573441));
#83091=CARTESIAN_POINT('Ctrl Pts',(-6.19789886854471,24.6660135814516,5.85223543345373));
#83092=CARTESIAN_POINT('Ctrl Pts',(-6.16991741944744,24.5027230435007,5.81260266048362));
#83093=CARTESIAN_POINT('Ctrl Pts',(-6.14193597035018,24.3413727800146,5.76619074824303));
#83094=CARTESIAN_POINT('Ctrl Pts',(-6.11395507996023,24.1800257382191,5.71977976271195));
#83095=CARTESIAN_POINT('Ctrl Pts',(-6.08597418957029,24.0206191947924,5.66658999169828));
#83096=CARTESIAN_POINT('Ctrl Pts',(-6.05799329918034,23.863721702701,5.60680970218266));
#83097=CARTESIAN_POINT('Ctrl Pts',(-6.03001453781447,23.706836148705,5.54703396125978));
#83098=CARTESIAN_POINT('Ctrl Pts',(-6.00203577644859,23.5524595563791,5.48066881599614));
#83099=CARTESIAN_POINT('Ctrl Pts',(-5.97405701508271,23.4011418616442,5.40795121804017));
#83100=CARTESIAN_POINT('Ctrl Pts',(-5.94607549652134,23.2498092551532,5.33522645405453));
#83101=CARTESIAN_POINT('Ctrl Pts',(-5.91809397795996,23.1015364303583,5.25614812199193));
#83102=CARTESIAN_POINT('Ctrl Pts',(-5.89011245939859,22.9568506906527,5.17100012386571));
#83103=CARTESIAN_POINT('Ctrl Pts',(-5.8804218206274,22.9067427154278,5.14151142795663));
#83104=CARTESIAN_POINT('Ctrl Pts',(-5.87073118185622,22.8570647534989,5.11129514189335));
#83105=CARTESIAN_POINT('Ctrl Pts',(-5.86104054308503,22.8078379774101,5.08036431976434));
#83106=CARTESIAN_POINT('Ctrl Pts',(-5.83308821337882,22.6658449562999,4.99114537778861));
#83107=CARTESIAN_POINT('Ctrl Pts',(-5.8051358836726,22.5275804084579,4.89596087443907));
#83108=CARTESIAN_POINT('Ctrl Pts',(-5.77718355396639,22.3935383858232,4.79514698684719));
#83109=CARTESIAN_POINT('Ctrl Pts',(-5.74923416624616,22.2595104711272,4.69434370992882));
#83110=CARTESIAN_POINT('Ctrl Pts',(-5.72128477852594,22.1297044453186,4.5879124202907));
#83111=CARTESIAN_POINT('Ctrl Pts',(-5.69333539080571,22.004583184726,4.47623105661738));
#83112=CARTESIAN_POINT('Ctrl Pts',(-5.66538333752667,21.8794499912037,4.36453904178971));
#83113=CARTESIAN_POINT('Ctrl Pts',(-5.63743128424762,21.7590026916137,4.2475961597402));
#83114=CARTESIAN_POINT('Ctrl Pts',(-5.60947923096859,21.6436696069346,4.12581937394926));
#83115=CARTESIAN_POINT('Ctrl Pts',(-5.5815273625192,21.528337284882,4.00404339339295));
#83116=CARTESIAN_POINT('Ctrl Pts',(-5.55357549406982,21.4181193239461,3.87743380304682));
#83117=CARTESIAN_POINT('Ctrl Pts',(-5.52562362562044,21.3134059826887,3.74644318212646));
#83118=CARTESIAN_POINT('Ctrl Pts',(-5.49766596098341,21.2086709277424,3.6154253985776));
#83119=CARTESIAN_POINT('Ctrl Pts',(-5.46970829634638,21.1094429684166,3.48002501533422));
#83120=CARTESIAN_POINT('Ctrl Pts',(-5.44175063170935,21.0160714821414,3.34072694617136));
#83121=CARTESIAN_POINT('Ctrl Pts',(-5.4319142853303,20.9832205880179,3.29171770037032));
#83122=CARTESIAN_POINT('Ctrl Pts',(-5.42207793895126,20.9510942486745,3.24222625381832));
#83123=CARTESIAN_POINT('Ctrl Pts',(-5.4122415925722,20.9197064041771,3.19227457782702));
#83124=CARTESIAN_POINT('Ctrl Pts',(-5.38431534913912,20.8305935819466,3.05045742236428));
#83125=CARTESIAN_POINT('Ctrl Pts',(-5.35638910570604,20.7474079569722,2.90488308404311));
#83126=CARTESIAN_POINT('Ctrl Pts',(-5.32846286227296,20.6704504265211,2.75606628073979));
#83127=CARTESIAN_POINT('Ctrl Pts',(-5.30054208319254,20.5935079544178,2.60727859655151));
#83128=CARTESIAN_POINT('Ctrl Pts',(-5.27262130411212,20.5227912898402,2.45524999358071));
#83129=CARTESIAN_POINT('Ctrl Pts',(-5.2447005250317,20.4585552514206,2.30051952794176));
#83130=CARTESIAN_POINT('Ctrl Pts',(-5.21678052781217,20.3943210117919,2.14579339519407));
#83131=CARTESIAN_POINT('Ctrl Pts',(-5.18886053059263,20.3365671599187,1.98836584097777));
#83132=CARTESIAN_POINT('Ctrl Pts',(-5.1609405333731,20.2855005264566,1.82879626171768));
#83133=CARTESIAN_POINT('Ctrl Pts',(-5.13302264012483,20.2344377412302,1.66923870716541));
#83134=CARTESIAN_POINT('Ctrl Pts',(-5.10510474687656,20.1900612627682,1.50753975087095));
#83135=CARTESIAN_POINT('Ctrl Pts',(-5.07718685362829,20.1525282592692,1.34427461530531));
#83136=CARTESIAN_POINT('Ctrl Pts',(-5.04926572100557,20.1149909007333,1.18099053572748));
#83137=CARTESIAN_POINT('Ctrl Pts',(-5.02134458838285,20.0842986743378,1.01614022132391));
#83138=CARTESIAN_POINT('Ctrl Pts',(-4.99342345576012,20.0605579321982,0.85031048636718));
#83139=CARTESIAN_POINT('Ctrl Pts',(-4.98342985119321,20.0520605838895,0.790956275383463));
#83140=CARTESIAN_POINT('Ctrl Pts',(-4.97343624662629,20.0444533022396,0.731476675806575));
#83141=CARTESIAN_POINT('Ctrl Pts',(-4.96344264205937,20.0377393583589,0.67189883251683));
#83142=CARTESIAN_POINT('Ctrl Pts',(-4.93544641569036,20.0189308202128,0.504996612587124));
#83143=CARTESIAN_POINT('Ctrl Pts',(-4.90745018932134,20.0071330673888,0.337289066390713));
#83144=CARTESIAN_POINT('Ctrl Pts',(-4.87945396295232,20.0023911032032,0.169373909041591));
#83145=CARTESIAN_POINT('Ctrl Pts',(-4.85146053479445,19.997649612975,0.00147553474236162));
#83146=CARTESIAN_POINT('Ctrl Pts',(-4.82346710663657,19.9999625122051,-0.166630097560031));
#83147=CARTESIAN_POINT('Ctrl Pts',(-4.79547367847869,20.0093227149932,-0.334343635955789));
#83148=CARTESIAN_POINT('Ctrl Pts',(-4.76747777806289,20.0186837444339,-0.502071986082449));
#83149=CARTESIAN_POINT('Ctrl Pts',(-4.73948187764708,20.0350933060655,-0.669407861490774));
#83150=CARTESIAN_POINT('Ctrl Pts',(-4.71148597723127,20.0584922596335,-0.835754611811684));
#83151=CARTESIAN_POINT('Ctrl Pts',(-4.68349048736598,20.0818908700636,-1.00209892271317));
#83152=CARTESIAN_POINT('Ctrl Pts',(-4.65549499750069,20.1122786214671,-1.16745382898266));
#83153=CARTESIAN_POINT('Ctrl Pts',(-4.6274995076354,20.1495447954169,-1.33123022019737));
#83154=CARTESIAN_POINT('Ctrl Pts',(-4.59949888080676,20.1868178074314,-1.49503666315689));
#83155=CARTESIAN_POINT('Ctrl Pts',(-4.57149825397813,20.2309716937099,-1.65726370832291));
#83156=CARTESIAN_POINT('Ctrl Pts',(-4.5434976271495,20.2818449635609,-1.81733403072898));
#83157=CARTESIAN_POINT('Ctrl Pts',(-4.53387964861519,20.2993195015557,-1.87231683287499));
#83158=CARTESIAN_POINT('Ctrl Pts',(-4.52426167008086,20.3175864012626,-1.92704529676114));
#83159=CARTESIAN_POINT('Ctrl Pts',(-4.51464369154655,20.3366377648732,-1.98149645312302));
#83160=CARTESIAN_POINT('Ctrl Pts',(-4.48671174395061,20.3919655749844,-2.13963018575835));
#83161=CARTESIAN_POINT('Ctrl Pts',(-4.45877979635468,20.4539299931781,-2.29547185730847));
#83162=CARTESIAN_POINT('Ctrl Pts',(-4.43084784875875,20.5223162427038,-2.44846495891884));
#83163=CARTESIAN_POINT('Ctrl Pts',(-4.40292155618005,20.5906886469572,-2.60142708601074));
#83164=CARTESIAN_POINT('Ctrl Pts',(-4.37499526360135,20.6654801595467,-2.7515415064063));
#83165=CARTESIAN_POINT('Ctrl Pts',(-4.34706897102266,20.7464282390894,-2.89827254635629));
#83166=CARTESIAN_POINT('Ctrl Pts',(-4.31914380742579,20.8273730461278,-3.04499765438114));
#83167=CARTESIAN_POINT('Ctrl Pts',(-4.29121864382891,20.914473773728,-3.18833937760928));
#83168=CARTESIAN_POINT('Ctrl Pts',(-4.26329348023204,21.0074220522362,-3.3277868674996));
#83169=CARTESIAN_POINT('Ctrl Pts',(-4.23537064029043,21.1003625965102,-3.4672227539523));
#83170=CARTESIAN_POINT('Ctrl Pts',(-4.20744780034882,21.1991495440843,-3.60276479269939));
#83171=CARTESIAN_POINT('Ctrl Pts',(-4.17952496040721,21.3034311739776,-3.73393107360522));
#83172=CARTESIAN_POINT('Ctrl Pts',(-4.15159925266601,21.4077235140571,-3.86511082587024));
#83173=CARTESIAN_POINT('Ctrl Pts',(-4.12367354492482,21.5175114678987,-3.99191367560493));
#83174=CARTESIAN_POINT('Ctrl Pts',(-4.09574783718362,21.6324025551485,-4.11389019782085));
#83175=CARTESIAN_POINT('Ctrl Pts',(-4.08578013846699,21.6734113544078,-4.15742804600068));
#83176=CARTESIAN_POINT('Ctrl Pts',(-4.07581243975035,21.7150699487486,-4.20035132298714));
#83177=CARTESIAN_POINT('Ctrl Pts',(-4.06584474103372,21.7573593128807,-4.24264068711927));
#83178=CARTESIAN_POINT('Ctrl Pts',(-4.06584464821331,21.7573593128807,-4.24264068711927));
#83179=CARTESIAN_POINT('Ctrl Pts',(-4.03771516188517,21.8767026160842,-4.36198399032277));
#83180=CARTESIAN_POINT('Ctrl Pts',(-4.00958567555705,22.0010901908825,-4.47629422602707));
#83181=CARTESIAN_POINT('Ctrl Pts',(-3.98145618922891,22.1300774906703,-4.58516082289194));
#83182=CARTESIAN_POINT('Ctrl Pts',(-3.95332846351848,22.2590567171744,-4.69402060582301));
#83183=CARTESIAN_POINT('Ctrl Pts',(-3.92520073780805,22.3926348602974,-4.79743723369757));
#83184=CARTESIAN_POINT('Ctrl Pts',(-3.89707301209762,22.5303337208148,-4.89503992946789));
#83185=CARTESIAN_POINT('Ctrl Pts',(-3.86894262111681,22.6680456291235,-4.99265187367786));
#83186=CARTESIAN_POINT('Ctrl Pts',(-3.84081223013601,22.8098787870859,-5.08444860681414));
#83187=CARTESIAN_POINT('Ctrl Pts',(-3.8126818391552,22.9553247265007,-5.17010178612975));
#83188=CARTESIAN_POINT('Ctrl Pts',(-3.78455214045757,23.1007670865208,-5.25575285753813));
#83189=CARTESIAN_POINT('Ctrl Pts',(-3.75642244175993,23.2498217860661,-5.33526052436333));
#83190=CARTESIAN_POINT('Ctrl Pts',(-3.7282927430623,23.4019541134999,-5.40834148067964));
#83191=CARTESIAN_POINT('Ctrl Pts',(-3.70015938579756,23.5541062273644,-5.48143194195318));
#83192=CARTESIAN_POINT('Ctrl Pts',(-3.67202602853282,23.7093364934794,-5.54809389086397));
#83193=CARTESIAN_POINT('Ctrl Pts',(-3.64389267126808,23.8670877576044,-5.60809106258438));
#83194=CARTESIAN_POINT('Ctrl Pts',(-3.63494368007888,23.9172671464152,-5.62717567292969));
#83195=CARTESIAN_POINT('Ctrl Pts',(-3.62599468888967,23.9677014644956,-5.64558629009007));
#83196=CARTESIAN_POINT('Ctrl Pts',(-3.61704569770047,24.0183723790421,-5.66331634043665));
#83197=CARTESIAN_POINT('Ctrl Pts',(-3.58917226838873,24.1761971131281,-5.71854014103948));
#83198=CARTESIAN_POINT('Ctrl Pts',(-3.56129883907699,24.3363538428541,-5.76717021039578));
#83199=CARTESIAN_POINT('Ctrl Pts',(-3.53342540976525,24.4982753557587,-5.80902944500011));
#83200=CARTESIAN_POINT('Ctrl Pts',(-3.50555603581229,24.6601733103914,-5.85088258942398));
#83201=CARTESIAN_POINT('Ctrl Pts',(-3.47768666185932,24.8238352281641,-5.88596678558931));
#83202=CARTESIAN_POINT('Ctrl Pts',(-3.44981728790635,24.9886805465176,-5.91415530426856));
#83203=CARTESIAN_POINT('Ctrl Pts',(-3.42194618026319,25.1535361195224,-5.94234557649128));
#83204=CARTESIAN_POINT('Ctrl Pts',(-3.39407507262003,25.3195749273882,-5.96363925759899));
#83205=CARTESIAN_POINT('Ctrl Pts',(-3.36620396497687,25.4862073472971,-5.97796094918898));
#83206=CARTESIAN_POINT('Ctrl Pts',(-3.33833338825653,25.6528365929886,-5.99228236796194));
#83207=CARTESIAN_POINT('Ctrl Pts',(-3.31046281153618,25.8200591112097,-5.99963203804457));
#83208=CARTESIAN_POINT('Ctrl Pts',(-3.28259223481584,25.9872810886311,-5.99998651909265));
#83209=CARTESIAN_POINT('Ctrl Pts',(-3.25471577267068,26.1545383782883,-6.00034107499643));
#83210=CARTESIAN_POINT('Ctrl Pts',(-3.22683931052552,26.3217948090041,-5.99369749083168));
#83211=CARTESIAN_POINT('Ctrl Pts',(-3.19896284838036,26.4884567296998,-5.98008444950495));
#83212=CARTESIAN_POINT('Ctrl Pts',(-3.18872414798279,26.5496697152214,-5.9750845377185));
#83213=CARTESIAN_POINT('Ctrl Pts',(-3.17848544758522,26.6108025300056,-5.96914494737047));
#83214=CARTESIAN_POINT('Ctrl Pts',(-3.16824674718765,26.6718259090464,-5.96226885907822));
#83215=CARTESIAN_POINT('Ctrl Pts',(-3.14026030146104,26.838627106392,-5.94347377138838));
#83216=CARTESIAN_POINT('Ctrl Pts',(-3.11227385573443,27.0046628436322,-5.91767201436493));
#83217=CARTESIAN_POINT('Ctrl Pts',(-3.08428741000782,27.1693407138992,-5.8849504921297));
#83218=CARTESIAN_POINT('Ctrl Pts',(-3.05630589929474,27.333989545555,-5.8522347398717));
#83219=CARTESIAN_POINT('Ctrl Pts',(-3.02832438858165,27.4972806815948,-5.81260171851936));
#83220=CARTESIAN_POINT('Ctrl Pts',(-3.00034287786857,27.6586314959111,-5.76618951828429));
#83221=CARTESIAN_POINT('Ctrl Pts',(-2.97236191520299,27.8199791500009,-5.7197782270813));
#83222=CARTESIAN_POINT('Ctrl Pts',(-2.94438095253741,27.9793862569935,-5.66658810562624));
#83223=CARTESIAN_POINT('Ctrl Pts',(-2.91639998987183,28.1362842619755,-5.6068074295481));
#83224=CARTESIAN_POINT('Ctrl Pts',(-2.88842115033735,28.2931703618977,-5.54703128949018));
#83225=CARTESIAN_POINT('Ctrl Pts',(-2.86044231080287,28.447547448432,-5.48066570620433));
#83226=CARTESIAN_POINT('Ctrl Pts',(-2.83246347126839,28.5988655844751,-5.4079476397087));
#83227=CARTESIAN_POINT('Ctrl Pts',(-2.80448186676361,28.7501986743246,-5.33522238695025));
#83228=CARTESIAN_POINT('Ctrl Pts',(-2.77650026225883,28.8984719278766,-5.25614353206902));
#83229=CARTESIAN_POINT('Ctrl Pts',(-2.74851865775405,29.0431580411126,-5.1709949851853));
#83230=CARTESIAN_POINT('Ctrl Pts',(-2.73882837072764,29.0932641730091,-5.14150726016784));
#83231=CARTESIAN_POINT('Ctrl Pts',(-2.72913808370123,29.1429403188547,-5.1112919991724));
#83232=CARTESIAN_POINT('Ctrl Pts',(-2.71944779667482,29.1921653085973,-5.08036225505503));
#83233=CARTESIAN_POINT('Ctrl Pts',(-2.69135596545285,29.3348669747074,-4.99069791909505));
#83234=CARTESIAN_POINT('Ctrl Pts',(-2.66326413423087,29.4738017201919,-4.89500908884372));
#83235=CARTESIAN_POINT('Ctrl Pts',(-2.6351723030089,29.6084706716364,-4.79363530235036));
#83236=CARTESIAN_POINT('Ctrl Pts',(-2.60708243574623,29.7431302080898,-4.69226860311273));
#83237=CARTESIAN_POINT('Ctrl Pts',(-2.57899256848356,29.8735242993192,-4.5852179242781));
#83238=CARTESIAN_POINT('Ctrl Pts',(-2.55090270122089,29.9991851541301,-4.47286464170168));
#83239=CARTESIAN_POINT('Ctrl Pts',(-2.5322845748429,30.0824738950045,-4.39839623662062));
#83240=CARTESIAN_POINT('Ctrl Pts',(-2.51366644846492,30.1636839143914,-4.32159919483766));
#83241=CARTESIAN_POINT('Ctrl Pts',(-2.49504832208693,30.2426872863434,-4.24259408738332));
#83242=CARTESIAN_POINT('Origin',(-31.4159265358979,26.,7.7715611723761E-15));
#83243=CARTESIAN_POINT('',(5.63664190388931,30.2426838347204,-4.24259753907934));
#83244=CARTESIAN_POINT('',(3.78813707791307,30.2426869010466,-4.2425944726886));
#83245=CARTESIAN_POINT('',(-31.4159265358979,30.2426406871193,-4.24264068711928));
#83246=CARTESIAN_POINT('',(4.06584552699229,21.7573593180495,-4.24264068195053));
#83247=CARTESIAN_POINT('Ctrl Pts',(5.63664190388088,30.2426838346846,-4.24259753911516));
#83248=CARTESIAN_POINT('Ctrl Pts',(5.6085541904248,30.1234976659262,-4.36178613215216));
#83249=CARTESIAN_POINT('Ctrl Pts',(5.58046647696872,29.9992876476353,-4.47594753544482));
#83250=CARTESIAN_POINT('Ctrl Pts',(5.55237876351264,29.8704989412251,-4.58467424644055));
#83251=CARTESIAN_POINT('Ctrl Pts',(5.52428659397689,29.7416898026521,-4.69341820678932));
#83252=CARTESIAN_POINT('Ctrl Pts',(5.49619442444114,29.6083007588941,-4.79672555322897));
#83253=CARTESIAN_POINT('Ctrl Pts',(5.4681022549054,29.4708105808102,-4.894228633006));
#83254=CARTESIAN_POINT('Ctrl Pts',(5.4494823125889,29.3796798768698,-4.9588552443049));
#83255=CARTESIAN_POINT('Ctrl Pts',(5.43086237027242,29.2867481229324,-5.02093272423811));
#83256=CARTESIAN_POINT('Ctrl Pts',(5.41224242795593,29.1921620225893,-5.08036431976472));
#83257=CARTESIAN_POINT('Ctrl Pts',(5.38426093251302,29.0500208445595,-5.16967635366504));
#83258=CARTESIAN_POINT('Ctrl Pts',(5.35627943707011,28.9041159465853,-5.25302763668842));
#83259=CARTESIAN_POINT('Ctrl Pts',(5.3282979416272,28.7549657670488,-5.33011853736753));
#83260=CARTESIAN_POINT('Ctrl Pts',(5.30031925100227,28.6058305380751,-5.40720171058461));
#83261=CARTESIAN_POINT('Ctrl Pts',(5.27234056037734,28.4534509546491,-5.47802561079631));
#83262=CARTESIAN_POINT('Ctrl Pts',(5.2443618697524,28.2983695338176,-5.54233682538501));
#83263=CARTESIAN_POINT('Ctrl Pts',(5.21638057970836,28.1432737048206,-5.60665401494237));
#83264=CARTESIAN_POINT('Ctrl Pts',(5.18839928966432,27.9854758247472,-5.66445718784532));
#83265=CARTESIAN_POINT('Ctrl Pts',(5.16041799962029,27.8255385637381,-5.71554100259154));
#83266=CARTESIAN_POINT('Ctrl Pts',(5.13243700769939,27.6656030067604,-5.76662427307167));
#83267=CARTESIAN_POINT('Ctrl Pts',(5.10445601577849,27.5035284130956,-5.81098823603987));
#83268=CARTESIAN_POINT('Ctrl Pts',(5.07647502385759,27.3398930292745,-5.84847729499751));
#83269=CARTESIAN_POINT('Ctrl Pts',(5.0484886204334,27.1762259984904,-5.88597360431161));
#83270=CARTESIAN_POINT('Ctrl Pts',(5.02050221700923,27.010997879448,-5.91659228413978));
#83271=CARTESIAN_POINT('Ctrl Pts',(4.99251581358505,26.844798319737,-5.94022859820811));
#83272=CARTESIAN_POINT('Ctrl Pts',(4.98282503487107,26.7872488328984,-5.94841308285869));
#83273=CARTESIAN_POINT('Ctrl Pts',(4.97313425615709,26.7295829452508,-5.95576082645302));
#83274=CARTESIAN_POINT('Ctrl Pts',(4.96344347744311,26.671825343199,-5.96226892283763));
#83275=CARTESIAN_POINT('Ctrl Pts',(4.9355665537412,26.5056772643785,-5.98099040144252));
#83276=CARTESIAN_POINT('Ctrl Pts',(4.90768963003929,26.3387175535921,-5.99276581585045));
#83277=CARTESIAN_POINT('Ctrl Pts',(4.87981270633737,26.1715384837214,-5.99754737777056));
#83278=CARTESIAN_POINT('Ctrl Pts',(4.85194115438949,26.0043916284828,-6.00232801830583));
#83279=CARTESIAN_POINT('Ctrl Pts',(4.8240696024416,25.8370258160442,-6.00011748649615));
#83280=CARTESIAN_POINT('Ctrl Pts',(4.79619805049373,25.670035265695,-5.99092006908079));
#83281=CARTESIAN_POINT('Ctrl Pts',(4.76832671673624,25.5030460226191,-5.98172272366673));
#83282=CARTESIAN_POINT('Ctrl Pts',(4.74045538297876,25.3364323532721,-5.96553861588635));
#83283=CARTESIAN_POINT('Ctrl Pts',(4.71258404922128,25.170785987995,-5.9424240947861));
#83284=CARTESIAN_POINT('Ctrl Pts',(4.68471437664526,25.0051494955382,-5.91931095135276));
#83285=CARTESIAN_POINT('Ctrl Pts',(4.65684470406925,24.8404805065169,-5.88926826528848));
#83286=CARTESIAN_POINT('Ctrl Pts',(4.62897503149323,24.6773634267367,-5.85240399281066));
#83287=CARTESIAN_POINT('Ctrl Pts',(4.60110112330571,24.5142215565475,-5.81553411772893));
#83288=CARTESIAN_POINT('Ctrl Pts',(4.57322721511818,24.3526323768021,-5.77184065528646));
#83289=CARTESIAN_POINT('Ctrl Pts',(4.54535330693066,24.1931686540343,-5.72148236799133));
#83290=CARTESIAN_POINT('Ctrl Pts',(4.53511704693053,24.134608077747,-5.70298906886563));
#83291=CARTESIAN_POINT('Ctrl Pts',(4.52488078693041,24.0763340041334,-5.68359743145589));
#83292=CARTESIAN_POINT('Ctrl Pts',(4.51464452693028,24.0183742706934,-5.66331700233619));
#83293=CARTESIAN_POINT('Ctrl Pts',(4.4865117157702,23.8590807166286,-5.6075793127247));
#83294=CARTESIAN_POINT('Ctrl Pts',(4.45837890461014,23.7021267572523,-5.54511207805169));
#83295=CARTESIAN_POINT('Ctrl Pts',(4.43024609345007,23.5480757211417,-5.47613616802442));
#83296=CARTESIAN_POINT('Ctrl Pts',(4.4021167522165,23.3940436858259,-5.40716876554857));
#83297=CARTESIAN_POINT('Ctrl Pts',(4.37398741098292,23.242914137515,-5.33169441516217));
#83298=CARTESIAN_POINT('Ctrl Pts',(4.34585806974934,23.0952292992012,-5.24998163575655));
#83299=CARTESIAN_POINT('Ctrl Pts',(4.31772857627372,22.9475436615853,-5.16826841410376));
#83300=CARTESIAN_POINT('Ctrl Pts',(4.28959908279809,22.8033030395622,-5.080316841577));
#83301=CARTESIAN_POINT('Ctrl Pts',(4.26146958932246,22.6630246528152,-4.98644116903836));
#83302=CARTESIAN_POINT('Ctrl Pts',(4.23334224738877,22.5227569955479,-4.89257267677286));
#83303=CARTESIAN_POINT('Ctrl Pts',(4.20521490545508,22.3864512211851,-4.79278116046609));
#83304=CARTESIAN_POINT('Ctrl Pts',(4.17708756352139,22.2545955059214,-4.68742415146482));
#83305=CARTESIAN_POINT('Ctrl Pts',(4.1489586600171,22.1227324703069,-4.58206129326496));
#83306=CARTESIAN_POINT('Ctrl Pts',(4.1208297565128,21.9953202260986,-4.47113251538342));
#83307=CARTESIAN_POINT('Ctrl Pts',(4.0927008530085,21.8728144094322,-4.35503606196433));
#83308=CARTESIAN_POINT('Ctrl Pts',(4.08374909414482,21.8338280859864,-4.31808945806355));
#83309=CARTESIAN_POINT('Ctrl Pts',(4.07479733528114,21.795338409257,-4.28061978349561));
#83310=CARTESIAN_POINT('Ctrl Pts',(4.06584557641746,21.7573593128807,-4.24264068711927));
#83311=CARTESIAN_POINT('',(0.924252830007244,30.2426406871193,4.24264068711929));
#83312=CARTESIAN_POINT('Ctrl Pts',(4.06584548359704,21.7573593128807,-4.24264068711927));
#83313=CARTESIAN_POINT('Ctrl Pts',(4.03791880226835,21.6388764384194,-4.12415781265794));
#83314=CARTESIAN_POINT('Ctrl Pts',(4.00999212093965,21.5253476884487,-4.00069641994847));
#83315=CARTESIAN_POINT('Ctrl Pts',(3.98206543961095,21.4171793209539,-3.87269345852562));
#83316=CARTESIAN_POINT('Ctrl Pts',(3.9541416574735,21.3090221828915,-3.74470378565145));
#83317=CARTESIAN_POINT('Ctrl Pts',(3.92621787533605,21.206224519716,-3.61217372590949));
#83318=CARTESIAN_POINT('Ctrl Pts',(3.8982940931986,21.1091529040836,-3.47557400789661));
#83319=CARTESIAN_POINT('Ctrl Pts',(3.87036737455777,21.0120710802665,-3.33895992486932));
#83320=CARTESIAN_POINT('Ctrl Pts',(3.84244065591694,20.9207166917825,-3.19827558389406));
#83321=CARTESIAN_POINT('Ctrl Pts',(3.81451393727611,20.8354139383164,-3.05402207121422));
#83322=CARTESIAN_POINT('Ctrl Pts',(3.7865871902451,20.7501110981319,-2.90976841188688));
#83323=CARTESIAN_POINT('Ctrl Pts',(3.75866044321409,20.6708600628755,-2.76194584652404));
#83324=CARTESIAN_POINT('Ctrl Pts',(3.73073369618308,20.5979399885723,-2.61108169786646));
#83325=CARTESIAN_POINT('Ctrl Pts',(3.70280067048967,20.525003519931,-2.46018363100646));
#83326=CARTESIAN_POINT('Ctrl Pts',(3.67486764479626,20.4584009922193,-2.30624289886807));
#83327=CARTESIAN_POINT('Ctrl Pts',(3.64693461910284,20.3983645016636,-2.14980923427589));
#83328=CARTESIAN_POINT('Ctrl Pts',(3.6369719237633,20.3769516668628,-2.09401503001439));
#83329=CARTESIAN_POINT('Ctrl Pts',(3.62700922842375,20.3563736444569,-2.03790388561375));
#83330=CARTESIAN_POINT('Ctrl Pts',(3.6170465330842,20.336639465377,-1.98150131336679));
#83331=CARTESIAN_POINT('Ctrl Pts',(3.58904611033923,20.2811760252203,-1.82298036968697));
#83332=CARTESIAN_POINT('Ctrl Pts',(3.56104568759426,20.2323648472564,-1.6621079135492));
#83333=CARTESIAN_POINT('Ctrl Pts',(3.53304526484928,20.1903845618598,-1.49945605501576));
#83334=CARTESIAN_POINT('Ctrl Pts',(3.50504956423739,20.1484113562312,-1.33683162691539));
#83335=CARTESIAN_POINT('Ctrl Pts',(3.47705386362551,20.1132668219182,-1.1724286972628));
#83336=CARTESIAN_POINT('Ctrl Pts',(3.44905816301361,20.0850792209348,-1.00683274548563));
#83337=CARTESIAN_POINT('Ctrl Pts',(3.42106282883359,20.0568919888949,-0.841238961171053));
#83338=CARTESIAN_POINT('Ctrl Pts',(3.39306749465355,20.0356615636487,-0.674452492907592));
#83339=CARTESIAN_POINT('Ctrl Pts',(3.36507216047352,20.0214648828223,-0.507067897497593));
#83340=CARTESIAN_POINT('Ctrl Pts',(3.33707888229296,20.0072692446113,-0.339695594944594));
#83341=CARTESIAN_POINT('Ctrl Pts',(3.30908560411241,20.0001063440121,-0.171725563911534));
#83342=CARTESIAN_POINT('Ctrl Pts',(3.28109232593185,20.0000011760623,-0.00375669357035702));
#83343=CARTESIAN_POINT('Ctrl Pts',(3.25309629274952,19.9998959977622,0.164228707687036));
#83344=CARTESIAN_POINT('Ctrl Pts',(3.22510025956719,20.0068499401413,0.332212636062041));
#83345=CARTESIAN_POINT('Ctrl Pts',(3.19710422638486,20.0208358776276,0.499596234708716));
#83346=CARTESIAN_POINT('Ctrl Pts',(3.1874853451137,20.0256411681226,0.557105916585281));
#83347=CARTESIAN_POINT('Ctrl Pts',(3.17786646384254,20.031276114924,0.614544754401049));
#83348=CARTESIAN_POINT('Ctrl Pts',(3.16824758257138,20.0377382015578,0.671888567276623));
#83349=CARTESIAN_POINT('Ctrl Pts',(3.14032641770501,20.0564959948186,0.838343065282123));
#83350=CARTESIAN_POINT('Ctrl Pts',(3.11240525283864,20.0822308275213,1.00403023929455));
#83351=CARTESIAN_POINT('Ctrl Pts',(3.08448408797227,20.1148547894252,1.16836032560507));
#83352=CARTESIAN_POINT('Ctrl Pts',(3.05656615786135,20.1474749717396,1.33267137375424));
#83353=CARTESIAN_POINT('Ctrl Pts',(3.02864822775042,20.1869826286598,1.49562533866357));
#83354=CARTESIAN_POINT('Ctrl Pts',(3.0007302976395,20.2332386904674,1.65664238714261));
#83355=CARTESIAN_POINT('Ctrl Pts',(2.97280985307306,20.2794989183721,1.81767393777864));
#83356=CARTESIAN_POINT('Ctrl Pts',(2.94488940850663,20.3325086810178,1.9767679193988));
#83357=CARTESIAN_POINT('Ctrl Pts',(2.9169689639402,20.392078748676,2.13335867564475));
#83358=CARTESIAN_POINT('Ctrl Pts',(2.88904871462632,20.4516483997502,2.28994833682409));
#83359=CARTESIAN_POINT('Ctrl Pts',(2.86112846531243,20.517778149159,2.44403451376054));
#83360=CARTESIAN_POINT('Ctrl Pts',(2.83320821599856,20.5902301593064,2.59507037876083));
#83361=CARTESIAN_POINT('Ctrl Pts',(2.80528195296983,20.6626977748205,2.7461387752265));
#83362=CARTESIAN_POINT('Ctrl Pts',(2.77735568994111,20.7414902343532,2.89415526299696));
#83363=CARTESIAN_POINT('Ctrl Pts',(2.74942942691238,20.8263228280928,3.0385958140046));
#83364=CARTESIAN_POINT('Ctrl Pts',(2.73943582862777,20.8566807339251,3.09028482235108));
#83365=CARTESIAN_POINT('Ctrl Pts',(2.72944223034316,20.8878117233957,3.14151612715943));
#83366=CARTESIAN_POINT('Ctrl Pts',(2.71944863205855,20.9197013523565,3.19226653817505));
#83367=CARTESIAN_POINT('Ctrl Pts',(2.69149131753093,21.0089133020105,3.33424194710808));
#83368=CARTESIAN_POINT('Ctrl Pts',(2.66353400300332,21.1040942925657,3.47249735556752));
#83369=CARTESIAN_POINT('Ctrl Pts',(2.6355766884757,21.2049100802888,3.60653748932186));
#83370=CARTESIAN_POINT('Ctrl Pts',(2.60762463203012,21.3057069070462,3.74055241342958));
#83371=CARTESIAN_POINT('Ctrl Pts',(2.57967257558453,21.4121362273927,3.87035339407639));
#83372=CARTESIAN_POINT('Ctrl Pts',(2.55172051913895,21.5238218980808,3.99547614182584));
#83373=CARTESIAN_POINT('Ctrl Pts',(2.52376921738104,21.6355045533272,4.120595511341));
#83374=CARTESIAN_POINT('Ctrl Pts',(2.49581791562314,21.7524430687688,4.24103666382374));
#83375=CARTESIAN_POINT('Ctrl Pts',(2.46786661386523,21.8742221707881,4.35636973912725));
#83376=CARTESIAN_POINT('Ctrl Pts',(2.43991747800799,21.995991836344,4.47169387745935));
#83377=CARTESIAN_POINT('Ctrl Pts',(2.41196834215075,22.122601110396,4.58191051421212));
#83378=CARTESIAN_POINT('Ctrl Pts',(2.38401920629351,22.2535989196033,4.68662767294378));
#83379=CARTESIAN_POINT('Ctrl Pts',(2.35606714794483,22.3846104265499,4.79135578138786));
#83380=CARTESIAN_POINT('Ctrl Pts',(2.32811508959615,22.5200111402011,4.89058306673688));
#83381=CARTESIAN_POINT('Ctrl Pts',(2.30016303124748,22.6593174977051,4.98395830829879));
#83382=CARTESIAN_POINT('Ctrl Pts',(2.29032524801356,22.7083466508048,5.01682191263311));
#83383=CARTESIAN_POINT('Ctrl Pts',(2.28048746477965,22.7578593220079,5.04896100631227));
#83384=CARTESIAN_POINT('Ctrl Pts',(2.27064968154573,22.8078335665496,5.0803615482712));
#83385=CARTESIAN_POINT('Ctrl Pts',(2.24266806215881,22.9499753739736,5.1696741497736));
#83386=CARTESIAN_POINT('Ctrl Pts',(2.2146864427719,23.0958809689459,5.25302596012788));
#83387=CARTESIAN_POINT('Ctrl Pts',(2.18670482338498,23.2450319119771,5.33011733773052));
#83388=CARTESIAN_POINT('Ctrl Pts',(2.15872601735941,23.3941678588963,5.40720096431996));
#83389=CARTESIAN_POINT('Ctrl Pts',(2.13074721133383,23.5465482247839,5.47802527131766));
#83390=CARTESIAN_POINT('Ctrl Pts',(2.10276840530826,23.7016304907273,5.54233683556363));
#83391=CARTESIAN_POINT('Ctrl Pts',(2.07478701386981,23.8567270872209,5.60665434259165));
#83392=CARTESIAN_POINT('Ctrl Pts',(2.04680562243137,24.0145257947562,5.66445778234574));
#83393=CARTESIAN_POINT('Ctrl Pts',(2.01882423099292,24.1744639407621,5.71554180252599));
#83394=CARTESIAN_POINT('Ctrl Pts',(1.99084314620162,24.3344003340109,5.76662526287813));
#83395=CARTESIAN_POINT('Ctrl Pts',(1.96286206141032,24.4964758201881,5.81098935838593));
#83396=CARTESIAN_POINT('Ctrl Pts',(1.93488097661903,24.6601121493087,5.84847848141463));
#83397=CARTESIAN_POINT('Ctrl Pts',(1.90689449378863,24.8237800467303,5.88597483674879));
#83398=CARTESIAN_POINT('Ctrl Pts',(1.87890801095822,24.9890090837231,5.91659350071802));
#83399=CARTESIAN_POINT('Ctrl Pts',(1.85092152812782,25.155209608394,5.94022972571351));
#83400=CARTESIAN_POINT('Ctrl Pts',(1.84123126242951,25.2127562194855,5.94841372302747));
#83401=CARTESIAN_POINT('Ctrl Pts',(1.83154099673121,25.2704192240213,5.95576106384894));
#83402=CARTESIAN_POINT('Ctrl Pts',(1.8218507310329,25.3281739395001,5.96226884201251));
#83403=CARTESIAN_POINT('Ctrl Pts',(1.79397447623059,25.4943185236473,5.98098994708153));
#83404=CARTESIAN_POINT('Ctrl Pts',(1.76609822142828,25.6612746781566,5.99276527668448));
#83405=CARTESIAN_POINT('Ctrl Pts',(1.73822196662597,25.8284501539608,5.99754705278116));
#83406=CARTESIAN_POINT('Ctrl Pts',(1.71035107197587,25.9955934846291,6.00232790941977));
#83407=CARTESIAN_POINT('Ctrl Pts',(1.68248017732578,26.1629557348742,6.00011788683632));
#83408=CARTESIAN_POINT('Ctrl Pts',(1.65460928267568,26.3299427101814,5.99092128207325));
#83409=CARTESIAN_POINT('Ctrl Pts',(1.62673858385612,26.4969285121805,5.98172474192871));
#83410=CARTESIAN_POINT('Ctrl Pts',(1.59886788503655,26.6635387269724,5.96554173164701));
#83411=CARTESIAN_POINT('Ctrl Pts',(1.57099718621698,26.8291816496961,5.94242861057728));
#83412=CARTESIAN_POINT('Ctrl Pts',(1.54312813425875,26.994814784688,5.91931685524672));
#83413=CARTESIAN_POINT('Ctrl Pts',(1.51525908230051,27.1594804272277,5.88927585270319));
#83414=CARTESIAN_POINT('Ctrl Pts',(1.48739003034228,27.3225941986181,5.85241356927054));
#83415=CARTESIAN_POINT('Ctrl Pts',(1.45951671757968,27.485732907917,5.81554565008901));
#83416=CARTESIAN_POINT('Ctrl Pts',(1.43164340481709,27.6473189620354,5.77185443681084));
#83417=CARTESIAN_POINT('Ctrl Pts',(1.40377009205449,27.8067796228967,5.72149870176385));
#83418=CARTESIAN_POINT('Ctrl Pts',(1.39353065487635,27.8653585020267,5.70300020501307));
#83419=CARTESIAN_POINT('Ctrl Pts',(1.38329121769821,27.9236506969668,5.68360281467011));
#83420=CARTESIAN_POINT('Ctrl Pts',(1.37305178052007,27.9816283440733,5.66331608741429));
#83421=CARTESIAN_POINT('Ctrl Pts',(1.34491819503623,28.1409260732985,5.60757685433833));
#83422=CARTESIAN_POINT('Ctrl Pts',(1.3167846095524,28.2978840579134,5.54510773076915));
#83423=CARTESIAN_POINT('Ctrl Pts',(1.28865102406856,28.4519389419314,5.47612960265192));
#83424=CARTESIAN_POINT('Ctrl Pts',(1.26052090720747,28.605974832342,5.40715997892899));
#83425=CARTESIAN_POINT('Ctrl Pts',(1.23239079034638,28.7571080582065,5.33168307752366));
#83426=CARTESIAN_POINT('Ctrl Pts',(1.20426067348529,28.9047963694786,5.24996743340983));
#83427=CARTESIAN_POINT('Ctrl Pts',(1.17613041007705,29.0524854501504,5.16825136358875));
#83428=CARTESIAN_POINT('Ctrl Pts',(1.1480001466688,29.19672931206,5.08029663171104));
#83429=CARTESIAN_POINT('Ctrl Pts',(1.11986988326057,29.3370107087109,4.9864175045767));
#83430=CARTESIAN_POINT('Ctrl Pts',(1.0917417770414,29.4772813477841,4.89254557662939));
#83431=CARTESIAN_POINT('Ctrl Pts',(1.06361367082224,29.6135898756071,4.79275033176959));
#83432=CARTESIAN_POINT('Ctrl Pts',(1.03548556460307,29.7454480889377,4.68738931742103));
#83433=CARTESIAN_POINT('Ctrl Pts',(1.00735591092944,29.8773135563857,4.58202250668605));
#83434=CARTESIAN_POINT('Ctrl Pts',(0.979226257255812,30.0047279815099,4.47108950501795));
#83435=CARTESIAN_POINT('Ctrl Pts',(0.951096603582176,30.1272357008951,4.35498857280439));
#83436=CARTESIAN_POINT('Ctrl Pts',(0.942148679057198,30.1662048911846,4.3180573545683));
#83437=CARTESIAN_POINT('Ctrl Pts',(0.933200754532215,30.2046778584644,4.28060351577423));
#83438=CARTESIAN_POINT('Ctrl Pts',(0.924252830007237,30.2426406871193,4.24264068711928));
#83439=CARTESIAN_POINT('Ctrl Pts',(0.924252830007237,30.2426406871193,4.24264068711928));
#83440=CARTESIAN_POINT('Ctrl Pts',(0.89632614867855,30.3611235615806,4.12415781265799));
#83441=CARTESIAN_POINT('Ctrl Pts',(0.868399467349873,30.4746523115512,4.00069641994855));
#83442=CARTESIAN_POINT('Ctrl Pts',(0.840472786021184,30.582820679046,3.87269345852573));
#83443=CARTESIAN_POINT('Ctrl Pts',(0.812549003883679,30.6909778171086,3.74470378565134));
#83444=CARTESIAN_POINT('Ctrl Pts',(0.784625221746176,30.7937754802843,3.61217372590913));
#83445=CARTESIAN_POINT('Ctrl Pts',(0.756701439608673,30.8908470959168,3.475574007896));
#83446=CARTESIAN_POINT('Ctrl Pts',(0.728774720967817,30.987928919734,3.33895992486855));
#83447=CARTESIAN_POINT('Ctrl Pts',(0.70084800232696,31.0792833082181,3.19827558389312));
#83448=CARTESIAN_POINT('Ctrl Pts',(0.672921283686104,31.1645860616843,3.05402207121311));
#83449=CARTESIAN_POINT('Ctrl Pts',(0.644994536655131,31.2498889018687,2.90976841188593));
#83450=CARTESIAN_POINT('Ctrl Pts',(0.617067789624155,31.3291399371249,2.76194584652326));
#83451=CARTESIAN_POINT('Ctrl Pts',(0.58914104259318,31.402060011428,2.61108169786585));
#83452=CARTESIAN_POINT('Ctrl Pts',(0.561208016899777,31.4749964800692,2.46018363100591));
#83453=CARTESIAN_POINT('Ctrl Pts',(0.533274991206372,31.5415990077809,2.30624289886759));
#83454=CARTESIAN_POINT('Ctrl Pts',(0.505341965512969,31.6016354983365,2.14980923427548));
#83455=CARTESIAN_POINT('Ctrl Pts',(0.49537927017345,31.6230483331373,2.09401503001411));
#83456=CARTESIAN_POINT('Ctrl Pts',(0.485416574833935,31.6436263555431,2.03790388561361));
#83457=CARTESIAN_POINT('Ctrl Pts',(0.475453879494417,31.663360534623,1.98150131336679));
#83458=CARTESIAN_POINT('Ctrl Pts',(0.447453456749435,31.7188239747797,1.82298036968693));
#83459=CARTESIAN_POINT('Ctrl Pts',(0.419453034004449,31.7676351527436,1.66210791354913));
#83460=CARTESIAN_POINT('Ctrl Pts',(0.391452611259467,31.8096154381402,1.49945605501565));
#83461=CARTESIAN_POINT('Ctrl Pts',(0.363456910647587,31.8515886437689,1.33683162691534));
#83462=CARTESIAN_POINT('Ctrl Pts',(0.335461210035708,31.8867331780818,1.17242869726283));
#83463=CARTESIAN_POINT('Ctrl Pts',(0.307465509423828,31.9149207790652,1.00683274548574));
#83464=CARTESIAN_POINT('Ctrl Pts',(0.279470175243799,31.9431080111051,0.841238961171152));
#83465=CARTESIAN_POINT('Ctrl Pts',(0.251474841063771,31.9643384363513,0.674452492907679));
#83466=CARTESIAN_POINT('Ctrl Pts',(0.223479506883741,31.9785351171777,0.50706789749767));
#83467=CARTESIAN_POINT('Ctrl Pts',(0.195486228703238,31.9927307553886,0.339695594944983));
#83468=CARTESIAN_POINT('Ctrl Pts',(0.167492950522737,31.9998936559878,0.171725563912239));
#83469=CARTESIAN_POINT('Ctrl Pts',(0.139499672342232,31.9999988239377,0.00375669357137531));
#83470=CARTESIAN_POINT('Ctrl Pts',(0.111503639159925,32.0001040022378,-0.164228707685864));
#83471=CARTESIAN_POINT('Ctrl Pts',(0.0835076059776147,31.9931500598587,
-0.332212636060722));
#83472=CARTESIAN_POINT('Ctrl Pts',(0.0555115727953073,31.9791641223725,
-0.499596234707248));
#83473=CARTESIAN_POINT('Ctrl Pts',(0.045892691524066,31.9743588318775,-0.557105916584305));
#83474=CARTESIAN_POINT('Ctrl Pts',(0.0362738102528267,31.9687238850761,
-0.614544754400563));
#83475=CARTESIAN_POINT('Ctrl Pts',(0.0266549289815856,31.9622617984422,
-0.671888567276625));
#83476=CARTESIAN_POINT('Ctrl Pts',(-0.00126623588478278,31.9435040051814,
-0.838343065282101));
#83477=CARTESIAN_POINT('Ctrl Pts',(-0.0291874007511589,31.9177691724787,
-1.0040302392945));
#83478=CARTESIAN_POINT('Ctrl Pts',(-0.0571085656175256,31.8851452105749,
-1.168360325605));
#83479=CARTESIAN_POINT('Ctrl Pts',(-0.0850264957284651,31.8525250282604,
-1.33267137375427));
#83480=CARTESIAN_POINT('Ctrl Pts',(-0.112944425839412,31.8130173713401,
-1.4956253386637));
#83481=CARTESIAN_POINT('Ctrl Pts',(-0.14086235595035,31.7667613095326,-1.65664238714284));
#83482=CARTESIAN_POINT('Ctrl Pts',(-0.168782800516778,31.7205010816279,
-1.81767393777883));
#83483=CARTESIAN_POINT('Ctrl Pts',(-0.196703245083203,31.6674913189821,
-1.97676791939895));
#83484=CARTESIAN_POINT('Ctrl Pts',(-0.224623689649633,31.607921251324,-2.13335867564485));
#83485=CARTESIAN_POINT('Ctrl Pts',(-0.252543938963529,31.5483516002497,
-2.2899483368243));
#83486=CARTESIAN_POINT('Ctrl Pts',(-0.280464188277424,31.4822218508408,
-2.44403451376085));
#83487=CARTESIAN_POINT('Ctrl Pts',(-0.308384437591322,31.4097698406934,
-2.59507037876124));
#83488=CARTESIAN_POINT('Ctrl Pts',(-0.336310700620064,31.3373022251793,
-2.746138775227));
#83489=CARTESIAN_POINT('Ctrl Pts',(-0.364236963648801,31.2585097656465,
-2.89415526299755));
#83490=CARTESIAN_POINT('Ctrl Pts',(-0.392163226677543,31.1736771719068,
-3.03859581400527));
#83491=CARTESIAN_POINT('Ctrl Pts',(-0.402156824962108,31.1433192660746,
-3.09028482235153));
#83492=CARTESIAN_POINT('Ctrl Pts',(-0.412150423246673,31.1121882766042,
-3.14151612715966));
#83493=CARTESIAN_POINT('Ctrl Pts',(-0.422144021531238,31.0802986476434,
-3.19226653817506));
#83494=CARTESIAN_POINT('Ctrl Pts',(-0.450530238418072,30.989718068122,-3.33642003856181));
#83495=CARTESIAN_POINT('Ctrl Pts',(-0.478916455304906,30.8929892453202,
-3.47673026481364));
#83496=CARTESIAN_POINT('Ctrl Pts',(-0.507302672191738,30.7904579669258,
-3.61268770683503));
#83497=CARTESIAN_POINT('Ctrl Pts',(-0.535682769382887,30.6879487929289,
-3.74861583821688));
#83498=CARTESIAN_POINT('Ctrl Pts',(-0.564062866574028,30.5796398364838,
-3.88019282519102));
#83499=CARTESIAN_POINT('Ctrl Pts',(-0.592442963765176,30.4659187273337,
-4.00694021927577));
#83500=CARTESIAN_POINT('Ctrl Pts',(-0.610476474549829,30.3936571408251,
-4.08747907306331));
#83501=CARTESIAN_POINT('Ctrl Pts',(-0.628509985334481,30.3192111329926,
-4.16606851660056));
#83502=CARTESIAN_POINT('Ctrl Pts',(-0.646543496119133,30.2426884810913,
-4.24259289260889));
#83503=CARTESIAN_POINT('',(-0.924251994623517,30.2426406871193,4.24264068711929));
#83504=CARTESIAN_POINT('Ctrl Pts',(-2.49504832207809,30.2426872863809,-4.24259408734582));
#83505=CARTESIAN_POINT('Ctrl Pts',(-2.46667006335947,30.3631063921147,-4.12217233630957));
#83506=CARTESIAN_POINT('Ctrl Pts',(-2.43829180464085,30.4783810719969,-3.99663506167176));
#83507=CARTESIAN_POINT('Ctrl Pts',(-2.40991354592223,30.5880984395498,-3.86643928039754));
#83508=CARTESIAN_POINT('Ctrl Pts',(-2.38152675269319,30.6978488036309,-3.73620434389315));
#83509=CARTESIAN_POINT('Ctrl Pts',(-2.35313995946415,30.8020383276375,-3.60130832543165));
#83510=CARTESIAN_POINT('Ctrl Pts',(-2.32475316623511,30.9002941637225,-3.46224163064734));
#83511=CARTESIAN_POINT('Ctrl Pts',(-2.30671839287741,30.962718324161,-3.37388940636458));
#83512=CARTESIAN_POINT('Ctrl Pts',(-2.2886836195197,31.022748262084,-3.28385440346218));
#83513=CARTESIAN_POINT('Ctrl Pts',(-2.270648846162,31.0802973280948,-3.19226863815583));
#83514=CARTESIAN_POINT('Ctrl Pts',(-2.24272260406513,31.1694101280169,-3.05045115013736));
#83515=CARTESIAN_POINT('Ctrl Pts',(-2.21479636196826,31.2525956824996,-2.90487651342687));
#83516=CARTESIAN_POINT('Ctrl Pts',(-2.18687011987139,31.3295531040625,-2.75605945345486));
#83517=CARTESIAN_POINT('Ctrl Pts',(-2.15894933075943,31.4064954986247,-2.60727145207154));
#83518=CARTESIAN_POINT('Ctrl Pts',(-2.13102854164748,31.477212042224,-2.45524257097675));
#83519=CARTESIAN_POINT('Ctrl Pts',(-2.10310775253553,31.541447926615,-2.30051187273918));
#83520=CARTESIAN_POINT('Ctrl Pts',(-2.07518772874498,31.6056820502715,-2.14578541573972));
#83521=CARTESIAN_POINT('Ctrl Pts',(-2.04726770495442,31.6634357454588,-1.98835757959765));
#83522=CARTESIAN_POINT('Ctrl Pts',(-2.01934768116386,31.7145021922793,-1.82878776637276));
#83523=CARTESIAN_POINT('Ctrl Pts',(-1.99142975184323,31.7655648082602,-1.66922992355936));
#83524=CARTESIAN_POINT('Ctrl Pts',(-1.96351182252259,31.8099410829883,-1.50753072550295));
#83525=CARTESIAN_POINT('Ctrl Pts',(-1.93559389320195,31.8474738594471,-1.34426539904996));
#83526=CARTESIAN_POINT('Ctrl Pts',(-1.90767271091177,31.8850110091879,-1.18098104908242));
#83527=CARTESIAN_POINT('Ctrl Pts',(-1.8797515286216,31.9157029968264,-1.01613051365243));
#83528=CARTESIAN_POINT('Ctrl Pts',(-1.85183034633142,31.9394434816715,-0.850300610390311));
#83529=CARTESIAN_POINT('Ctrl Pts',(-1.84183686277067,31.9479406198857,-0.790947163429956));
#83530=CARTESIAN_POINT('Ctrl Pts',(-1.83184337920992,31.9555477137923,-0.731468338095572));
#83531=CARTESIAN_POINT('Ctrl Pts',(-1.82184989564917,31.9622614929435,-0.671891278231294));
#83532=CARTESIAN_POINT('Ctrl Pts',(-1.79385381433342,31.9810696999027,-0.504990096839036));
#83533=CARTESIAN_POINT('Ctrl Pts',(-1.76585773301767,31.9928672096575,-0.337283608813402));
#83534=CARTESIAN_POINT('Ctrl Pts',(-1.73786165170193,31.9976090206897,-0.169369521879895));
#83535=CARTESIAN_POINT('Ctrl Pts',(-1.70986836725733,32.0023503580043,-0.00147220993925742));
#83536=CARTESIAN_POINT('Ctrl Pts',(-1.68187508281275,32.0000373950918,0.166632347773044));
#83537=CARTESIAN_POINT('Ctrl Pts',(-1.65388179836815,31.9906772196565,0.334344806882151));
#83538=CARTESIAN_POINT('Ctrl Pts',(-1.62588603799567,31.9813162163397,0.50207209969018));
#83539=CARTESIAN_POINT('Ctrl Pts',(-1.59789027762319,31.9649067700317,0.669406912970671));
#83540=CARTESIAN_POINT('Ctrl Pts',(-1.56989451725071,31.9415080227897,0.83575260401952));
#83541=CARTESIAN_POINT('Ctrl Pts',(-1.54189916480914,31.9181096164948,1.00209587121748));
#83542=CARTESIAN_POINT('Ctrl Pts',(-1.51390381236757,31.8877221589244,1.16744973644604));
#83543=CARTESIAN_POINT('Ctrl Pts',(-1.485908459926,31.8504563702668,1.33122509727129));
#83544=CARTESIAN_POINT('Ctrl Pts',(-1.45790796537159,31.8131837367269,1.49503053992486));
#83545=CARTESIAN_POINT('Ctrl Pts',(-1.42990747081718,31.7690303178787,1.6572565948491));
#83546=CARTESIAN_POINT('Ctrl Pts',(-1.40190697626278,31.7181576061116,1.81732594535721));
#83547=CARTESIAN_POINT('Ctrl Pts',(-1.39228829922063,31.7006819081808,1.87231266653428));
#83548=CARTESIAN_POINT('Ctrl Pts',(-1.38266962217848,31.6824137366426,1.92704501227138));
#83549=CARTESIAN_POINT('Ctrl Pts',(-1.37305094513634,31.6633609912275,1.98150000833774));
#83550=CARTESIAN_POINT('Ctrl Pts',(-1.34511823087734,31.608031667746,2.13963774790754));
#83551=CARTESIAN_POINT('Ctrl Pts',(-1.31718551661833,31.5460654028897,2.29548329282442));
#83552=CARTESIAN_POINT('Ctrl Pts',(-1.28925280235933,31.4776769861386,2.4484801072354));
#83553=CARTESIAN_POINT('Ctrl Pts',(-1.26132574550914,31.4093024205739,2.60144593412696));
#83554=CARTESIAN_POINT('Ctrl Pts',(-1.23339868865894,31.3345084272542,2.75156389430813));
#83555=CARTESIAN_POINT('Ctrl Pts',(-1.20547163180875,31.253557560246,2.89829828713029));
#83556=CARTESIAN_POINT('Ctrl Pts',(-1.17754571388895,31.1726099946025,3.04502669578233));
#83557=CARTESIAN_POINT('Ctrl Pts',(-1.14961979596914,31.0855062060404,3.18837153517099));
#83558=CARTESIAN_POINT('Ctrl Pts',(-1.12169387804934,30.9925545768458,3.32782192991391));
#83559=CARTESIAN_POINT('Ctrl Pts',(-1.09377029132843,30.8996107070644,3.46726068362119));
#83560=CARTESIAN_POINT('Ctrl Pts',(-1.06584670460752,30.8008201474129,3.60280538045999));
#83561=CARTESIAN_POINT('Ctrl Pts',(-1.03792311788661,30.6965346318148,3.73397408295295));
#83562=CARTESIAN_POINT('Ctrl Pts',(-1.00999667958778,30.5922384665005,3.86515618049359));
#83563=CARTESIAN_POINT('Ctrl Pts',(-0.98207024128895,30.4824464201251,3.99196114407935));
#83564=CARTESIAN_POINT('Ctrl Pts',(-0.954143802990121,30.3675509863158,
4.11393952093755));
#83565=CARTESIAN_POINT('Ctrl Pts',(-0.944179866867919,30.3265571885763,
4.15746045770362));
#83566=CARTESIAN_POINT('Ctrl Pts',(-0.934215930745716,30.2849140879152,
4.20036728632337));
#83567=CARTESIAN_POINT('Ctrl Pts',(-0.924251994623514,30.2426406871193,
4.24264068711928));
#83568=CARTESIAN_POINT('',(2.21734070236153,21.7573593077119,-4.24264069228803));
#83569=CARTESIAN_POINT('Ctrl Pts',(-0.924251994623514,30.2426406871193,
4.24264068711928));
#83570=CARTESIAN_POINT('Ctrl Pts',(-0.896122308120024,30.1232965346437,
4.3619848395949));
#83571=CARTESIAN_POINT('Ctrl Pts',(-0.867992621616533,29.998908050666,4.47629584114187));
#83572=CARTESIAN_POINT('Ctrl Pts',(-0.839862935113043,29.8699197905936,
4.58516311753156));
#83573=CARTESIAN_POINT('Ctrl Pts',(-0.811735005997595,29.7409395889981,
4.69402359249282));
#83574=CARTESIAN_POINT('Ctrl Pts',(-0.783607076882148,29.6073604186198,
4.79744082484517));
#83575=CARTESIAN_POINT('Ctrl Pts',(-0.7554791477667,29.4696604872218,4.89504403487973));
#83576=CARTESIAN_POINT('Ctrl Pts',(-0.727348550661214,29.3319474947114,
4.99265650277294));
#83577=CARTESIAN_POINT('Ctrl Pts',(-0.699217953555737,29.1901132081159,
5.08445366825331));
#83578=CARTESIAN_POINT('Ctrl Pts',(-0.671087356450254,29.0446661039873,
5.17010718604854));
#83579=CARTESIAN_POINT('Ctrl Pts',(-0.642957450664213,28.8992225742731,
5.25575859887807));
#83580=CARTESIAN_POINT('Ctrl Pts',(-0.614827544878162,28.7501666686984,
5.33526651284798));
#83581=CARTESIAN_POINT('Ctrl Pts',(-0.586697639092119,28.5980331070789,
5.40834761960824));
#83582=CARTESIAN_POINT('Ctrl Pts',(-0.55856407496633,28.4458797602437,5.48143823068464));
#83583=CARTESIAN_POINT('Ctrl Pts',(-0.530430510840543,28.2906482330414,
5.54810023279348));
#83584=CARTESIAN_POINT('Ctrl Pts',(-0.502296946714754,28.132895687777,5.60809735873605));
#83585=CARTESIAN_POINT('Ctrl Pts',(-0.493348979180065,28.0827220003185,
5.62717963116725));
#83586=CARTESIAN_POINT('Ctrl Pts',(-0.484401011645379,28.0322934436315,
5.64558806450506));
#83587=CARTESIAN_POINT('Ctrl Pts',(-0.47545304411069,27.9816283440737,5.66331608741415));
#83588=CARTESIAN_POINT('Ctrl Pts',(-0.447579776163769,27.8238045824141,
5.71853957037812));
#83589=CARTESIAN_POINT('Ctrl Pts',(-0.419706508216854,27.6636488268566,
5.76716941207883));
#83590=CARTESIAN_POINT('Ctrl Pts',(-0.391833240269932,27.501728281285,5.80902850476642));
#83591=CARTESIAN_POINT('Ctrl Pts',(-0.363964033260086,27.3398313263864,
5.85088149888166));
#83592=CARTESIAN_POINT('Ctrl Pts',(-0.336094826250237,27.1761704022288,
5.88596563316397));
#83593=CARTESIAN_POINT('Ctrl Pts',(-0.308225619240392,27.0113260634304,
5.9141541739649));
#83594=CARTESIAN_POINT('Ctrl Pts',(-0.280354685379861,26.8464715104353,
5.9423444614033));
#83595=CARTESIAN_POINT('Ctrl Pts',(-0.252483751519326,26.6804337091038,
5.96363824511411));
#83596=CARTESIAN_POINT('Ctrl Pts',(-0.224612817658794,26.5138022747661,
5.97796012218593));
#83597=CARTESIAN_POINT('Ctrl Pts',(-0.196742418305686,26.3471740360781,
5.99228172459349));
#83598=CARTESIAN_POINT('Ctrl Pts',(-0.168872018952584,26.1799525040583,
5.99963166297465));
#83599=CARTESIAN_POINT('Ctrl Pts',(-0.141001619599475,26.0127314851022,
5.9999864924254));
#83600=CARTESIAN_POINT('Ctrl Pts',(-0.113125338855247,25.84547517809,6.00034139675454));
#83601=CARTESIAN_POINT('Ctrl Pts',(-0.0852490581110152,25.6782197022789,
5.99369824315483));
#83602=CARTESIAN_POINT('Ctrl Pts',(-0.0573727773667869,25.5115587022245,
5.98008570997336));
#83603=CARTESIAN_POINT('Ctrl Pts',(-0.0471332161104769,25.4503405097852,
5.97508553191359));
#83604=CARTESIAN_POINT('Ctrl Pts',(-0.0368936548541687,25.3892024979934,
5.9691455154932));
#83605=CARTESIAN_POINT('Ctrl Pts',(-0.026654093597859,25.3281739395,5.9622688420125));
#83606=CARTESIAN_POINT('Ctrl Pts',(0.00133237775107972,25.16137245641,5.94347371783423));
#83607=CARTESIAN_POINT('Ctrl Pts',(0.0293188491000237,24.9953364493688,
5.91767190179122));
#83608=CARTESIAN_POINT('Ctrl Pts',(0.0573053204489611,24.830658326687,5.88495030149394));
#83609=CARTESIAN_POINT('Ctrl Pts',(0.0852868598251298,24.6660092247418,
5.85223446762714));
#83610=CARTESIAN_POINT('Ctrl Pts',(0.113268399201294,24.5027178360857,5.81260134412805));
#83611=CARTESIAN_POINT('Ctrl Pts',(0.141249938577463,24.3413667879488,5.76618902464018));
#83612=CARTESIAN_POINT('Ctrl Pts',(0.169230933987283,24.1800188765065,5.71977760741647));
#83613=CARTESIAN_POINT('Ctrl Pts',(0.197211929397112,24.0206115315198,5.66658734086016));
#83614=CARTESIAN_POINT('Ctrl Pts',(0.225192924806933,23.8637133088066,5.60680650397623));
#83615=CARTESIAN_POINT('Ctrl Pts',(0.253171799331124,23.7068269785648,5.54703019832201));
#83616=CARTESIAN_POINT('Ctrl Pts',(0.281150673855311,23.5524496823706,5.4806644326814));
#83617=CARTESIAN_POINT('Ctrl Pts',(0.309129548379502,23.4011313579394,5.40794617034175));
#83618=CARTESIAN_POINT('Ctrl Pts',(0.337111190803452,23.2497980638583,5.33522071411514));
#83619=CARTESIAN_POINT('Ctrl Pts',(0.365092833227402,23.1015246279873,5.25614164094682));
#83620=CARTESIAN_POINT('Ctrl Pts',(0.393074475651353,22.9568383547437,5.17099286412591));
#83621=CARTESIAN_POINT('Ctrl Pts',(0.402764602739227,22.9067330623395,5.14150558613592));
#83622=CARTESIAN_POINT('Ctrl Pts',(0.412454729827095,22.8570577432985,5.11129079675859));
#83623=CARTESIAN_POINT('Ctrl Pts',(0.422144856914969,22.807833566549,5.08036154827086));
#83624=CARTESIAN_POINT('Ctrl Pts',(0.45009688294762,22.6658420882681,4.99114340375536));
#83625=CARTESIAN_POINT('Ctrl Pts',(0.478048908980264,22.5275789742579,4.89595980073667));
#83626=CARTESIAN_POINT('Ctrl Pts',(0.506000935012917,22.3935382722901,4.79514690145816));
#83627=CARTESIAN_POINT('Ctrl Pts',(0.533950009814166,22.2595117226105,4.69434464620932));
#83628=CARTESIAN_POINT('Ctrl Pts',(0.561899084615418,22.1297069458922,4.58791446993937));
#83629=CARTESIAN_POINT('Ctrl Pts',(0.589848159416665,22.0045868150917,4.47623429702482));
#83630=CARTESIAN_POINT('Ctrl Pts',(0.617799888666578,21.8794548010727,4.36454351734464));
#83631=CARTESIAN_POINT('Ctrl Pts',(0.645751617916485,21.7590085579661,4.24760195201275));
#83632=CARTESIAN_POINT('Ctrl Pts',(0.673703347166398,21.6436764038817,4.12582655063237));
#83633=CARTESIAN_POINT('Ctrl Pts',(0.701654885842154,21.5283450361289,4.00405197951348));
#83634=CARTESIAN_POINT('Ctrl Pts',(0.729606424517915,21.4181279015186,3.87744386828778));
#83635=CARTESIAN_POINT('Ctrl Pts',(0.757557963193673,21.3134152563028,3.74645478287737));
#83636=CARTESIAN_POINT('Ctrl Pts',(0.785515291843235,21.2086809205647,3.61543856395628));
#83637=CARTESIAN_POINT('Ctrl Pts',(0.813472620492793,21.1094535477017,3.48003980368646));
#83638=CARTESIAN_POINT('Ctrl Pts',(0.841429949142356,21.0160825131925,3.34074340300097));
#83639=CARTESIAN_POINT('Ctrl Pts',(0.851267901904173,20.9832260182699,3.29172615149555));
#83640=CARTESIAN_POINT('Ctrl Pts',(0.86110585466598,20.9510943155683,3.24222653576395));
#83641=CARTESIAN_POINT('Ctrl Pts',(0.870943807427796,20.9197013523558,3.19226653817392));
#83642=CARTESIAN_POINT('Ctrl Pts',(0.898870053403839,20.8305885426266,3.05044890442022));
#83643=CARTESIAN_POINT('Ctrl Pts',(0.926796299379875,20.7474029982992,2.90487413347756));
#83644=CARTESIAN_POINT('Ctrl Pts',(0.954722545355917,20.6704456032832,2.75605695377225));
#83645=CARTESIAN_POINT('Ctrl Pts',(0.982643342595285,20.5935032235535,2.6072688100364));
#83646=CARTESIAN_POINT('Ctrl Pts',(1.01056413983465,20.5227867130616,2.45523980009785));
#83647=CARTESIAN_POINT('Ctrl Pts',(1.03848493707402,20.4585508762575,2.30050898910937));
#83648=CARTESIAN_POINT('Ctrl Pts',(1.06640497513163,20.3943167860609,2.14578238533637));
#83649=CARTESIAN_POINT('Ctrl Pts',(1.09432501318922,20.3365631416576,1.98835441732583));
#83650=CARTESIAN_POINT('Ctrl Pts',(1.12224505124682,20.285496759011,1.82878448941532));
#83651=CARTESIAN_POINT('Ctrl Pts',(1.15016299834979,20.2344342007678,1.6692265118281));
#83652=CARTESIAN_POINT('Ctrl Pts',(1.17808094545276,20.190057998844,1.50752719563975));
#83653=CARTESIAN_POINT('Ctrl Pts',(1.20599889255573,20.1525253061649,1.34426176950714));
#83654=CARTESIAN_POINT('Ctrl Pts',(1.23392009762376,20.1149882335004,1.18097729064647));
#83655=CARTESIAN_POINT('Ctrl Pts',(1.26184130269178,20.0842963363596,1.01612664422016));
#83656=CARTESIAN_POINT('Ctrl Pts',(1.28976250775981,20.0605559512525,0.850296649292306));
#83657=CARTESIAN_POINT('Ctrl Pts',(1.29975592448675,20.0520589124945,0.790943614883419));
#83658=CARTESIAN_POINT('Ctrl Pts',(1.30974934121368,20.0444519058687,0.73146520645205));
#83659=CARTESIAN_POINT('Ctrl Pts',(1.31974275794062,20.0377382015577,0.671888567275174));
#83660=CARTESIAN_POINT('Ctrl Pts',(1.34773877292647,20.0189301230358,0.504987843651186));
#83661=CARTESIAN_POINT('Ctrl Pts',(1.37573478791231,20.007132702851,0.337281820351));
#83662=CARTESIAN_POINT('Ctrl Pts',(1.40373080289816,20.0023909420332,0.169368201840285));
#83663=CARTESIAN_POINT('Ctrl Pts',(1.43172402135423,19.9976496548712,0.00147135626790321));
#83664=CARTESIAN_POINT('Ctrl Pts',(1.45971723981031,19.9999626287568,-0.166632731380683));
#83665=CARTESIAN_POINT('Ctrl Pts',(1.48771045826638,20.009322775496,-0.334344720024882));
#83666=CARTESIAN_POINT('Ctrl Pts',(1.51570615389444,20.0186837505319,-0.502071549814969));
#83667=CARTESIAN_POINT('Ctrl Pts',(1.5437018495225,20.0350931295111,-0.669405899637445));
#83668=CARTESIAN_POINT('Ctrl Pts',(1.57169754515055,20.0584917698864,-0.835751130117129));
#83669=CARTESIAN_POINT('Ctrl Pts',(1.59969283378329,20.0818900700973,-1.0020939423061));
#83670=CARTESIAN_POINT('Ctrl Pts',(1.627688122416,20.1122773825116,-1.16744735534482));
#83671=CARTESIAN_POINT('Ctrl Pts',(1.65568341104874,20.1495429864649,-1.33122227023831));
#83672=CARTESIAN_POINT('Ctrl Pts',(1.68368384374439,20.186815437878,-1.49502727835492));
#83673=CARTESIAN_POINT('Ctrl Pts',(1.71168427644005,20.2309686359984,-1.65725290477794));
#83674=CARTESIAN_POINT('Ctrl Pts',(1.7396847091357,20.2818410879826,-1.81732183636135));
#83675=CARTESIAN_POINT('Ctrl Pts',(1.74930370890828,20.2993173216317,-1.87231038004687));
#83676=CARTESIAN_POINT('Ctrl Pts',(1.75892270868087,20.3175860809654,-1.92704453122915));
#83677=CARTESIAN_POINT('Ctrl Pts',(1.76854170845345,20.3366394653772,-1.98150131336752));
#83678=CARTESIAN_POINT('Ctrl Pts',(1.79647472012914,20.3919693771996,-2.13964061758363));
#83679=CARTESIAN_POINT('Ctrl Pts',(1.82440773180482,20.4539363601836,-2.29548767417718));
#83680=CARTESIAN_POINT('Ctrl Pts',(1.85234074348051,20.5223256196587,-2.4484859368501));
#83681=CARTESIAN_POINT('Ctrl Pts',(1.88026809706484,20.5907010262531,-2.60145320830169));
#83682=CARTESIAN_POINT('Ctrl Pts',(1.90819545064917,20.6654959848677,-2.75157254979298));
#83683=CARTESIAN_POINT('Ctrl Pts',(1.9361228042335,20.7464479362731,-2.89830825029203));
#83684=CARTESIAN_POINT('Ctrl Pts',(1.96404901537803,20.827396576132,-3.04503794819205));
#83685=CARTESIAN_POINT('Ctrl Pts',(1.99197522652255,20.9145015564675,-3.18838400406016));
#83686=CARTESIAN_POINT('Ctrl Pts',(2.01990143766708,21.0074544898585,-3.3278355321689));
#83687=CARTESIAN_POINT('Ctrl Pts',(2.04782531488487,21.1003996547292,-3.46727540564799));
#83688=CARTESIAN_POINT('Ctrl Pts',(2.07574919210266,21.1991916207523,-3.60282113992212));
#83689=CARTESIAN_POINT('Ctrl Pts',(2.10367306932045,21.3034786487632,-3.73399078699681));
#83690=CARTESIAN_POINT('Ctrl Pts',(2.131599792102,21.407776304073,-3.86517380082534));
#83691=CARTESIAN_POINT('Ctrl Pts',(2.15952651488354,21.5175699441395,-3.99197958972882));
#83692=CARTESIAN_POINT('Ctrl Pts',(2.18745323766509,21.6324670699787,-4.11395869026166));
#83693=CARTESIAN_POINT('Ctrl Pts',(2.19741571143215,21.6734550373473,-4.15747305457479));
#83694=CARTESIAN_POINT('Ctrl Pts',(2.20737818519921,21.7150921163322,-4.20037349057077));
#83695=CARTESIAN_POINT('Ctrl Pts',(2.21734065896628,21.7573593128807,-4.24264068711927));
#83696=CARTESIAN_POINT('Ctrl Pts',(2.2173407517867,21.7573593128807,-4.24264068711927));
#83697=CARTESIAN_POINT('Ctrl Pts',(2.24547017450468,21.8767023462092,-4.36198372044778));
#83698=CARTESIAN_POINT('Ctrl Pts',(2.27359959722266,22.0010896320607,-4.47629371275351));
#83699=CARTESIAN_POINT('Ctrl Pts',(2.30172901994065,22.1300766266187,-4.58516009362348));
#83700=CARTESIAN_POINT('Ctrl Pts',(2.3298566810282,22.25905554325,-4.69401965663829));
#83701=CARTESIAN_POINT('Ctrl Pts',(2.35798434211575,22.3926333598853,-4.79743609238731));
#83702=CARTESIAN_POINT('Ctrl Pts',(2.3861120032033,22.5303318800058,-4.89503862467868));
#83703=CARTESIAN_POINT('Ctrl Pts',(2.41424232871702,22.6680434437826,-4.99265040248606));
#83704=CARTESIAN_POINT('Ctrl Pts',(2.44237265423074,22.8098762430537,-5.08444699821573));
#83705=CARTESIAN_POINT('Ctrl Pts',(2.47050297974446,22.955321812265,-5.17010006993391));
#83706=CARTESIAN_POINT('Ctrl Pts',(2.4986326126804,23.100763800559,-5.25575103284557));
#83707=CARTESIAN_POINT('Ctrl Pts',(2.52676224561635,23.2498181167879,-5.33525862110907));
#83708=CARTESIAN_POINT('Ctrl Pts',(2.55489187855229,23.4019500519087,-5.40833952958048));
#83709=CARTESIAN_POINT('Ctrl Pts',(2.58302517014452,23.5541017739375,-5.48142994325679));
#83710=CARTESIAN_POINT('Ctrl Pts',(2.61115846173675,23.7093316392366,-5.54809187524892));
#83711=CARTESIAN_POINT('Ctrl Pts',(2.63929175332897,23.8670824961232,-5.60808906149463));
#83712=CARTESIAN_POINT('Ctrl Pts',(2.64824106965249,23.9172636956446,-5.62717441439312));
#83713=CARTESIAN_POINT('Ctrl Pts',(2.657190385976,23.9676998435017,-5.64558572516249));
#83714=CARTESIAN_POINT('Ctrl Pts',(2.66613970229952,24.018372604843,-5.66331641944571));
#83715=CARTESIAN_POINT('Ctrl Pts',(2.69401318247694,24.1761976450724,-5.71854032010687));
#83716=CARTESIAN_POINT('Ctrl Pts',(2.72188666265437,24.3363546815082,-5.76717046119709));
#83717=CARTESIAN_POINT('Ctrl Pts',(2.74976014283179,24.4982764989898,-5.80902974054304));
#83718=CARTESIAN_POINT('Ctrl Pts',(2.77762956940271,24.6601747683773,-5.85088293234464));
#83719=CARTESIAN_POINT('Ctrl Pts',(2.80549899597363,24.8238369989971,-5.88596714805142));
#83720=CARTESIAN_POINT('Ctrl Pts',(2.83336842254456,24.9886826257904,-5.91415565982344));
#83721=CARTESIAN_POINT('Ctrl Pts',(2.86123958495308,25.1535385199364,-5.94234592730716));
#83722=CARTESIAN_POINT('Ctrl Pts',(2.88911074736159,25.3195776447197,-5.9636395761651));
#83723=CARTESIAN_POINT('Ctrl Pts',(2.91698190977011,25.4862103749654,-5.97796120940967));
#83724=CARTESIAN_POINT('Ctrl Pts',(2.94485254238088,25.6528399377204,-5.99228257041697));
#83725=CARTESIAN_POINT('Ctrl Pts',(2.97272317499164,25.8200627664747,-5.99963215607798));
#83726=CARTESIAN_POINT('Ctrl Pts',(3.00059380760241,25.987285045716,-5.99998652747966));
#83727=CARTESIAN_POINT('Ctrl Pts',(3.02847032690278,26.1545426447746,-6.00034097372983));
#83728=CARTESIAN_POINT('Ctrl Pts',(3.05634684620316,26.3217993761771,-5.99369725404841));
#83729=CARTESIAN_POINT('Ctrl Pts',(3.08422336550353,26.4884615867904,-5.98008405277301));
#83730=CARTESIAN_POINT('Ctrl Pts',(3.09446179460647,26.5496729313316,-5.97508422497456));
#83731=CARTESIAN_POINT('Ctrl Pts',(3.10470022370941,26.6108041082623,-5.96914476897286));
#83732=CARTESIAN_POINT('Ctrl Pts',(3.11493865281235,26.6718258549855,-5.96226886516978));
#83733=CARTESIAN_POINT('Ctrl Pts',(3.14292509107457,26.8386269657956,-5.94347378876235));
#83734=CARTESIAN_POINT('Ctrl Pts',(3.17091152933679,27.0046626214334,-5.91767204983508));
#83735=CARTESIAN_POINT('Ctrl Pts',(3.19889796759901,27.1693404154645,-5.88495055142872));
#83736=CARTESIAN_POINT('Ctrl Pts',(3.2268794699022,27.3339891653265,-5.85223482410241));
#83737=CARTESIAN_POINT('Ctrl Pts',(3.2548609722054,27.4972802250278,-5.81260183387949));
#83738=CARTESIAN_POINT('Ctrl Pts',(3.28284247450859,27.6586309687947,-5.76618966990811));
#83739=CARTESIAN_POINT('Ctrl Pts',(3.31082342749156,27.8199785449967,-5.71977841707938));
#83740=CARTESIAN_POINT('Ctrl Pts',(3.33880438047452,27.9793855800658,-5.66658833974861));
#83741=CARTESIAN_POINT('Ctrl Pts',(3.36678533345749,28.1362835193544,-5.60680771249868));
#83742=CARTESIAN_POINT('Ctrl Pts',(3.39476416260806,28.2931695496517,-5.54703162276515));
#83743=CARTESIAN_POINT('Ctrl Pts',(3.42274299175863,28.4475465729151,-5.48066609483681));
#83744=CARTESIAN_POINT('Ctrl Pts',(3.4507218209092,28.5988646522158,-5.40794808771897));
#83745=CARTESIAN_POINT('Ctrl Pts',(3.47870341411161,28.7501976803556,-5.33522289672862));
#83746=CARTESIAN_POINT('Ctrl Pts',(3.50668500731404,28.8984708789272,-5.25614410805264));
#83747=CARTESIAN_POINT('Ctrl Pts',(3.53466660051646,29.0431569440202,-5.17099563082988));
#83748=CARTESIAN_POINT('Ctrl Pts',(3.54435693478603,29.0932633237662,-5.14150777426415));
#83749=CARTESIAN_POINT('Ctrl Pts',(3.5540472690556,29.1429397137401,-5.11129237445318));
#83750=CARTESIAN_POINT('Ctrl Pts',(3.56373760332517,29.1921649435568,-5.08036248442241));
#83751=CARTESIAN_POINT('Ctrl Pts',(3.59182937948356,29.3348663302056,-4.99069833835923));
#83752=CARTESIAN_POINT('Ctrl Pts',(3.61992115564195,29.4738008104779,-4.89500972265669));
#83753=CARTESIAN_POINT('Ctrl Pts',(3.64801293180034,29.6084695131929,-4.79363617438342));
#83754=CARTESIAN_POINT('Ctrl Pts',(3.67610274521235,29.7431288067304,-4.69226970898605));
#83755=CARTESIAN_POINT('Ctrl Pts',(3.70419255862436,29.8735226711554,-4.58521928717258));
#83756=CARTESIAN_POINT('Ctrl Pts',(3.73228237203637,29.999183317532,-4.47286628380213));
#83757=CARTESIAN_POINT('Ctrl Pts',(3.7509006073286,30.0824725671577,-4.39839748538549));
#83758=CARTESIAN_POINT('Ctrl Pts',(3.76951884262084,30.1636830710683,-4.32160002382929));
#83759=CARTESIAN_POINT('Ctrl Pts',(3.78813707791307,30.2426869010466,-4.2425944726886));
#83760=CARTESIAN_POINT('Origin',(-31.4159265358979,26.,7.7715611723761E-15));
#83761=CARTESIAN_POINT('',(11.9198273038894,30.2426793568795,-4.24260201700658));
#83762=CARTESIAN_POINT('',(10.0713224779131,30.2426823068249,-4.24259906700534));
#83763=CARTESIAN_POINT('',(-31.4159265358979,30.2426406871193,-4.24264068711928));
#83764=CARTESIAN_POINT('',(10.3490309269923,21.7573593180495,-4.24264068195052));
#83765=CARTESIAN_POINT('Ctrl Pts',(11.9198273038809,30.2426793568436,-4.24260201704246));
#83766=CARTESIAN_POINT('Ctrl Pts',(11.8917400717272,30.123495274846,-4.36178827168631));
#83767=CARTESIAN_POINT('Ctrl Pts',(11.8636528395734,29.999287505876,-4.47594754696579));
#83768=CARTESIAN_POINT('Ctrl Pts',(11.8355656074197,29.8705011892402,-4.58467234860792));
#83769=CARTESIAN_POINT('Ctrl Pts',(11.8074739290482,29.7416944856895,-4.69341436142083));
#83770=CARTESIAN_POINT('Ctrl Pts',(11.7793822506767,29.608308020656,-4.7967199828174));
#83771=CARTESIAN_POINT('Ctrl Pts',(11.7512905723051,29.470820543405,-4.89422156787753));
#83772=CARTESIAN_POINT('Ctrl Pts',(11.7326696575221,29.379685276805,-4.95885169366101));
#83773=CARTESIAN_POINT('Ctrl Pts',(11.714048742739,29.2867487626982,-5.02093243374107));
#83774=CARTESIAN_POINT('Ctrl Pts',(11.6954278279559,29.1921577294537,-5.08036701728221));
#83775=CARTESIAN_POINT('Ctrl Pts',(11.6674463996327,29.0500169029914,-5.16967866274384));
#83776=CARTESIAN_POINT('Ctrl Pts',(11.6394649713094,28.9041124055508,-5.25302957654197));
#83777=CARTESIAN_POINT('Ctrl Pts',(11.6114835429862,28.7549626758259,-5.3301201351195));
#83778=CARTESIAN_POINT('Ctrl Pts',(11.5835049124322,28.6058278590825,-5.40720298567047));
#83779=CARTESIAN_POINT('Ctrl Pts',(11.5555262818782,28.4534487355297,-5.47802658718929));
#83780=CARTESIAN_POINT('Ctrl Pts',(11.5275476513242,28.2983678218862,-5.54233753531108));
#83781=CARTESIAN_POINT('Ctrl Pts',(11.4995664100833,28.1432724376382,-5.60665448428929));
#83782=CARTESIAN_POINT('Ctrl Pts',(11.4715851688425,27.9854750474674,-5.66445744360215));
#83783=CARTESIAN_POINT('Ctrl Pts',(11.4436039276017,27.8255383207092,-5.71554108021472));
#83784=CARTESIAN_POINT('Ctrl Pts',(11.4156229776983,27.6656032591937,-5.76662418495037));
#83785=CARTESIAN_POINT('Ctrl Pts',(11.3876420277949,27.5035292043085,-5.8109880143795));
#83786=CARTESIAN_POINT('Ctrl Pts',(11.3596610778915,27.3398944009461,-5.84847698074578));
#83787=CARTESIAN_POINT('Ctrl Pts',(11.3316747059724,27.1762278892077,-5.88597321154614));
#83788=CARTESIAN_POINT('Ctrl Pts',(11.3036883340533,27.0110003297392,-5.91659184866189));
#83789=CARTESIAN_POINT('Ctrl Pts',(11.2757019621341,26.8448013678039,-5.94022816472201));
#83790=CARTESIAN_POINT('Ctrl Pts',(11.2660109339038,26.7872505414007,-5.94841287000865));
#83791=CARTESIAN_POINT('Ctrl Pts',(11.2563199056734,26.7295833125003,-5.9557607946252));
#83792=CARTESIAN_POINT('Ctrl Pts',(11.2466288774431,26.6718243693625,-5.96226903256894));
#83793=CARTESIAN_POINT('Ctrl Pts',(11.2187513961962,26.505673387662,-5.98099081078629));
#83794=CARTESIAN_POINT('Ctrl Pts',(11.1908739149493,26.3387107239503,-5.99276628493694));
#83795=CARTESIAN_POINT('Ctrl Pts',(11.1629964337025,26.1715286708957,-5.99754765842346));
#83796=CARTESIAN_POINT('Ctrl Pts',(11.1351243336815,26.0043788892069,-6.00232810895532));
#83797=CARTESIAN_POINT('Ctrl Pts',(11.1072522336605,25.8370101201943,-6.00011714374969));
#83798=CARTESIAN_POINT('Ctrl Pts',(11.0793801336396,25.6700166037108,-5.99091904119672));
#83799=CARTESIAN_POINT('Ctrl Pts',(11.0515082701352,25.5030245042977,-5.98172101669682));
#83800=CARTESIAN_POINT('Ctrl Pts',(11.0236364066307,25.3364079685368,-5.96553598726629));
#83801=CARTESIAN_POINT('Ctrl Pts',(10.9957645431263,25.1707587479012,-5.94242029360239));
#83802=CARTESIAN_POINT('Ctrl Pts',(10.9678943525553,25.005119469913,-5.91930598739562));
#83803=CARTESIAN_POINT('Ctrl Pts',(10.9400241619842,24.8404477055799,-5.88926189348273));
#83804=CARTESIAN_POINT('Ctrl Pts',(10.9121539714132,24.6773278831695,-5.8523959598919));
#83805=CARTESIAN_POINT('Ctrl Pts',(10.8842795659469,24.5141833916432,-5.81552445095176));
#83806=CARTESIAN_POINT('Ctrl Pts',(10.8564051604806,24.3525916209166,-5.77182911146859));
#83807=CARTESIAN_POINT('Ctrl Pts',(10.8285307550143,24.1931253610869,-5.72146869599517));
#83808=CARTESIAN_POINT('Ctrl Pts',(10.818297145653,24.134580061838,-5.70297973414616));
#83809=CARTESIAN_POINT('Ctrl Pts',(10.8080635362916,24.076321113965,-5.68359289742881));
#83810=CARTESIAN_POINT('Ctrl Pts',(10.7978299269303,24.0183763331579,-5.6633177240034));
#83811=CARTESIAN_POINT('Ctrl Pts',(10.7696977847909,23.8590864138009,-5.60758137130871));
#83812=CARTESIAN_POINT('Ctrl Pts',(10.7415656426516,23.702135956483,-5.54511577331444));
#83813=CARTESIAN_POINT('Ctrl Pts',(10.7134335005122,23.5480882661828,-5.47614178501336));
#83814=CARTESIAN_POINT('Ctrl Pts',(10.6853048301441,23.3940595868179,-5.40717630875183));
#83815=CARTESIAN_POINT('Ctrl Pts',(10.6571761597759,23.2429332378814,-5.33170417045805));
#83816=CARTESIAN_POINT('Ctrl Pts',(10.6290474894078,23.0952514191351,-5.24999387446911));
#83817=CARTESIAN_POINT('Ctrl Pts',(10.6009186628996,22.9475687806187,-5.16828312491282));
#83818=CARTESIAN_POINT('Ctrl Pts',(10.5727898363915,22.8033309788704,-5.08033429409392));
#83819=CARTESIAN_POINT('Ctrl Pts',(10.5446610098833,22.6630552105896,-4.98646161846521));
#83820=CARTESIAN_POINT('Ctrl Pts',(10.5165343306218,22.5227901504224,-4.89259610871617));
#83821=CARTESIAN_POINT('Ctrl Pts',(10.4884076513603,22.3864867726021,-4.79280782832261));
#83822=CARTESIAN_POINT('Ctrl Pts',(10.4602809720987,22.2546332301958,-4.68745429413948));
#83823=CARTESIAN_POINT('Ctrl Pts',(10.4321527198829,22.1227723140219,-4.58209486817321));
#83824=CARTESIAN_POINT('Ctrl Pts',(10.404024467667,21.9953619691791,-4.47116975696246));
#83825=CARTESIAN_POINT('Ctrl Pts',(10.3758962154512,21.872857808516,-4.35507719004761));
#83826=CARTESIAN_POINT('Ctrl Pts',(10.3669411357733,21.8338566465811,-4.31811726168941));
#83827=CARTESIAN_POINT('Ctrl Pts',(10.3579860560953,21.7953524982787,-4.28063387251726));
#83828=CARTESIAN_POINT('Ctrl Pts',(10.3490309764174,21.7573593128807,-4.24264068711927));
#83829=CARTESIAN_POINT('',(7.20743823000724,30.2426406871193,4.24264068711929));
#83830=CARTESIAN_POINT('Ctrl Pts',(10.349030883597,21.7573593128807,-4.24264068711927));
#83831=CARTESIAN_POINT('Ctrl Pts',(10.3211052174972,21.6388807456707,-4.12416211990928));
#83832=CARTESIAN_POINT('Ctrl Pts',(10.2931795513974,21.5253558725309,-4.00070532573603));
#83833=CARTESIAN_POINT('Ctrl Pts',(10.2652538852976,21.4171909397775,-3.87270720782532));
#83834=CARTESIAN_POINT('Ctrl Pts',(10.2373311367051,21.3090373074524,-3.74472246239618));
#83835=CARTESIAN_POINT('Ctrl Pts',(10.2094083881127,21.2062427009957,-3.61219758103455));
#83836=CARTESIAN_POINT('Ctrl Pts',(10.1814856395203,21.1091736828357,-3.47560324768711));
#83837=CARTESIAN_POINT('Ctrl Pts',(10.1535599725185,21.0120945192872,-3.33899463787312));
#83838=CARTESIAN_POINT('Ctrl Pts',(10.1256343055166,20.9207423243946,-3.19831598171024));
#83839=CARTESIAN_POINT('Ctrl Pts',(10.0977086385148,20.8354412884937,-3.05406832199351));
#83840=CARTESIAN_POINT('Ctrl Pts',(10.0697829511709,20.7501401904563,-2.90982055720133));
#83841=CARTESIAN_POINT('Ctrl Pts',(10.0418572638269,20.6708904178689,-2.76200405661509));
#83842=CARTESIAN_POINT('Ctrl Pts',(10.013931576483,20.5979711181347,-2.61114610075604));
#83843=CARTESIAN_POINT('Ctrl Pts',(9.98599961470421,20.5250354346536,-2.46025424963762));
#83844=CARTESIAN_POINT('Ctrl Pts',(9.95806765292542,20.4584332020016,-2.30631986222864));
#83845=CARTESIAN_POINT('Ctrl Pts',(9.93013569114663,20.3983965081866,-2.14989262999431));
#83846=CARTESIAN_POINT('Ctrl Pts',(9.92016777179247,20.376971556836,-2.09406933881071));
#83847=CARTESIAN_POINT('Ctrl Pts',(9.91019985243831,20.3563822938692,-2.03792876199266));
#83848=CARTESIAN_POINT('Ctrl Pts',(9.90023193308415,20.3366377648729,-1.98149645312239));
#83849=CARTESIAN_POINT('Ctrl Pts',(9.87223131619321,20.2811739341101,-1.82297395662084));
#83850=CARTESIAN_POINT('Ctrl Pts',(9.84423069930227,20.2323625038322,-1.66209993737829));
#83851=CARTESIAN_POINT('Ctrl Pts',(9.81623008241133,20.1903821004303,-1.49944651821894));
#83852=CARTESIAN_POINT('Ctrl Pts',(9.78823418181804,20.1484087680182,-1.33682049566804));
#83853=CARTESIAN_POINT('Ctrl Pts',(9.76023828122473,20.1132642440369,-1.1724159732874));
#83854=CARTESIAN_POINT('Ctrl Pts',(9.73224238063144,20.0850767863215,-1.00681844256419));
#83855=CARTESIAN_POINT('Ctrl Pts',(9.70424684027408,20.0568896913069,-0.841223042659437));
#83856=CARTESIAN_POINT('Ctrl Pts',(9.67625129991674,20.0356595390914,-0.674434972048046));
#83857=CARTESIAN_POINT('Ctrl Pts',(9.64825575955938,20.0214632630262,-0.507048799085849));
#83858=CARTESIAN_POINT('Ctrl Pts',(9.62026227232045,20.0072680280781,-0.33967490178013));
#83859=CARTESIAN_POINT('Ctrl Pts',(9.59226878508153,20.0001056639017,-0.171703300650773));
#83860=CARTESIAN_POINT('Ctrl Pts',(9.56427529784261,20.0000011612094,-0.00373289588396664));
#83861=CARTESIAN_POINT('Ctrl Pts',(9.53627905335459,19.999896648224,0.164254053311281));
#83862=CARTESIAN_POINT('Ctrl Pts',(9.50828280886656,20.006851385897,0.332239493958736));
#83863=CARTESIAN_POINT('Ctrl Pts',(9.48028656437853,20.0208382443311,0.499624558589952));
#83864=CARTESIAN_POINT('Ctrl Pts',(9.47066870377616,20.0256433050506,0.557128207668029));
#83865=CARTESIAN_POINT('Ctrl Pts',(9.46105084317377,20.0312778483098,0.61456102333078));
#83866=CARTESIAN_POINT('Ctrl Pts',(9.45143298257139,20.037739358359,0.671898832518114));
#83867=CARTESIAN_POINT('Ctrl Pts',(9.42351189031721,20.0564974196,0.83835313313213));
#83868=CARTESIAN_POINT('Ctrl Pts',(9.39559079806303,20.0822324985814,1.00404004116379));
#83869=CARTESIAN_POINT('Ctrl Pts',(9.36766970580884,20.1148566697071,1.16836979672944));
#83870=CARTESIAN_POINT('Ctrl Pts',(9.33975183339789,20.1474770786335,1.33268060188844));
#83871=CARTESIAN_POINT('Ctrl Pts',(9.31183396098695,20.1869849324514,1.49563425761114));
#83872=CARTESIAN_POINT('Ctrl Pts',(9.283916088576,20.233241146378,1.65665093612744));
#83873=CARTESIAN_POINT('Ctrl Pts',(9.25599567924702,20.2795015636414,1.81768224635024));
#83874=CARTESIAN_POINT('Ctrl Pts',(9.22807526991804,20.3325114817047,1.97677592365439));
#83875=CARTESIAN_POINT('Ctrl Pts',(9.20015486058906,20.3920816560673,2.1333663182358));
#83876=CARTESIAN_POINT('Ctrl Pts',(9.17223463338991,20.4516514418429,2.28995569134995));
#83877=CARTESIAN_POINT('Ctrl Pts',(9.14431440619078,20.5177812833871,2.44404152052552));
#83878=CARTESIAN_POINT('Ctrl Pts',(9.11639417899164,20.5902333289587,2.59507698631285));
#83879=CARTESIAN_POINT('Ctrl Pts',(9.08846791866522,20.6627010302915,2.74614508851758));
#83880=CARTESIAN_POINT('Ctrl Pts',(9.06054165833879,20.7414935276847,2.89416122631526));
#83881=CARTESIAN_POINT('Ctrl Pts',(9.03261539801237,20.8263260977992,3.03860138117629));
#83882=CARTESIAN_POINT('Ctrl Pts',(9.0226216093611,20.8566845763982,3.09029123737493));
#83883=CARTESIAN_POINT('Ctrl Pts',(9.01262782070982,20.8878161603781,3.14152336661647));
#83884=CARTESIAN_POINT('Ctrl Pts',(9.00263403205854,20.9197064041777,3.19227457782808));
#83885=CARTESIAN_POINT('Ctrl Pts',(8.97467638145488,21.0089194468914,3.33425122755296));
#83886=CARTESIAN_POINT('Ctrl Pts',(8.94671873085123,21.1041016465399,3.47250780419374));
#83887=CARTESIAN_POINT('Ctrl Pts',(8.91876108024757,21.2049187549211,3.60654902269362));
#83888=CARTESIAN_POINT('Ctrl Pts',(8.89080869264064,21.3057168845933,3.74056500808271));
#83889=CARTESIAN_POINT('Ctrl Pts',(8.86285630503372,21.412147617434,3.8703669680771));
#83890=CARTESIAN_POINT('Ctrl Pts',(8.8349039174268,21.5238348055542,3.99549060217045));
#83891=CARTESIAN_POINT('Ctrl Pts',(8.8069522943046,21.6355189390821,4.12061081419089));
#83892=CARTESIAN_POINT('Ctrl Pts',(8.77900067118241,21.752459034069,4.24105271946324));
#83893=CARTESIAN_POINT('Ctrl Pts',(8.75104904806022,21.8742398121431,4.35638644662011));
#83894=CARTESIAN_POINT('Ctrl Pts',(8.7230995972203,21.9960111259288,4.4717112105261));
#83895=CARTESIAN_POINT('Ctrl Pts',(8.69515014638039,22.1226221425189,4.58192837425858));
#83896=CARTESIAN_POINT('Ctrl Pts',(8.66720069554047,22.2536217833888,4.6866459497279));
#83897=CARTESIAN_POINT('Ctrl Pts',(8.63924833355655,22.3846350688493,4.7913744323146));
#83898=CARTESIAN_POINT('Ctrl Pts',(8.61129597157264,22.5200376465994,4.89060198602177));
#83899=CARTESIAN_POINT('Ctrl Pts',(8.58334360958872,22.6593459482259,4.9839773781956));
#83900=CARTESIAN_POINT('Ctrl Pts',(8.57350743357439,22.7083672429503,5.01683530960609));
#83901=CARTESIAN_POINT('Ctrl Pts',(8.56367125756006,22.7578718971903,5.04896896823911));
#83902=CARTESIAN_POINT('Ctrl Pts',(8.55383508154573,22.8078379774106,5.08036431976468));
#83903=CARTESIAN_POINT('Ctrl Pts',(8.52585358610291,22.9499791554399,5.16967635366472));
#83904=CARTESIAN_POINT('Ctrl Pts',(8.49787209066009,23.0958840534137,5.25302763668785));
#83905=CARTESIAN_POINT('Ctrl Pts',(8.46989059521728,23.2450342329497,5.33011853736677));
#83906=CARTESIAN_POINT('Ctrl Pts',(8.44191190459252,23.3941694619224,5.40720171058341));
#83907=CARTESIAN_POINT('Ctrl Pts',(8.41393321396774,23.5465490453474,5.47802561079475));
#83908=CARTESIAN_POINT('Ctrl Pts',(8.38595452334298,23.7016304661779,5.54233682538317));
#83909=CARTESIAN_POINT('Ctrl Pts',(8.35797323329905,23.8567262951743,5.60665401494042));
#83910=CARTESIAN_POINT('Ctrl Pts',(8.32999194325513,24.0145241752471,5.66445718784331));
#83911=CARTESIAN_POINT('Ctrl Pts',(8.3020106532112,24.1744614362556,5.71554100258952));
#83912=CARTESIAN_POINT('Ctrl Pts',(8.27402966129036,24.3343969932329,5.76662427306973));
#83913=CARTESIAN_POINT('Ctrl Pts',(8.24604866936951,24.4964715868972,5.81098823603804));
#83914=CARTESIAN_POINT('Ctrl Pts',(8.21806767744866,24.660106970718,5.84847729499581));
#83915=CARTESIAN_POINT('Ctrl Pts',(8.19008127402464,24.8237740015011,5.88597360430991));
#83916=CARTESIAN_POINT('Ctrl Pts',(8.16209487060061,24.9890021205426,5.91659228413816));
#83917=CARTESIAN_POINT('Ctrl Pts',(8.13410846717658,25.1552016802526,5.94022859820664));
#83918=CARTESIAN_POINT('Ctrl Pts',(8.12441768846202,25.2127511670947,5.94841308285782));
#83919=CARTESIAN_POINT('Ctrl Pts',(8.11472690974746,25.2704170547458,5.95576082645265));
#83920=CARTESIAN_POINT('Ctrl Pts',(8.1050361310329,25.328174656801,5.96226892283765));
#83921=CARTESIAN_POINT('Ctrl Pts',(8.07715920733096,25.4943227356217,5.98099040144255));
#83922=CARTESIAN_POINT('Ctrl Pts',(8.049282283629,25.6612824464083,5.99276581585049));
#83923=CARTESIAN_POINT('Ctrl Pts',(8.02140535992706,25.8284615162792,5.99754737777059));
#83924=CARTESIAN_POINT('Ctrl Pts',(7.99353380797928,25.9956083715171,6.00232801830583));
#83925=CARTESIAN_POINT('Ctrl Pts',(7.96566225603151,26.1629741839552,6.00011748649617));
#83926=CARTESIAN_POINT('Ctrl Pts',(7.93779070408373,26.3299647343038,5.99092006908087));
#83927=CARTESIAN_POINT('Ctrl Pts',(7.90991937032615,26.4969539773803,5.98172272366681));
#83928=CARTESIAN_POINT('Ctrl Pts',(7.88204803656856,26.6635676467278,5.96553861588639));
#83929=CARTESIAN_POINT('Ctrl Pts',(7.85417670281099,26.8292140120055,5.94242409478605));
#83930=CARTESIAN_POINT('Ctrl Pts',(7.82630703023503,26.9948505044619,5.91931095135275));
#83931=CARTESIAN_POINT('Ctrl Pts',(7.79843735765908,27.1595194934828,5.88926826528854));
#83932=CARTESIAN_POINT('Ctrl Pts',(7.77056768508313,27.3226365732627,5.85240399281082));
#83933=CARTESIAN_POINT('Ctrl Pts',(7.7426937768956,27.4857784434519,5.8155341177291));
#83934=CARTESIAN_POINT('Ctrl Pts',(7.71481986870808,27.6473676231973,5.77184065528664));
#83935=CARTESIAN_POINT('Ctrl Pts',(7.68694596052055,27.8068313459651,5.72148236799152));
#83936=CARTESIAN_POINT('Ctrl Pts',(7.67670970052039,27.8653919222526,5.70298906886577));
#83937=CARTESIAN_POINT('Ctrl Pts',(7.66647344052023,27.9236659958665,5.68359743145597));
#83938=CARTESIAN_POINT('Ctrl Pts',(7.65623718052007,27.9816257293065,5.66331700233621));
#83939=CARTESIAN_POINT('Ctrl Pts',(7.62810436935998,28.1409192833715,5.60757931272468));
#83940=CARTESIAN_POINT('Ctrl Pts',(7.59997155819989,28.2978732427479,5.54511207805163));
#83941=CARTESIAN_POINT('Ctrl Pts',(7.5718387470398,28.4519242788586,5.4761361680243));
#83942=CARTESIAN_POINT('Ctrl Pts',(7.5437094058063,28.6059563141739,5.40716876554863));
#83943=CARTESIAN_POINT('Ctrl Pts',(7.5155800645728,28.7570858624845,5.33169441516243));
#83944=CARTESIAN_POINT('Ctrl Pts',(7.4874507233393,28.9047707007979,5.24998163575705));
#83945=CARTESIAN_POINT('Ctrl Pts',(7.45932122986369,29.0524563384138,5.16826841410433));
#83946=CARTESIAN_POINT('Ctrl Pts',(7.43119173638808,29.1966969604368,5.08031684157763));
#83947=CARTESIAN_POINT('Ctrl Pts',(7.40306224291247,29.3369753471838,4.98644116903908));
#83948=CARTESIAN_POINT('Ctrl Pts',(7.37493490097868,29.4772430044515,4.8925726767733));
#83949=CARTESIAN_POINT('Ctrl Pts',(7.34680755904491,29.6135487788148,4.79278116046622));
#83950=CARTESIAN_POINT('Ctrl Pts',(7.31868021711113,29.7454044940789,4.68742415146459));
#83951=CARTESIAN_POINT('Ctrl Pts',(7.29055131360684,29.8772675296933,4.58206129326477));
#83952=CARTESIAN_POINT('Ctrl Pts',(7.26242241010255,30.0046797739015,4.47113251538327));
#83953=CARTESIAN_POINT('Ctrl Pts',(7.23429350659826,30.1271855905679,4.35503606196422));
#83954=CARTESIAN_POINT('Ctrl Pts',(7.22534174773459,30.1661719140137,4.31808945806348));
#83955=CARTESIAN_POINT('Ctrl Pts',(7.21638998887092,30.204661590743,4.28061978349558));
#83956=CARTESIAN_POINT('Ctrl Pts',(7.20743823000725,30.2426406871193,4.24264068711928));
#83957=CARTESIAN_POINT('Ctrl Pts',(7.20743823000725,30.2426406871193,4.24264068711928));
#83958=CARTESIAN_POINT('Ctrl Pts',(7.17951256390743,30.3611192543293,4.1241621199093));
#83959=CARTESIAN_POINT('Ctrl Pts',(7.15158689780761,30.4746441274691,4.00070532573605));
#83960=CARTESIAN_POINT('Ctrl Pts',(7.1236612317078,30.5828090602225,3.87270720782535));
#83961=CARTESIAN_POINT('Ctrl Pts',(7.09573848311536,30.6909626925476,3.74472246239618));
#83962=CARTESIAN_POINT('Ctrl Pts',(7.06781573452291,30.7937572990044,3.61219758103451));
#83963=CARTESIAN_POINT('Ctrl Pts',(7.03989298593048,30.8908263171644,3.47560324768702));
#83964=CARTESIAN_POINT('Ctrl Pts',(7.01196731892867,30.9879054807129,3.33899463787309));
#83965=CARTESIAN_POINT('Ctrl Pts',(6.98404165192688,31.0792576756054,3.19831598171026));
#83966=CARTESIAN_POINT('Ctrl Pts',(6.95611598492507,31.1645587115063,3.05406832199359));
#83967=CARTESIAN_POINT('Ctrl Pts',(6.92819029758115,31.2498598095437,2.90982055720145));
#83968=CARTESIAN_POINT('Ctrl Pts',(6.90026461023721,31.329109582131,2.76200405661523));
#83969=CARTESIAN_POINT('Ctrl Pts',(6.87233892289328,31.4020288818652,2.61114610075623));
#83970=CARTESIAN_POINT('Ctrl Pts',(6.84440696111448,31.4749645653464,2.46025424963772));
#83971=CARTESIAN_POINT('Ctrl Pts',(6.81647499933569,31.5415667979984,2.30631986222865));
#83972=CARTESIAN_POINT('Ctrl Pts',(6.78854303755689,31.6016034918134,2.14989262999423));
#83973=CARTESIAN_POINT('Ctrl Pts',(6.77857511820273,31.6230284431641,2.09406933881066));
#83974=CARTESIAN_POINT('Ctrl Pts',(6.76860719884858,31.6436177061308,2.03792876199264));
#83975=CARTESIAN_POINT('Ctrl Pts',(6.75863927949442,31.6633622351271,1.9814964531224));
#83976=CARTESIAN_POINT('Ctrl Pts',(6.73063866260346,31.71882606589,1.82297395662076));
#83977=CARTESIAN_POINT('Ctrl Pts',(6.70263804571251,31.7676374961679,1.66209993737812));
#83978=CARTESIAN_POINT('Ctrl Pts',(6.67463742882156,31.8096178995698,1.49944651821868));
#83979=CARTESIAN_POINT('Ctrl Pts',(6.64664152822826,31.8515912319819,1.33682049566777));
#83980=CARTESIAN_POINT('Ctrl Pts',(6.61864562763495,31.8867357559632,1.17241597328713));
#83981=CARTESIAN_POINT('Ctrl Pts',(6.59064972704165,31.9149232136785,1.0068184425639));
#83982=CARTESIAN_POINT('Ctrl Pts',(6.56265418668425,31.9431103086931,0.841223042658928));
#83983=CARTESIAN_POINT('Ctrl Pts',(6.53465864632685,31.9643404609087,0.67443497204731));
#83984=CARTESIAN_POINT('Ctrl Pts',(6.50666310596945,31.9785367369739,0.507048799084887));
#83985=CARTESIAN_POINT('Ctrl Pts',(6.4786696187305,31.992731971922,0.339674901779049));
#83986=CARTESIAN_POINT('Ctrl Pts',(6.45067613149154,31.9998943360983,0.171703300649576));
#83987=CARTESIAN_POINT('Ctrl Pts',(6.42268264425259,31.9999988387906,0.00373289588265302));
#83988=CARTESIAN_POINT('Ctrl Pts',(6.39468639976459,32.000103351776,-0.164254053312412));
#83989=CARTESIAN_POINT('Ctrl Pts',(6.3666901552766,31.9931486141029,-0.332239493959689));
#83990=CARTESIAN_POINT('Ctrl Pts',(6.3386939107886,31.9791617556689,-0.499624558590723));
#83991=CARTESIAN_POINT('Ctrl Pts',(6.32907605018627,31.9743566949493,-0.557128207668544));
#83992=CARTESIAN_POINT('Ctrl Pts',(6.31945818958392,31.9687221516902,-0.614561023331037));
#83993=CARTESIAN_POINT('Ctrl Pts',(6.30984032898158,31.962260641641,-0.671898832518117));
#83994=CARTESIAN_POINT('Ctrl Pts',(6.28191923672742,31.9435025804001,-0.838353133131996));
#83995=CARTESIAN_POINT('Ctrl Pts',(6.25399814447326,31.9177675014186,-1.00404004116352));
#83996=CARTESIAN_POINT('Ctrl Pts',(6.2260770522191,31.8851433302929,-1.16836979672903));
#83997=CARTESIAN_POINT('Ctrl Pts',(6.19815917980828,31.8525229213668,-1.33268060188732));
#83998=CARTESIAN_POINT('Ctrl Pts',(6.17024130739745,31.8130150675491,-1.49563425760931));
#83999=CARTESIAN_POINT('Ctrl Pts',(6.14232343498663,31.7667588536228,-1.65665093612492));
#84000=CARTESIAN_POINT('Ctrl Pts',(6.11440302565763,31.7204984363593,-1.81768224634783));
#84001=CARTESIAN_POINT('Ctrl Pts',(6.08648261632864,31.6674885182961,-1.97677592365209));
#84002=CARTESIAN_POINT('Ctrl Pts',(6.05856220699964,31.6079183439335,-2.1333663182336));
#84003=CARTESIAN_POINT('Ctrl Pts',(6.03064197980054,31.5483485581581,-2.28995569134754));
#84004=CARTESIAN_POINT('Ctrl Pts',(6.00272175260146,31.482218716614,-2.44404152052291));
#84005=CARTESIAN_POINT('Ctrl Pts',(5.97480152540236,31.4097666710427,-2.59507698631006));
#84006=CARTESIAN_POINT('Ctrl Pts',(5.94687526507597,31.3372989697099,-2.74614508851467));
#84007=CARTESIAN_POINT('Ctrl Pts',(5.91894900474958,31.2585064723169,-2.89416122631225));
#84008=CARTESIAN_POINT('Ctrl Pts',(5.89102274442319,31.1736739022026,-3.03860138117318));
#84009=CARTESIAN_POINT('Ctrl Pts',(5.88102895577172,31.1433154236031,-3.09029123737288));
#84010=CARTESIAN_POINT('Ctrl Pts',(5.87103516712024,31.1121838396226,-3.14152336661546));
#84011=CARTESIAN_POINT('Ctrl Pts',(5.86104137846877,31.0802935958222,-3.19227457782808));
#84012=CARTESIAN_POINT('Ctrl Pts',(5.83265381532736,30.9897086994383,-3.33643444182407));
#84013=CARTESIAN_POINT('Ctrl Pts',(5.80426625218595,30.8929750200676,-3.47675066095956));
#84014=CARTESIAN_POINT('Ctrl Pts',(5.77587868904454,30.7904383789029,-3.61271368059163));
#84015=CARTESIAN_POINT('Ctrl Pts',(5.74749725742285,30.6879238849523,-3.7486473331402));
#84016=CARTESIAN_POINT('Ctrl Pts',(5.71911582580117,30.5796091072431,-3.88022942977747));
#84017=CARTESIAN_POINT('Ctrl Pts',(5.69073439417949,30.4658817087328,-4.00698147782166));
#84018=CARTESIAN_POINT('Ctrl Pts',(5.67270356408276,30.3936302653519,-4.08750752996593));
#84019=CARTESIAN_POINT('Ctrl Pts',(5.65467273398604,30.3191950666548,-4.16608475088474));
#84020=CARTESIAN_POINT('Ctrl Pts',(5.63664190388932,30.2426838347204,-4.24259753907934));
#84021=CARTESIAN_POINT('',(5.35893340537649,30.2426406871193,4.24264068711929));
#84022=CARTESIAN_POINT('Ctrl Pts',(3.78813707791307,30.2426869010466,-4.24259447268859));
#84023=CARTESIAN_POINT('Ctrl Pts',(3.816515452064,30.3631064902981,-4.12217225999875));
#84024=CARTESIAN_POINT('Ctrl Pts',(3.84489382621493,30.4783816103409,-3.99663448658121));
#84025=CARTESIAN_POINT('Ctrl Pts',(3.87327220036586,30.5880993722131,-3.86643817365513));
#84026=CARTESIAN_POINT('Ctrl Pts',(3.90165911004251,30.6978501345234,-3.73620270084018));
#84027=CARTESIAN_POINT('Ctrl Pts',(3.93004601971916,30.8020400105107,-3.60130611285029));
#84028=CARTESIAN_POINT('Ctrl Pts',(3.95843292939582,30.9002961498858,-3.46223881952335));
#84029=CARTESIAN_POINT('Ctrl Pts',(3.97646747087655,30.9627194443367,-3.37388771337318));
#84030=CARTESIAN_POINT('Ctrl Pts',(3.99450201235727,31.0227485778494,-3.28385387398067));
#84031=CARTESIAN_POINT('Ctrl Pts',(4.012536553838,31.0802969047552,-3.19226931187434));
#84032=CARTESIAN_POINT('Ctrl Pts',(4.04046279521554,31.1694097036452,-3.05045186724619));
#84033=CARTESIAN_POINT('Ctrl Pts',(4.06838903659308,31.252595263152,-2.90487727016411));
#84034=CARTESIAN_POINT('Ctrl Pts',(4.09631527797061,31.3295526946622,-2.75606024513595));
#84035=CARTESIAN_POINT('Ctrl Pts',(4.12423606502702,31.4064950954872,-2.60727228581099));
#84036=CARTESIAN_POINT('Ctrl Pts',(4.15215685208344,31.4772116508648,-2.45524344240145));
#84037=CARTESIAN_POINT('Ctrl Pts',(4.18007763913985,31.5414475513461,-2.30051277668276));
#84038=CARTESIAN_POINT('Ctrl Pts',(4.20799765893873,31.6056816866379,-2.14578636293118));
#84039=CARTESIAN_POINT('Ctrl Pts',(4.23591767873761,31.6634353986696,-1.98835856524518));
#84040=CARTESIAN_POINT('Ctrl Pts',(4.26383769853649,31.7145018662962,-1.82878878498768));
#84041=CARTESIAN_POINT('Ctrl Pts',(4.29175562275567,31.7655645010513,-1.66923098148356));
#84042=CARTESIAN_POINT('Ctrl Pts',(4.31967354697488,31.8099407990447,-1.50753181741852));
#84043=CARTESIAN_POINT('Ctrl Pts',(4.34759147119407,31.8474736019631,-1.34426651908945));
#84044=CARTESIAN_POINT('Ctrl Pts',(4.37551264680177,31.8850107760418,-1.18098220649159));
#84045=CARTESIAN_POINT('Ctrl Pts',(4.40343382240945,31.9157027919866,-1.01613170273964));
#84046=CARTESIAN_POINT('Ctrl Pts',(4.43135499801715,31.939443307781,-0.8503018250333));
#84047=CARTESIAN_POINT('Ctrl Pts',(4.44134850012838,31.9479404748791,-0.790948262839224));
#84048=CARTESIAN_POINT('Ctrl Pts',(4.45134200223961,31.9555475942772,-0.731469320963337));
#84049=CARTESIAN_POINT('Ctrl Pts',(4.46133550435084,31.9622613954461,-0.671892143407596));
#84050=CARTESIAN_POINT('Ctrl Pts',(4.48933160516719,31.9810696422743,-0.504990825867469));
#84051=CARTESIAN_POINT('Ctrl Pts',(4.51732770598352,31.992867180341,-0.337284199462853));
#84052=CARTESIAN_POINT('Ctrl Pts',(4.54532380679987,31.9976090079534,-0.169369972888486));
#84053=CARTESIAN_POINT('Ctrl Pts',(4.57331711061984,32.0023503618258,-0.00147252206045653));
#84054=CARTESIAN_POINT('Ctrl Pts',(4.60131041443981,32.0000374038039,0.166632175800177));
#84055=CARTESIAN_POINT('Ctrl Pts',(4.62930371825977,31.9906772214171,0.334344775336205));
#84056=CARTESIAN_POINT('Ctrl Pts',(4.65729949760172,31.9813162112846,0.502072206141611));
#84057=CARTESIAN_POINT('Ctrl Pts',(4.68529527694368,31.9649067465216,0.669407157710664));
#84058=CARTESIAN_POINT('Ctrl Pts',(4.71329105628564,31.9415079690106,0.835752986344446));
#84059=CARTESIAN_POINT('Ctrl Pts',(4.74128642739747,31.918109532697,1.00209638934909));
#84060=CARTESIAN_POINT('Ctrl Pts',(4.76928179850931,31.8877220334429,1.16745038970294));
#84061=CARTESIAN_POINT('Ctrl Pts',(4.79727716962114,31.8504561912662,1.33122588394137));
#84062=CARTESIAN_POINT('Ctrl Pts',(4.82527768223529,31.8131835050147,1.49503145644092));
#84063=CARTESIAN_POINT('Ctrl Pts',(4.85327819484944,31.7690300219162,1.65725763956866));
#84064=CARTESIAN_POINT('Ctrl Pts',(4.88127870746359,31.7181572341969,1.81732711557434));
#84065=CARTESIAN_POINT('Ctrl Pts',(4.89089728993028,31.7006816932762,1.87231330374087));
#84066=CARTESIAN_POINT('Ctrl Pts',(4.90051587239697,31.6824136939749,1.92704512147826));
#84067=CARTESIAN_POINT('Ctrl Pts',(4.91013445486366,31.6633611357654,1.98149959523123));
#84068=CARTESIAN_POINT('Ctrl Pts',(4.93806707679286,31.6080319947938,2.13963685017107));
#84069=CARTESIAN_POINT('Ctrl Pts',(4.96599969872205,31.5460659526854,2.2954819267778));
#84070=CARTESIAN_POINT('Ctrl Pts',(4.99393232065124,31.4776777973362,2.44847829244406));
#84071=CARTESIAN_POINT('Ctrl Pts',(5.02185928540985,31.4093034925831,2.60144367188414));
#84072=CARTESIAN_POINT('Ctrl Pts',(5.04978625016845,31.334509798614,2.75156120412281));
#84073=CARTESIAN_POINT('Ctrl Pts',(5.07771321492705,31.2535592679187,2.89829519174042));
#84074=CARTESIAN_POINT('Ctrl Pts',(5.10563904188241,31.1726120353182,3.04502320110693));
#84075=CARTESIAN_POINT('Ctrl Pts',(5.13356486883776,31.0855086162654,3.18836766367047));
#84076=CARTESIAN_POINT('Ctrl Pts',(5.16149069579312,30.9925573914775,3.32781770726749));
#84077=CARTESIAN_POINT('Ctrl Pts',(5.18941419241778,30.8996139232046,3.46725611415569));
#84078=CARTESIAN_POINT('Ctrl Pts',(5.21733768904245,30.8008237995959,3.60280048960743));
#84079=CARTESIAN_POINT('Ctrl Pts',(5.24526118566711,30.6965387529717,3.73396889941992));
#84080=CARTESIAN_POINT('Ctrl Pts',(5.27318753576663,30.5922430495604,3.86515071320411));
#84081=CARTESIAN_POINT('Ctrl Pts',(5.30111388586613,30.4824514972791,3.99195542114597));
#84082=CARTESIAN_POINT('Ctrl Pts',(5.32904023596565,30.3675565881145,4.11393357379745));
#84083=CARTESIAN_POINT('Ctrl Pts',(5.33900462576926,30.3265609815534,4.15745654963257));
#84084=CARTESIAN_POINT('Ctrl Pts',(5.34896901557288,30.2849160127224,4.20036536151615));
#84085=CARTESIAN_POINT('Ctrl Pts',(5.35893340537649,30.2426406871193,4.24264068711928));
#84086=CARTESIAN_POINT('',(8.50052610236153,21.7573593077119,-4.24264069228803));
#84087=CARTESIAN_POINT('Ctrl Pts',(5.35893340537649,30.2426406871193,4.24264068711928));
#84088=CARTESIAN_POINT('Ctrl Pts',(5.3870628280945,30.1232976537907,4.3619837204479));
#84089=CARTESIAN_POINT('Ctrl Pts',(5.41519225081251,29.9989103679391,4.47629371275373));
#84090=CARTESIAN_POINT('Ctrl Pts',(5.44332167353052,29.8699233733809,4.58516009362379));
#84091=CARTESIAN_POINT('Ctrl Pts',(5.47144933461812,29.7409444567494,4.69401965663878));
#84092=CARTESIAN_POINT('Ctrl Pts',(5.49957699570573,29.6073666401139,4.79743609238796));
#84093=CARTESIAN_POINT('Ctrl Pts',(5.52770465679333,29.4696681199931,4.89503862467947));
#84094=CARTESIAN_POINT('Ctrl Pts',(5.55583498230706,29.3319565562162,4.99265040248689));
#84095=CARTESIAN_POINT('Ctrl Pts',(5.58396530782079,29.1901237569449,5.08444699821659));
#84096=CARTESIAN_POINT('Ctrl Pts',(5.61209563333453,29.0446781877336,5.17010006993478));
#84097=CARTESIAN_POINT('Ctrl Pts',(5.64022526627055,28.8992361994392,5.25575103284663));
#84098=CARTESIAN_POINT('Ctrl Pts',(5.66835489920657,28.7501818832098,5.33525862111028));
#84099=CARTESIAN_POINT('Ctrl Pts',(5.69648453214259,28.5980499480886,5.40833952958181));
#84100=CARTESIAN_POINT('Ctrl Pts',(5.72461782373482,28.4458982260597,5.48142994325803));
#84101=CARTESIAN_POINT('Ctrl Pts',(5.75275111532705,28.2906683607607,5.54809187525009));
#84102=CARTESIAN_POINT('Ctrl Pts',(5.78088440691927,28.1329175038741,5.60808906149571));
#84103=CARTESIAN_POINT('Ctrl Pts',(5.78983372324263,28.0827363043535,5.62717441439382));
#84104=CARTESIAN_POINT('Ctrl Pts',(5.79878303956597,28.0323001564974,5.64558572516284));
#84105=CARTESIAN_POINT('Ctrl Pts',(5.80773235588932,27.981627395157,5.66331641944572));
#84106=CARTESIAN_POINT('Ctrl Pts',(5.83560583606672,27.8238023549277,5.71854032010687));
#84107=CARTESIAN_POINT('Ctrl Pts',(5.86347931624414,27.6636453184919,5.76717046119707));
#84108=CARTESIAN_POINT('Ctrl Pts',(5.89135279642155,27.5017235010104,5.80902974054302));
#84109=CARTESIAN_POINT('Ctrl Pts',(5.91922222299253,27.3398252316225,5.85088293234471));
#84110=CARTESIAN_POINT('Ctrl Pts',(5.94709164956352,27.1761630010024,5.88596714805155));
#84111=CARTESIAN_POINT('Ctrl Pts',(5.97496107613449,27.0113173742088,5.9141556598236));
#84112=CARTESIAN_POINT('Ctrl Pts',(6.00283223854301,26.8464614800627,5.9423459273073));
#84113=CARTESIAN_POINT('Ctrl Pts',(6.03070340095152,26.6804223552794,5.96363957616521));
#84114=CARTESIAN_POINT('Ctrl Pts',(6.05857456336004,26.5137896250338,5.97796120940976));
#84115=CARTESIAN_POINT('Ctrl Pts',(6.08644519597083,26.3471600622786,5.99228257041705));
#84116=CARTESIAN_POINT('Ctrl Pts',(6.11431582858164,26.1799372335241,5.99963215607804));
#84117=CARTESIAN_POINT('Ctrl Pts',(6.14218646119243,26.0127149542826,5.99998652747968));
#84118=CARTESIAN_POINT('Ctrl Pts',(6.17006298049281,25.845457355224,6.0003409737298));
#84119=CARTESIAN_POINT('Ctrl Pts',(6.19793949979319,25.6782006238214,5.99369725404834));
#84120=CARTESIAN_POINT('Ctrl Pts',(6.22581601909357,25.511538413208,5.9800840527729));
#84121=CARTESIAN_POINT('Ctrl Pts',(6.23605444819643,25.4503270686674,5.97508422497447));
#84122=CARTESIAN_POINT('Ctrl Pts',(6.24629287729929,25.3891958917371,5.96914476897281));
#84123=CARTESIAN_POINT('Ctrl Pts',(6.25653130640214,25.3281741450145,5.96226886516979));
#84124=CARTESIAN_POINT('Ctrl Pts',(6.28451774466434,25.1613730342045,5.94347378876237));
#84125=CARTESIAN_POINT('Ctrl Pts',(6.31250418292654,24.9953373785667,5.91767204983512));
#84126=CARTESIAN_POINT('Ctrl Pts',(6.34049062118875,24.8306595845358,5.8849505514288));
#84127=CARTESIAN_POINT('Ctrl Pts',(6.36847212349185,24.6660108346743,5.8522348241026));
#84128=CARTESIAN_POINT('Ctrl Pts',(6.39645362579495,24.5027197749735,5.81260183387982));
#84129=CARTESIAN_POINT('Ctrl Pts',(6.42443512809806,24.341369031207,5.76618966990863));
#84130=CARTESIAN_POINT('Ctrl Pts',(6.45241608108101,24.1800214550052,5.71977841707999));
#84131=CARTESIAN_POINT('Ctrl Pts',(6.48039703406395,24.0206144199361,5.66658833974929));
#84132=CARTESIAN_POINT('Ctrl Pts',(6.5083779870469,23.8637164806476,5.60680771249946));
#84133=CARTESIAN_POINT('Ctrl Pts',(6.53635681619747,23.7068304503503,5.547031622766));
#84134=CARTESIAN_POINT('Ctrl Pts',(6.56433564534805,23.5524534270869,5.48066609483771));
#84135=CARTESIAN_POINT('Ctrl Pts',(6.59231447449862,23.4011353477862,5.40794808771993));
#84136=CARTESIAN_POINT('Ctrl Pts',(6.62029606770103,23.2498023196464,5.33522289672965));
#84137=CARTESIAN_POINT('Ctrl Pts',(6.64827766090344,23.1015291210748,5.25614410805374));
#84138=CARTESIAN_POINT('Ctrl Pts',(6.67625925410585,22.9568430559818,5.17099563083105));
#84139=CARTESIAN_POINT('Ctrl Pts',(6.68594958837556,22.906736676235,5.14150777426493));
#84140=CARTESIAN_POINT('Ctrl Pts',(6.69563992264525,22.8570602862605,5.11129237445357));
#84141=CARTESIAN_POINT('Ctrl Pts',(6.70533025691496,22.8078350564431,5.08036248442237));
#84142=CARTESIAN_POINT('Ctrl Pts',(6.73328239323225,22.6658430161469,4.99114404485486));
#84143=CARTESIAN_POINT('Ctrl Pts',(6.76123452954954,22.5275793803426,4.89596010939473));
#84144=CARTESIAN_POINT('Ctrl Pts',(6.78918666586683,22.3935381982795,4.79514684579429));
#84145=CARTESIAN_POINT('Ctrl Pts',(6.8171358543992,22.2595111519723,4.69434421378974));
#84146=CARTESIAN_POINT('Ctrl Pts',(6.84508504293158,22.1297059213547,4.58791362749829));
#84147=CARTESIAN_POINT('Ctrl Pts',(6.87303423146396,22.004585380564,4.47623301658856));
#84148=CARTESIAN_POINT('Ctrl Pts',(6.90098607860559,21.8794529379384,4.36454178228968));
#84149=CARTESIAN_POINT('Ctrl Pts',(6.92893792574723,21.759006311528,4.2475997328004));
#84150=CARTESIAN_POINT('Ctrl Pts',(6.95688977288886,21.6436738204348,4.12582382285462));
#84151=CARTESIAN_POINT('Ctrl Pts',(6.98484143161379,21.5283421067702,4.00404873377111));
#84152=CARTESIAN_POINT('Ctrl Pts',(7.0127930903387,21.4181246733265,3.87744007942548));
#84153=CARTESIAN_POINT('Ctrl Pts',(7.04074474906362,21.3134117771372,3.74645043065086));
#84154=CARTESIAN_POINT('Ctrl Pts',(7.0687022001181,21.2086771816417,3.61543363732567));
#84155=CARTESIAN_POINT('Ctrl Pts',(7.09665965117257,21.1094495978143,3.48003428166612));
#84156=CARTESIAN_POINT('Ctrl Pts',(7.12461710222705,21.0160784017799,3.34073726934573));
#84157=CARTESIAN_POINT('Ctrl Pts',(7.13445447062729,20.9832239455002,3.29172292878301));
#84158=CARTESIAN_POINT('Ctrl Pts',(7.14429183902755,20.951094195107,3.24222628351));
#84159=CARTESIAN_POINT('Ctrl Pts',(7.1541292074278,20.9197030952448,3.19226931187431));
#84160=CARTESIAN_POINT('Ctrl Pts',(7.18205544880533,20.8305902963548,3.05045186724616));
#84161=CARTESIAN_POINT('Ctrl Pts',(7.20998169018287,20.747404736848,2.9048772701641));
#84162=CARTESIAN_POINT('Ctrl Pts',(7.2379079315604,20.6704473053378,2.75606024513595));
#84163=CARTESIAN_POINT('Ctrl Pts',(7.26582871861674,20.593504904513,2.60727228581136));
#84164=CARTESIAN_POINT('Ctrl Pts',(7.29374950567309,20.5227883491355,2.4552434424022));
#84165=CARTESIAN_POINT('Ctrl Pts',(7.32167029272943,20.4585524486544,2.30051277668391));
#84166=CARTESIAN_POINT('Ctrl Pts',(7.34959031252838,20.3943183133624,2.145786362932));
#84167=CARTESIAN_POINT('Ctrl Pts',(7.37751033232731,20.3365646013306,1.98835856524566));
#84168=CARTESIAN_POINT('Ctrl Pts',(7.40543035212626,20.2854981337038,1.8287887849878));
#84169=CARTESIAN_POINT('Ctrl Pts',(7.43334827634547,20.2344354989487,1.66923098148351));
#84170=CARTESIAN_POINT('Ctrl Pts',(7.46126620056469,20.1900592009552,1.50753181741829));
#84171=CARTESIAN_POINT('Ctrl Pts',(7.48918412478391,20.1525263980368,1.34426651908904));
#84172=CARTESIAN_POINT('Ctrl Pts',(7.51710530039168,20.114989223958,1.18098220649074));
#84173=CARTESIAN_POINT('Ctrl Pts',(7.54502647599945,20.0842972080132,1.01613170273834));
#84174=CARTESIAN_POINT('Ctrl Pts',(7.57294765160723,20.0605566922187,0.850301825031545));
#84175=CARTESIAN_POINT('Ctrl Pts',(7.58294115371836,20.0520595251207,0.790948262838054));
#84176=CARTESIAN_POINT('Ctrl Pts',(7.59293465582949,20.0444524057227,0.731469320962755));
#84177=CARTESIAN_POINT('Ctrl Pts',(7.60292815794062,20.0377386045539,0.671892143407602));
#84178=CARTESIAN_POINT('Ctrl Pts',(7.63092425875694,20.0189303577257,0.504990825867639));
#84179=CARTESIAN_POINT('Ctrl Pts',(7.65892035957326,20.0071328196591,0.33728419946319));
#84180=CARTESIAN_POINT('Ctrl Pts',(7.68691646038959,20.0023909920466,0.169369972888987));
#84181=CARTESIAN_POINT('Ctrl Pts',(7.71490976420946,19.9976496381742,0.00147252206147364));
#84182=CARTESIAN_POINT('Ctrl Pts',(7.74290306802933,19.9999625961961,-0.166632175798642));
#84183=CARTESIAN_POINT('Ctrl Pts',(7.77089637184921,20.0093227785828,-0.33434477533416));
#84184=CARTESIAN_POINT('Ctrl Pts',(7.79889215119115,20.0186837887153,-0.502072206139494));
#84185=CARTESIAN_POINT('Ctrl Pts',(7.8268879305331,20.0350932534782,-0.669407157708479));
#84186=CARTESIAN_POINT('Ctrl Pts',(7.85488370987504,20.0584920309891,-0.835752986342195));
#84187=CARTESIAN_POINT('Ctrl Pts',(7.88287908098689,20.0818904673027,-1.00209638934693));
#84188=CARTESIAN_POINT('Ctrl Pts',(7.91087445209875,20.1122779665567,-1.16745038970086));
#84189=CARTESIAN_POINT('Ctrl Pts',(7.9388698232106,20.1495438087334,-1.33122588393938));
#84190=CARTESIAN_POINT('Ctrl Pts',(7.96687033582474,20.1868164949848,-1.49503145643893));
#84191=CARTESIAN_POINT('Ctrl Pts',(7.99487084843889,20.2309699780832,-1.65725763956667));
#84192=CARTESIAN_POINT('Ctrl Pts',(8.02287136105303,20.2818427658025,-1.81732711557235));
#84193=CARTESIAN_POINT('Ctrl Pts',(8.03248994351984,20.2993183067234,-1.87231330373955));
#84194=CARTESIAN_POINT('Ctrl Pts',(8.04210852598664,20.3175863060249,-1.92704512147761));
#84195=CARTESIAN_POINT('Ctrl Pts',(8.05172710845345,20.3366388642346,-1.98149959523124));
#84196=CARTESIAN_POINT('Ctrl Pts',(8.07965973038267,20.3919680052063,-2.13963685017114));
#84197=CARTESIAN_POINT('Ctrl Pts',(8.10759235231187,20.4539340473147,-2.29548192677793));
#84198=CARTESIAN_POINT('Ctrl Pts',(8.13552497424108,20.5223222026639,-2.44847829244425));
#84199=CARTESIAN_POINT('Ctrl Pts',(8.16345193899964,20.5906965074169,-2.60144367188407));
#84200=CARTESIAN_POINT('Ctrl Pts',(8.1913789037582,20.6654902013859,-2.75156120412248));
#84201=CARTESIAN_POINT('Ctrl Pts',(8.21930586851675,20.746440732081,-2.89829519173985));
#84202=CARTESIAN_POINT('Ctrl Pts',(8.24723169547209,20.8273879646814,-3.04502320110628));
#84203=CARTESIAN_POINT('Ctrl Pts',(8.27515752242742,20.9144913837342,-3.18836766366975));
#84204=CARTESIAN_POINT('Ctrl Pts',(8.30308334938276,21.0074426085219,-3.3278177072667));
#84205=CARTESIAN_POINT('Ctrl Pts',(8.33100684600741,21.1003860767948,-3.46725611415485));
#84206=CARTESIAN_POINT('Ctrl Pts',(8.35893034263206,21.1991762004034,-3.60280048960655));
#84207=CARTESIAN_POINT('Ctrl Pts',(8.38685383925671,21.3034612470276,-3.73396889941901));
#84208=CARTESIAN_POINT('Ctrl Pts',(8.4147801893562,21.4077569504388,-3.86515071320316));
#84209=CARTESIAN_POINT('Ctrl Pts',(8.44270653945571,21.51754850272,-3.99195542114498));
#84210=CARTESIAN_POINT('Ctrl Pts',(8.47063288955521,21.6324434118846,-4.11393357379643));
#84211=CARTESIAN_POINT('Ctrl Pts',(8.4805972793589,21.673439018446,-4.1574565496319));
#84212=CARTESIAN_POINT('Ctrl Pts',(8.49056166916259,21.7150839872773,-4.20036536151581));
#84213=CARTESIAN_POINT('Ctrl Pts',(8.50052605896628,21.7573593128807,-4.24264068711927));
#84214=CARTESIAN_POINT('Ctrl Pts',(8.50052615178669,21.7573593128807,-4.24264068711927));
#84215=CARTESIAN_POINT('Ctrl Pts',(8.52865485901884,21.8766993106599,-4.36198068489846));
#84216=CARTESIAN_POINT('Ctrl Pts',(8.55678356625099,22.0010833453181,-4.47628793832941));
#84217=CARTESIAN_POINT('Ctrl Pts',(8.58491227348314,22.1300669041397,-4.58515188773124));
#84218=CARTESIAN_POINT('Ctrl Pts',(8.61303920813034,22.2590423348126,-4.69400897686049));
#84219=CARTESIAN_POINT('Ctrl Pts',(8.64116614277755,22.392616477355,-4.79742325031555));
#84220=CARTESIAN_POINT('Ctrl Pts',(8.66929307742474,22.5303111654473,-4.89502394185975));
#84221=CARTESIAN_POINT('Ctrl Pts',(8.69742266764845,22.6680188538464,-4.99263384827602));
#84222=CARTESIAN_POINT('Ctrl Pts',(8.72555225787215,22.8098476171784,-5.08442889782456));
#84223=CARTESIAN_POINT('Ctrl Pts',(8.75368184809586,22.9552890194459,-5.17008075806301));
#84224=CARTESIAN_POINT('Ctrl Pts',(8.78181074280473,23.1007268256194,-5.25573050052658));
#84225=CARTESIAN_POINT('Ctrl Pts',(8.80993963751361,23.2497768279433,-5.33523720429478));
#84226=CARTESIAN_POINT('Ctrl Pts',(8.83806853222248,23.4019043463697,-5.40831757338522));
#84227=CARTESIAN_POINT('Ctrl Pts',(8.86620108713286,23.554051660006,-5.48140745187444));
#84228=CARTESIAN_POINT('Ctrl Pts',(8.89433364204323,23.7092770144246,-5.54806919311663));
#84229=CARTESIAN_POINT('Ctrl Pts',(8.92246619695361,23.8670232865689,-5.60806654204109));
#84230=CARTESIAN_POINT('Ctrl Pts',(8.93141916540225,23.9172248200556,-5.62716023522444));
#84231=CARTESIAN_POINT('Ctrl Pts',(8.94037213385088,23.9676815158992,-5.64557933645468));
#84232=CARTESIAN_POINT('Ctrl Pts',(8.94932510229951,24.0183750162368,-5.66331726320585));
#84233=CARTESIAN_POINT('Ctrl Pts',(8.97719914199932,24.1762034112589,-5.71854226229871));
#84234=CARTESIAN_POINT('Ctrl Pts',(9.00507318169912,24.3363638091913,-5.76717319154773));
#84235=CARTESIAN_POINT('Ctrl Pts',(9.03294722139892,24.4982889653192,-5.8090329632666));
#84236=CARTESIAN_POINT('Ctrl Pts',(9.06081722659187,24.6601906842935,-5.85088667617456));
#84237=CARTESIAN_POINT('Ctrl Pts',(9.08868723178481,24.8238563441035,-5.88597110800244));
#84238=CARTESIAN_POINT('Ctrl Pts',(9.11655723697776,24.9887053523151,-5.91415954600176));
#84239=CARTESIAN_POINT('Ctrl Pts',(9.14442900138379,25.1535647661413,-5.94234976331433));
#84240=CARTESIAN_POINT('Ctrl Pts',(9.17230076578983,25.3196073648312,-5.96364306054573));
#84241=CARTESIAN_POINT('Ctrl Pts',(9.20017253019587,25.4862434973884,-5.97796405610006));
#84242=CARTESIAN_POINT('Ctrl Pts',(9.22804377704257,25.6528765356282,-5.99228478572342));
#84243=CARTESIAN_POINT('Ctrl Pts',(9.25591502388926,25.8201027688212,-5.99963344784175));
#84244=CARTESIAN_POINT('Ctrl Pts',(9.28378627073596,25.9873283575251,-5.99998661910815));
#84245=CARTESIAN_POINT('Ctrl Pts',(9.31166341799586,26.1545893483077,-6.00033986514181));
#84246=CARTESIAN_POINT('Ctrl Pts',(9.33954056525577,26.3218493764439,-5.99369466172522));
#84247=CARTESIAN_POINT('Ctrl Pts',(9.36741771251567,26.4885147662724,-5.98007970876089));
#84248=CARTESIAN_POINT('Ctrl Pts',(9.37765315928123,26.5497080694948,-5.97508080679352));
#84249=CARTESIAN_POINT('Ctrl Pts',(9.38788860604678,26.6108212395971,-5.96914283018167));
#84250=CARTESIAN_POINT('Ctrl Pts',(9.39812405281234,26.6718250404551,-5.96226895695066));
#84251=CARTESIAN_POINT('Ctrl Pts',(9.42611042972821,26.8386253182754,-5.94347399748075));
#84252=CARTESIAN_POINT('Ctrl Pts',(9.45409680664407,27.0046601922689,-5.91767244072537));
#84253=CARTESIAN_POINT('Ctrl Pts',(9.48208318355993,27.1693372600206,-5.88495117841495));
#84254=CARTESIAN_POINT('Ctrl Pts',(9.51006461450599,27.3339852247624,-5.85223569886003));
#84255=CARTESIAN_POINT('Ctrl Pts',(9.53804604545205,27.4972755556528,-5.81260301525687));
#84256=CARTESIAN_POINT('Ctrl Pts',(9.56602747639812,27.6586256298888,-5.76619120562924));
#84257=CARTESIAN_POINT('Ctrl Pts',(9.59400834442122,27.819972458127,-5.71978032970201));
#84258=CARTESIAN_POINT('Ctrl Pts',(9.62198921244433,27.979378806388,-5.66659068357769));
#84259=CARTESIAN_POINT('Ctrl Pts',(9.64997008046744,28.1362761222771,-5.60681053089799));
#84260=CARTESIAN_POINT('Ctrl Pts',(9.67794881712259,28.2931614869319,-5.54703493181189));
#84261=CARTESIAN_POINT('Ctrl Pts',(9.70592755377774,28.4475379092945,-5.48066994143182));
#84262=CARTESIAN_POINT('Ctrl Pts',(9.73390629043289,28.5988554537139,-5.40795250817734));
#84263=CARTESIAN_POINT('Ctrl Pts',(9.76188778115008,28.750187892941,-5.33522791704707));
#84264=CARTESIAN_POINT('Ctrl Pts',(9.78986927186726,28.8984605708052,-5.25614976907949));
#84265=CARTESIAN_POINT('Ctrl Pts',(9.81785076258445,29.0431461839619,-5.17100196316323));
#84266=CARTESIAN_POINT('Ctrl Pts',(9.82754150949802,29.0932547244006,-5.14151297539912));
#84267=CARTESIAN_POINT('Ctrl Pts',(9.8372322564116,29.1429332435305,-5.11129638076745));
#84268=CARTESIAN_POINT('Ctrl Pts',(9.84692300332517,29.1921605680295,-5.08036523371278));
#84269=CARTESIAN_POINT('Ctrl Pts',(9.87501419887874,29.3348590010206,-4.99070311495582));
#84270=CARTESIAN_POINT('Ctrl Pts',(9.90310539443231,29.4737906803365,-4.89501678685941));
#84271=CARTESIAN_POINT('Ctrl Pts',(9.93119658998587,29.60845675826,-4.79364577579194));
#84272=CARTESIAN_POINT('Ctrl Pts',(9.95928583520492,29.7431134864959,-4.69228180277956));
#84273=CARTESIAN_POINT('Ctrl Pts',(9.98737508042397,29.8735049579827,-4.58523411793288));
#84274=CARTESIAN_POINT('Ctrl Pts',(10.015464325643,29.9991634074874,-4.47288408526466));
#84275=CARTESIAN_POINT('Ctrl Pts',(10.034083709733,30.0824580249553,-4.39841115463005));
#84276=CARTESIAN_POINT('Ctrl Pts',(10.0527030938231,30.1636736421363,-4.32160928184441));
#84277=CARTESIAN_POINT('Ctrl Pts',(10.0713224779131,30.2426823068249,-4.24259906700534));
#84278=CARTESIAN_POINT('Origin',(-31.4159265358979,26.,7.7715611723761E-15));
#84279=CARTESIAN_POINT('',(17.341,30.2426406871193,-4.24264068711928));
#84280=CARTESIAN_POINT('',(16.354507877922,30.2426778922245,-4.24260348168784));
#84281=CARTESIAN_POINT('',(-31.4159265358979,30.2426406871193,-4.24264068711928));
#84282=CARTESIAN_POINT('',(17.341,25.540762340228,-5.98239924878364));
#84283=CARTESIAN_POINT('Origin',(17.341,26.,7.7715611723761E-15));
#84284=CARTESIAN_POINT('',(16.6322163269923,21.7573593180495,-4.24264068195053));
#84285=CARTESIAN_POINT('Ctrl Pts',(17.341,25.540762340228,-5.98239924878364));
#84286=CARTESIAN_POINT('Ctrl Pts',(17.2225532411293,24.8321665389389,-5.92800403643227));
#84287=CARTESIAN_POINT('Ctrl Pts',(17.1059809364002,24.1388327450978,-5.748143051765));
#84288=CARTESIAN_POINT('Ctrl Pts',(16.8692225121782,22.847541981894,-5.15431362704027));
#84289=CARTESIAN_POINT('Ctrl Pts',(16.750641223211,22.2597933862528,-4.74507476049141));
#84290=CARTESIAN_POINT('Ctrl Pts',(16.6322163764174,21.7573593128807,-4.24264068711927));
#84291=CARTESIAN_POINT('',(13.4906236300072,30.2426406871193,4.24264068711929));
#84292=CARTESIAN_POINT('Ctrl Pts',(16.632216283597,21.7573593128807,-4.24264068711927));
#84293=CARTESIAN_POINT('Ctrl Pts',(16.6042913968638,21.6388840522434,-4.12416542648196));
#84294=CARTESIAN_POINT('Ctrl Pts',(16.5763665101307,21.5253621514006,-4.00071215862345));
#84295=CARTESIAN_POINT('Ctrl Pts',(16.5484416233975,21.4171998487376,-3.87271775031295));
#84296=CARTESIAN_POINT('Ctrl Pts',(16.5205196696009,21.3090489063057,-3.74473678518948));
#84297=CARTESIAN_POINT('Ctrl Pts',(16.4925977158043,21.2062566416934,-3.6122158724385));
#84298=CARTESIAN_POINT('Ctrl Pts',(16.4646757620076,21.1091896105983,-3.47562566093074));
#84299=CARTESIAN_POINT('Ctrl Pts',(16.436750905734,21.0121124894206,-3.33902125092011));
#84300=CARTESIAN_POINT('Ctrl Pts',(16.4088260494604,20.9207619755784,-3.19834695246211));
#84301=CARTESIAN_POINT('Ctrl Pts',(16.3809011931868,20.8354622534116,-3.05410377427876));
#84302=CARTESIAN_POINT('Ctrl Pts',(16.3529763239393,20.7501624916145,-2.90986052907979));
#84303=CARTESIAN_POINT('Ctrl Pts',(16.3250514546917,20.6709136847872,-2.76204867382332));
#84304=CARTESIAN_POINT('Ctrl Pts',(16.2971265854442,20.5979949749762,-2.61119545603485));
#84305=CARTESIAN_POINT('Ctrl Pts',(16.2691954467488,20.5250598940929,-2.46030836999875));
#84306=CARTESIAN_POINT('Ctrl Pts',(16.2412643080534,20.4584578858779,-2.30637884153029));
#84307=CARTESIAN_POINT('Ctrl Pts',(16.213333169358,20.398421033345,-2.14995652986948));
#84308=CARTESIAN_POINT('Ctrl Pts',(16.2033612239334,20.3769867401194,-2.09411080255835));
#84309=CARTESIAN_POINT('Ctrl Pts',(16.1933892785088,20.3563888110039,-2.0379475223848));
#84310=CARTESIAN_POINT('Ctrl Pts',(16.1834173330842,20.3366363029578,-1.98149227478286));
#84311=CARTESIAN_POINT('Ctrl Pts',(16.1554166241976,20.2811722782334,-1.82296884872001));
#84312=CARTESIAN_POINT('Ctrl Pts',(16.127415915311,20.2323607377876,-1.66209389997231));
#84313=CARTESIAN_POINT('Ctrl Pts',(16.0994152064245,20.1903803043503,-1.49943955927496));
#84314=CARTESIAN_POINT('Ctrl Pts',(16.0714192091262,20.1484069348241,-1.33681258789509));
#84315=CARTESIAN_POINT('Ctrl Pts',(16.043423211828,20.1132624561311,-1.17240712404425));
#84316=CARTESIAN_POINT('Ctrl Pts',(16.0154272145297,20.0850751222934,-1.00680866657375));
#84317=CARTESIAN_POINT('Ctrl Pts',(15.987431571927,20.0568881455754,-0.84121230715428));
#84318=CARTESIAN_POINT('Ctrl Pts',(15.9594359293243,20.0356581929918,-0.674423291272229));
#84319=CARTESIAN_POINT('Ctrl Pts',(15.9314402867215,20.0214621940045,-0.507036194252439));
#84320=CARTESIAN_POINT('Ctrl Pts',(15.9034466944445,20.0072672346939,-0.339661356213942));
#84321=CARTESIAN_POINT('Ctrl Pts',(15.8754531021674,20.0001052249912,-0.171688835435331));
#84322=CARTESIAN_POINT('Ctrl Pts',(15.8474595098903,20.0000011516745,-0.00371753860386348));
#84323=CARTESIAN_POINT('Ctrl Pts',(15.8194631574341,19.9998970680962,0.164270320263236));
#84324=CARTESIAN_POINT('Ctrl Pts',(15.7914668049778,20.0068523115617,0.332256642999523));
#84325=CARTESIAN_POINT('Ctrl Pts',(15.7634704525216,20.0208397482382,0.499642555985247));
#84326=CARTESIAN_POINT('Ctrl Pts',(15.7538530958715,20.0256447372934,0.557143261689614));
#84327=CARTESIAN_POINT('Ctrl Pts',(15.7442357392215,20.0312791241108,0.614573137971777));
#84328=CARTESIAN_POINT('Ctrl Pts',(15.7346183825714,20.037740393227,0.671908015611504));
#84329=CARTESIAN_POINT('Ctrl Pts',(15.7066973281163,20.0564987125248,0.838362302272619));
#84330=CARTESIAN_POINT('Ctrl Pts',(15.6787762736612,20.0822340439421,1.00404913498184));
#84331=CARTESIAN_POINT('Ctrl Pts',(15.6508552192062,20.1148584484018,1.16837875607722));
#84332=CARTESIAN_POINT('Ctrl Pts',(15.6229373718183,20.1474791055584,1.3326895019496));
#84333=CARTESIAN_POINT('Ctrl Pts',(15.5950195244303,20.1869871947943,1.49564303801235));
#84334=CARTESIAN_POINT('Ctrl Pts',(15.5671016770424,20.2332436180977,1.65665954009544));
#84335=CARTESIAN_POINT('Ctrl Pts',(15.5391812737269,20.2795042762573,1.81769078352007));
#84336=CARTESIAN_POINT('Ctrl Pts',(15.5112608704114,20.3325144183481,1.97678433460715));
#84337=CARTESIAN_POINT('Ctrl Pts',(15.4833404670958,20.3920847868941,2.13337454813151));
#84338=CARTESIAN_POINT('Ctrl Pts',(15.4554202348681,20.4516547904109,2.28996380211851));
#84339=CARTESIAN_POINT('Ctrl Pts',(15.4275000026403,20.5177848250248,2.44404945535309));
#84340=CARTESIAN_POINT('Ctrl Pts',(15.3995797704125,20.5902370265517,2.59508469439968));
#84341=CARTESIAN_POINT('Ctrl Pts',(15.3716534889113,20.6627049257695,2.74615265715181));
#84342=CARTESIAN_POINT('Ctrl Pts',(15.3437272074102,20.7414975912157,2.89416860115279));
#84343=CARTESIAN_POINT('Ctrl Pts',(15.315800925909,20.8263302876324,3.03860851498343));
#84344=CARTESIAN_POINT('Ctrl Pts',(15.3058070946255,20.8566889179167,3.09029846623458));
#84345=CARTESIAN_POINT('Ctrl Pts',(15.295813263342,20.887820653669,3.14153068128663));
#84346=CARTESIAN_POINT('Ctrl Pts',(15.2858194320586,20.9197110486647,3.19228196920965));
#84347=CARTESIAN_POINT('Ctrl Pts',(15.2578615192377,21.0089249705158,3.33425955949041));
#84348=CARTESIAN_POINT('Ctrl Pts',(15.2299036064168,21.1041081373684,3.4725170175672));
#84349=CARTESIAN_POINT('Ctrl Pts',(15.2019456935959,21.2049262970795,3.60655905033598));
#84350=CARTESIAN_POINT('Ctrl Pts',(15.1739930471236,21.3057254659747,3.74057583400706));
#84351=CARTESIAN_POINT('Ctrl Pts',(15.1460404006513,21.4121573208104,3.87037852614376));
#84352=CARTESIAN_POINT('Ctrl Pts',(15.118087754179,21.5238457096574,3.99550281805025));
#84353=CARTESIAN_POINT('Ctrl Pts',(15.090135879103,21.6355310162916,4.12062365695957));
#84354=CARTESIAN_POINT('Ctrl Pts',(15.062184004027,21.7524723605252,4.24106611711228));
#84355=CARTESIAN_POINT('Ctrl Pts',(15.0342321289509,21.8742544598873,4.3564003188688));
#84356=CARTESIAN_POINT('Ctrl Pts',(15.0062824307059,21.9960270751254,4.4717255386496));
#84357=CARTESIAN_POINT('Ctrl Pts',(14.9783327324608,22.1226394636412,4.58194307964691));
#84358=CARTESIAN_POINT('Ctrl Pts',(14.9503830342157,22.2536405425231,4.68666094521177));
#84359=CARTESIAN_POINT('Ctrl Pts',(14.9224304330414,22.384655227522,4.79138968704997));
#84360=CARTESIAN_POINT('Ctrl Pts',(14.8944778318671,22.5200592683346,4.89061741606617));
#84361=CARTESIAN_POINT('Ctrl Pts',(14.8665252306927,22.6593690919098,4.9839928908369));
#84362=CARTESIAN_POINT('Ctrl Pts',(14.8566903143104,22.7083842249757,5.01684636235471));
#84363=CARTESIAN_POINT('Ctrl Pts',(14.8468553979281,22.7578825927692,5.04897574751083));
#84364=CARTESIAN_POINT('Ctrl Pts',(14.8370204815457,22.8078422705463,5.0803670172822));
#84365=CARTESIAN_POINT('Ctrl Pts',(14.8090390532225,22.9499830970086,5.1696786627439));
#84366=CARTESIAN_POINT('Ctrl Pts',(14.7810576248992,23.0958875944494,5.25302957654209));
#84367=CARTESIAN_POINT('Ctrl Pts',(14.753076196576,23.2450373241744,5.33012013511967));
#84368=CARTESIAN_POINT('Ctrl Pts',(14.725097566022,23.3941721409177,5.40720298567058));
#84369=CARTESIAN_POINT('Ctrl Pts',(14.697118935468,23.5465512644704,5.47802658718934));
#84370=CARTESIAN_POINT('Ctrl Pts',(14.669140304914,23.7016321781138,5.54233753531108));
#84371=CARTESIAN_POINT('Ctrl Pts',(14.6411590636731,23.8567275623619,5.60665448428935));
#84372=CARTESIAN_POINT('Ctrl Pts',(14.6131778224323,24.0145249525328,5.66445744360224));
#84373=CARTESIAN_POINT('Ctrl Pts',(14.5851965811914,24.1744616792911,5.71554108021484));
#84374=CARTESIAN_POINT('Ctrl Pts',(14.557215631288,24.3343967408066,5.76662418495049));
#84375=CARTESIAN_POINT('Ctrl Pts',(14.5292346813846,24.496470795692,5.81098801437962));
#84376=CARTESIAN_POINT('Ctrl Pts',(14.5012537314812,24.6601055990544,5.8484769807459));
#84377=CARTESIAN_POINT('Ctrl Pts',(14.4732673595621,24.8237721107926,5.88597321154622));
#84378=CARTESIAN_POINT('Ctrl Pts',(14.445280987643,24.988999670261,5.91659184866194));
#84379=CARTESIAN_POINT('Ctrl Pts',(14.4172946157239,25.1551986321962,5.94022816472204));
#84380=CARTESIAN_POINT('Ctrl Pts',(14.4076035874936,25.2127494585993,5.94841287000867));
#84381=CARTESIAN_POINT('Ctrl Pts',(14.3979125592632,25.2704166874997,5.95576079462521));
#84382=CARTESIAN_POINT('Ctrl Pts',(14.3882215310329,25.3281756306374,5.96226903256895));
#84383=CARTESIAN_POINT('Ctrl Pts',(14.360344049786,25.4943266123377,5.98099081078627));
#84384=CARTESIAN_POINT('Ctrl Pts',(14.3324665685392,25.6612892760491,5.99276628493692));
#84385=CARTESIAN_POINT('Ctrl Pts',(14.3045890872924,25.8284713291035,5.99754765842345));
#84386=CARTESIAN_POINT('Ctrl Pts',(14.2767169872715,25.9956211107917,6.00232810895532));
#84387=CARTESIAN_POINT('Ctrl Pts',(14.2488448872507,26.1629898798038,6.00011714374974));
#84388=CARTESIAN_POINT('Ctrl Pts',(14.2209727872298,26.3299833962866,5.99091904119687));
#84389=CARTESIAN_POINT('Ctrl Pts',(14.1931009237254,26.4969754956996,5.98172101669706));
#84390=CARTESIAN_POINT('Ctrl Pts',(14.165229060221,26.6635920314603,5.96553598726662));
#84391=CARTESIAN_POINT('Ctrl Pts',(14.1373571967166,26.8292412520957,5.94242029360283));
#84392=CARTESIAN_POINT('Ctrl Pts',(14.1094870061456,26.9948805300838,5.91930598739617));
#84393=CARTESIAN_POINT('Ctrl Pts',(14.0816168155746,27.1595522944168,5.88926189348339));
#84394=CARTESIAN_POINT('Ctrl Pts',(14.0537466250035,27.3226721168271,5.85239595989269));
#84395=CARTESIAN_POINT('Ctrl Pts',(14.0258722195373,27.4858166083534,5.81552445095265));
#84396=CARTESIAN_POINT('Ctrl Pts',(13.997997814071,27.64740837908,5.7718291114696));
#84397=CARTESIAN_POINT('Ctrl Pts',(13.9701234086047,27.8068746389096,5.72146869599629));
#84398=CARTESIAN_POINT('Ctrl Pts',(13.9598897992432,27.8654199381597,5.70297973414695));
#84399=CARTESIAN_POINT('Ctrl Pts',(13.9496561898816,27.9236788860339,5.68359289742922));
#84400=CARTESIAN_POINT('Ctrl Pts',(13.9394225805201,27.9816236668422,5.66331772400341));
#84401=CARTESIAN_POINT('Ctrl Pts',(13.9112904383807,28.140913586199,5.60758137130876));
#84402=CARTESIAN_POINT('Ctrl Pts',(13.8831582962414,28.2978640435168,5.54511577331456));
#84403=CARTESIAN_POINT('Ctrl Pts',(13.8550261541021,28.4519117338169,5.47614178501354));
#84404=CARTESIAN_POINT('Ctrl Pts',(13.826897483734,28.6059404131814,5.40717630875217));
#84405=CARTESIAN_POINT('Ctrl Pts',(13.7987688133659,28.7570667621176,5.33170417045857));
#84406=CARTESIAN_POINT('Ctrl Pts',(13.7706401429978,28.9047485808636,5.24999387446985));
#84407=CARTESIAN_POINT('Ctrl Pts',(13.7425113164897,29.0524312193798,5.16828312491369));
#84408=CARTESIAN_POINT('Ctrl Pts',(13.7143824899816,29.196669021128,5.08033429409493));
#84409=CARTESIAN_POINT('Ctrl Pts',(13.6862536634735,29.3369447894087,4.98646161846638));
#84410=CARTESIAN_POINT('Ctrl Pts',(13.6581269842118,29.4772098495769,4.89259610871675));
#84411=CARTESIAN_POINT('Ctrl Pts',(13.63000030495,29.613513227398,4.79280782832254));
#84412=CARTESIAN_POINT('Ctrl Pts',(13.6018736256883,29.7453667698052,4.68745429413868));
#84413=CARTESIAN_POINT('Ctrl Pts',(13.5737453734725,29.8772276859791,4.58209486817239));
#84414=CARTESIAN_POINT('Ctrl Pts',(13.5456171212566,30.0046380308218,4.47116975696162));
#84415=CARTESIAN_POINT('Ctrl Pts',(13.5174888690408,30.1271421914849,4.35507719004676));
#84416=CARTESIAN_POINT('Ctrl Pts',(13.5085337893629,30.1661433534195,4.31811726168885));
#84417=CARTESIAN_POINT('Ctrl Pts',(13.4995787096851,30.2046475017216,4.28063387251699));
#84418=CARTESIAN_POINT('Ctrl Pts',(13.4906236300072,30.2426406871193,4.24264068711928));
#84419=CARTESIAN_POINT('Ctrl Pts',(13.4906236300072,30.2426406871193,4.24264068711928));
#84420=CARTESIAN_POINT('Ctrl Pts',(13.4626987432741,30.3611159477566,4.12416542648202));
#84421=CARTESIAN_POINT('Ctrl Pts',(13.4347738565409,30.4746378485994,4.00071215862355));
#84422=CARTESIAN_POINT('Ctrl Pts',(13.4068489698078,30.5828001512623,3.8727177503131));
#84423=CARTESIAN_POINT('Ctrl Pts',(13.3789270160111,30.6909510936942,3.74473678518955));
#84424=CARTESIAN_POINT('Ctrl Pts',(13.3510050622145,30.7937433583066,3.61221587243848));
#84425=CARTESIAN_POINT('Ctrl Pts',(13.3230831084178,30.8908103894018,3.47562566093063));
#84426=CARTESIAN_POINT('Ctrl Pts',(13.2951582521442,30.9878875105796,3.3390212509199));
#84427=CARTESIAN_POINT('Ctrl Pts',(13.2672333958706,31.0792380244218,3.1983469524618));
#84428=CARTESIAN_POINT('Ctrl Pts',(13.2393085395969,31.1645377465886,3.05410377427835));
#84429=CARTESIAN_POINT('Ctrl Pts',(13.2113836703494,31.2498375083858,2.90986052907932));
#84430=CARTESIAN_POINT('Ctrl Pts',(13.1834588011019,31.3290863152131,2.76204867382277));
#84431=CARTESIAN_POINT('Ctrl Pts',(13.1555339318543,31.4020050250242,2.61119545603423));
#84432=CARTESIAN_POINT('Ctrl Pts',(13.1276027931589,31.4749401059074,2.46030836999807));
#84433=CARTESIAN_POINT('Ctrl Pts',(13.0996716544635,31.5415421141224,2.30637884152955));
#84434=CARTESIAN_POINT('Ctrl Pts',(13.071740515768,31.6015789666553,2.14995652986867));
#84435=CARTESIAN_POINT('Ctrl Pts',(13.0617685703435,31.6230132598808,2.09411080255781));
#84436=CARTESIAN_POINT('Ctrl Pts',(13.0517966249189,31.6436111889962,2.03794752238453));
#84437=CARTESIAN_POINT('Ctrl Pts',(13.0418246794944,31.6633636970422,1.98149227478286));
#84438=CARTESIAN_POINT('Ctrl Pts',(13.0138239706077,31.7188277217667,1.82296884871973));
#84439=CARTESIAN_POINT('Ctrl Pts',(12.9858232617211,31.7676392622126,1.66209389997174));
#84440=CARTESIAN_POINT('Ctrl Pts',(12.9578225528345,31.80961969565,1.49943955927409));
#84441=CARTESIAN_POINT('Ctrl Pts',(12.9298265555361,31.8515930651763,1.3368125878935));
#84442=CARTESIAN_POINT('Ctrl Pts',(12.9018305582378,31.8867375438694,1.17240712404193));
#84443=CARTESIAN_POINT('Ctrl Pts',(12.8738345609394,31.9149248777071,1.00680866657069));
#84444=CARTESIAN_POINT('Ctrl Pts',(12.8458389183366,31.943111854425,0.841212307151039));
#84445=CARTESIAN_POINT('Ctrl Pts',(12.8178432757339,31.9643418070086,0.674423291268812));
#84446=CARTESIAN_POINT('Ctrl Pts',(12.7898476331311,31.9785378059958,0.507036194248846));
#84447=CARTESIAN_POINT('Ctrl Pts',(12.761854040854,31.9927327653063,0.339661356210217));
#84448=CARTESIAN_POINT('Ctrl Pts',(12.7338604485769,31.9998947750089,0.171688835431475));
#84449=CARTESIAN_POINT('Ctrl Pts',(12.7058668562998,31.9999988483255,0.00371753859988222));
#84450=CARTESIAN_POINT('Ctrl Pts',(12.6778705038436,32.0001029319037,-0.164270320267365));
#84451=CARTESIAN_POINT('Ctrl Pts',(12.6498741513873,31.9931476884381,-0.33225664300379));
#84452=CARTESIAN_POINT('Ctrl Pts',(12.621877798931,31.9791602517615,-0.49964255598965));
#84453=CARTESIAN_POINT('Ctrl Pts',(12.6122604422812,31.9743552627063,-0.557143261692545));
#84454=CARTESIAN_POINT('Ctrl Pts',(12.6026430856314,31.9687208758891,-0.614573137973243));
#84455=CARTESIAN_POINT('Ctrl Pts',(12.5930257289816,31.962259606773,-0.671908015611506));
#84456=CARTESIAN_POINT('Ctrl Pts',(12.5651046745265,31.9435012874752,-0.838362302272481));
#84457=CARTESIAN_POINT('Ctrl Pts',(12.5371836200715,31.9177659560579,-1.00404913498156));
#84458=CARTESIAN_POINT('Ctrl Pts',(12.5092625656164,31.8851415515983,-1.16837875607681));
#84459=CARTESIAN_POINT('Ctrl Pts',(12.4813447182285,31.8525208944417,-1.33268950194925));
#84460=CARTESIAN_POINT('Ctrl Pts',(12.4534268708406,31.8130128052057,-1.49564303801208));
#84461=CARTESIAN_POINT('Ctrl Pts',(12.4255090234527,31.7667563819023,-1.65665954009523));
#84462=CARTESIAN_POINT('Ctrl Pts',(12.3975886201371,31.7204957237428,-1.81769078351988));
#84463=CARTESIAN_POINT('Ctrl Pts',(12.3696682168216,31.667485581652,-1.97678433460697));
#84464=CARTESIAN_POINT('Ctrl Pts',(12.3417478135061,31.607915213106,-2.13337454813135));
#84465=CARTESIAN_POINT('Ctrl Pts',(12.3138275812784,31.5483452095893,-2.28996380211801));
#84466=CARTESIAN_POINT('Ctrl Pts',(12.2859073490507,31.4822151749755,-2.44404945535227));
#84467=CARTESIAN_POINT('Ctrl Pts',(12.2579871168229,31.4097629734489,-2.59508469439855));
#84468=CARTESIAN_POINT('Ctrl Pts',(12.2300608353218,31.3372950742311,-2.74615265715067));
#84469=CARTESIAN_POINT('Ctrl Pts',(12.2021345538206,31.2585024087849,-2.89416860115163));
#84470=CARTESIAN_POINT('Ctrl Pts',(12.1742082723194,31.1736697123683,-3.03860851498227));
#84471=CARTESIAN_POINT('Ctrl Pts',(12.1642144410358,31.1433110820838,-3.09029846623381));
#84472=CARTESIAN_POINT('Ctrl Pts',(12.1542206097523,31.1121793463313,-3.14153068128624));
#84473=CARTESIAN_POINT('Ctrl Pts',(12.1442267784688,31.0802889513353,-3.19228196920963));
#84474=CARTESIAN_POINT('Ctrl Pts',(12.1158381645934,30.9897006589988,-3.33644677204223));
#84475=CARTESIAN_POINT('Ctrl Pts',(12.087449550718,30.8929631649647,-3.47676763811165));
#84476=CARTESIAN_POINT('Ctrl Pts',(12.0590609368427,30.7904223170505,-3.6127349784207));
#84477=CARTESIAN_POINT('Ctrl Pts',(12.0306784629411,30.6879036469758,-3.74867291130908));
#84478=CARTESIAN_POINT('Ctrl Pts',(12.0022959890396,30.5795843045573,-3.88025896473511));
#84479=CARTESIAN_POINT('Ctrl Pts',(11.9739135151381,30.4658519791244,-4.00701461197116));
#84480=CARTESIAN_POINT('Ctrl Pts',(11.9558847780552,30.3936084460142,-4.08753064611678));
#84481=CARTESIAN_POINT('Ctrl Pts',(11.9378560409723,30.3191816788964,-4.16609830040219));
#84482=CARTESIAN_POINT('Ctrl Pts',(11.9198273038894,30.2426793568795,-4.24260201700657));
#84483=CARTESIAN_POINT('',(11.6421188053765,30.2426406871193,4.24264068711929));
#84484=CARTESIAN_POINT('Ctrl Pts',(10.0713224779131,30.2426823068249,-4.24259906700533));
#84485=CARTESIAN_POINT('Ctrl Pts',(10.099702075706,30.3631070273837,-4.12217198371286));
#84486=CARTESIAN_POINT('Ctrl Pts',(10.1280816734989,30.4783868213669,-3.99662894535352));
#84487=CARTESIAN_POINT('Ctrl Pts',(10.1564612712918,30.5881087732421,-3.86642701791961));
#84488=CARTESIAN_POINT('Ctrl Pts',(10.1848494148972,30.6978637651638,-3.73618588340214));
#84489=CARTESIAN_POINT('Ctrl Pts',(10.2132375585026,30.8020573826946,-3.60128328063448));
#84490=CARTESIAN_POINT('Ctrl Pts',(10.2416257021081,30.900316749403,-3.46220966371485));
#84491=CARTESIAN_POINT('Ctrl Pts',(10.259657786018,30.9627308744707,-3.37387042023291));
#84492=CARTESIAN_POINT('Ctrl Pts',(10.277689869928,31.0227514918882,-3.28384892384956));
#84493=CARTESIAN_POINT('Ctrl Pts',(10.295721953838,31.0802919954162,-3.19227712476694));
#84494=CARTESIAN_POINT('Ctrl Pts',(10.3236482024984,31.1694048465757,-3.05046008108918));
#84495=CARTESIAN_POINT('Ctrl Pts',(10.3515744511589,31.2525905179036,-2.90488583932461));
#84496=CARTESIAN_POINT('Ctrl Pts',(10.3795006998193,31.3295481080712,-2.75606911447355));
#84497=CARTESIAN_POINT('Ctrl Pts',(10.4074214795192,31.406490627184,-2.60728153327165));
#84498=CARTESIAN_POINT('Ctrl Pts',(10.4353422592191,31.4772073541776,-2.45525301625694));
#84499=CARTESIAN_POINT('Ctrl Pts',(10.463263038919,31.5414434661153,-2.30052261711299));
#84500=CARTESIAN_POINT('Ctrl Pts',(10.4911830300089,31.6056777637326,-2.14579658826009));
#84501=CARTESIAN_POINT('Ctrl Pts',(10.5191030210989,31.6634316878239,-1.98836911978285));
#84502=CARTESIAN_POINT('Ctrl Pts',(10.5470230121888,31.714498403278,-1.82879960600742));
#84503=CARTESIAN_POINT('Ctrl Pts',(10.5749408954179,31.7655612633752,-1.66924213916772));
#84504=CARTESIAN_POINT('Ctrl Pts',(10.6028587786469,31.8099378283379,-1.50754325092965));
#84505=CARTESIAN_POINT('Ctrl Pts',(10.630776661876,31.8474709253391,-1.34427816217983));
#84506=CARTESIAN_POINT('Ctrl Pts',(10.6586977788765,31.8850083698569,-1.18099416218284));
#84507=CARTESIAN_POINT('Ctrl Pts',(10.686618895877,31.9157006919787,-1.01614390674221));
#84508=CARTESIAN_POINT('Ctrl Pts',(10.7145400128776,31.9394415348614,-0.850314208962638));
#84509=CARTESIAN_POINT('Ctrl Pts',(10.7245336433687,31.9479389460255,-0.79095982410671));
#84510=CARTESIAN_POINT('Ctrl Pts',(10.7345272738598,31.9555462855579,-0.731480047082945));
#84511=CARTESIAN_POINT('Ctrl Pts',(10.7445209043508,31.9622602820985,-0.671902022999215));
#84512=CARTESIAN_POINT('Ctrl Pts',(10.7725171760834,31.9810689494521,-0.504999459108853));
#84513=CARTESIAN_POINT('Ctrl Pts',(10.8005134478159,31.992866802328,-0.337291560570467));
#84514=CARTESIAN_POINT('Ctrl Pts',(10.8285097195484,31.9976088364781,-0.169376044941714));
#84515=CARTESIAN_POINT('Ctrl Pts',(10.8565031923509,32.0023503965428,-0.00147731668325168));
#84516=CARTESIAN_POINT('Ctrl Pts',(10.8844966651534,32.0000375374273,0.166628675507197));
#84517=CARTESIAN_POINT('Ctrl Pts',(10.9124901379559,31.9906773440968,0.334342577194388));
#84518=CARTESIAN_POINT('Ctrl Pts',(10.9404860813889,31.9813163246602,0.502071280870899));
#84519=CARTESIAN_POINT('Ctrl Pts',(10.9684820248219,31.9649067431905,0.669407513281637));
#84520=CARTESIAN_POINT('Ctrl Pts',(10.9964779682549,31.9415077390088,0.835754621463946));
#84521=CARTESIAN_POINT('Ctrl Pts',(11.0244735000281,31.9181090788924,1.00209928363357));
#84522=CARTESIAN_POINT('Ctrl Pts',(11.0524690318012,31.8877212475795,1.16745454211118));
#84523=CARTESIAN_POINT('Ctrl Pts',(11.0804645635743,31.850454962582,1.331231283737));
#84524=CARTESIAN_POINT('Ctrl Pts',(11.1084652302525,31.8131818422495,1.49503806508595));
#84525=CARTESIAN_POINT('Ctrl Pts',(11.1364658969307,31.7690278175163,1.65726544707923));
#84526=CARTESIAN_POINT('Ctrl Pts',(11.1644665636089,31.7181543781866,1.81733610188789));
#84527=CARTESIAN_POINT('Ctrl Pts',(11.1740843273605,31.7006801970778,1.87231771211886));
#84528=CARTESIAN_POINT('Ctrl Pts',(11.1837020911121,31.6824136882439,1.92704499564975));
#84529=CARTESIAN_POINT('Ctrl Pts',(11.1933198548636,31.663362748889,1.98149498472647));
#84530=CARTESIAN_POINT('Ctrl Pts',(11.2212515038255,31.6080355268652,2.13962716806498));
#84531=CARTESIAN_POINT('Ctrl Pts',(11.2491831527874,31.5460718260323,2.29546734104631));
#84532=CARTESIAN_POINT('Ctrl Pts',(11.2771148017493,31.4776864184661,2.44845900536477));
#84533=CARTESIAN_POINT('Ctrl Pts',(11.3050407969019,31.4093148531923,2.60141970174108));
#84534=CARTESIAN_POINT('Ctrl Pts',(11.3329667920545,31.3345243036091,2.75153275242724));
#84535=CARTESIAN_POINT('Ctrl Pts',(11.3608927872071,31.2535773064315,2.89826249421055));
#84536=CARTESIAN_POINT('Ctrl Pts',(11.3888176576472,31.1726335693742,3.04498632648999));
#84537=CARTESIAN_POINT('Ctrl Pts',(11.4167425280873,31.0855340292351,3.18832684446721));
#84538=CARTESIAN_POINT('Ctrl Pts',(11.4446673985274,30.9925870510111,3.32777321013268));
#84539=CARTESIAN_POINT('Ctrl Pts',(11.4725899484745,30.8996477964689,3.4672079881233));
#84540=CARTESIAN_POINT('Ctrl Pts',(11.5005124984216,30.8008622501275,3.60274899853689));
#84541=CARTESIAN_POINT('Ctrl Pts',(11.5284350483687,30.6965821281744,3.73391434198922));
#84542=CARTESIAN_POINT('Ctrl Pts',(11.5563604727484,30.5922912713068,3.86509318800296));
#84543=CARTESIAN_POINT('Ctrl Pts',(11.5842858971281,30.4825049047961,3.99189522028912));
#84544=CARTESIAN_POINT('Ctrl Pts',(11.6122113215079,30.3676155040598,4.11387102480096));
#84545=CARTESIAN_POINT('Ctrl Pts',(11.6221804827974,30.3266008734198,4.15741544697571));
#84546=CARTESIAN_POINT('Ctrl Pts',(11.632149644087,30.2849362564227,4.20034511781583));
#84547=CARTESIAN_POINT('Ctrl Pts',(11.6421188053765,30.2426406871193,4.24264068711928));
#84548=CARTESIAN_POINT('',(14.7837115023615,21.757359307712,-4.24264069228803));
#84549=CARTESIAN_POINT('Ctrl Pts',(11.6421188053765,30.2426406871193,4.24264068711928));
#84550=CARTESIAN_POINT('Ctrl Pts',(11.6702475126086,30.1233006893401,4.36198068489844));
#84551=CARTESIAN_POINT('Ctrl Pts',(11.6983762198408,29.998916654682,4.47628793832936));
#84552=CARTESIAN_POINT('Ctrl Pts',(11.7265049270729,29.8699330958604,4.58515188773117));
#84553=CARTESIAN_POINT('Ctrl Pts',(11.7546318617202,29.7409576651872,4.69400897686061));
#84554=CARTESIAN_POINT('Ctrl Pts',(11.7827587963674,29.6073835226446,4.79742325031584));
#84555=CARTESIAN_POINT('Ctrl Pts',(11.8108857310146,29.4696888345521,4.8950239418602));
#84556=CARTESIAN_POINT('Ctrl Pts',(11.8390153212383,29.3319811461531,4.99263384827642));
#84557=CARTESIAN_POINT('Ctrl Pts',(11.8671449114621,29.1901523828211,5.08442889782491));
#84558=CARTESIAN_POINT('Ctrl Pts',(11.8952745016858,29.0447109805536,5.17008075806332));
#84559=CARTESIAN_POINT('Ctrl Pts',(11.9234033963947,28.8992731743799,5.25573050052698));
#84560=CARTESIAN_POINT('Ctrl Pts',(11.9515322911036,28.7502231720558,5.33523720429525));
#84561=CARTESIAN_POINT('Ctrl Pts',(11.9796611858125,28.5980956536292,5.40831757338576));
#84562=CARTESIAN_POINT('Ctrl Pts',(12.0077937407229,28.445948339993,5.48140745187494));
#84563=CARTESIAN_POINT('Ctrl Pts',(12.0359262956333,28.2907229855743,5.54806919311709));
#84564=CARTESIAN_POINT('Ctrl Pts',(12.0640588505436,28.13297671343,5.60806654204151));
#84565=CARTESIAN_POINT('Ctrl Pts',(12.0730118189922,28.0827751799437,5.62716023522472));
#84566=CARTESIAN_POINT('Ctrl Pts',(12.0819647874408,28.0323184841005,5.64557933645482));
#84567=CARTESIAN_POINT('Ctrl Pts',(12.0909177558893,27.9816249837632,5.66331726320586));
#84568=CARTESIAN_POINT('Ctrl Pts',(12.1187917955891,27.8237965887412,5.71854226229868));
#84569=CARTESIAN_POINT('Ctrl Pts',(12.1466658352889,27.663636190809,5.76717319154767));
#84570=CARTESIAN_POINT('Ctrl Pts',(12.1745398749887,27.5017110346811,5.80903296326652));
#84571=CARTESIAN_POINT('Ctrl Pts',(12.2024098801815,27.3398093157074,5.85088667617435));
#84572=CARTESIAN_POINT('Ctrl Pts',(12.2302798853744,27.176143655898,5.88597110800216));
#84573=CARTESIAN_POINT('Ctrl Pts',(12.2581498905672,27.0112946476869,5.91415954600145));
#84574=CARTESIAN_POINT('Ctrl Pts',(12.2860216549733,26.8464352338608,5.94234976331403));
#84575=CARTESIAN_POINT('Ctrl Pts',(12.3138934193793,26.6803926351711,5.96364306054548));
#84576=CARTESIAN_POINT('Ctrl Pts',(12.3417651837853,26.5137565026141,5.97796405609986));
#84577=CARTESIAN_POINT('Ctrl Pts',(12.3696364306319,26.3471234643744,5.99228478572329));
#84578=CARTESIAN_POINT('Ctrl Pts',(12.3975076774786,26.1798972311815,5.99963344784168));
#84579=CARTESIAN_POINT('Ctrl Pts',(12.4253789243253,26.0126716424776,5.99998661910816));
#84580=CARTESIAN_POINT('Ctrl Pts',(12.4532560715852,25.845410651695,6.0003398651419));
#84581=CARTESIAN_POINT('Ctrl Pts',(12.4811332188451,25.6781506235587,5.99369466172538));
#84582=CARTESIAN_POINT('Ctrl Pts',(12.509010366105,25.5114852337302,5.98007970876112));
#84583=CARTESIAN_POINT('Ctrl Pts',(12.5192458128707,25.4502919305069,5.97508080679371));
#84584=CARTESIAN_POINT('Ctrl Pts',(12.5294812596364,25.3891787604038,5.96914283018179));
#84585=CARTESIAN_POINT('Ctrl Pts',(12.5397167064021,25.3281749595449,5.96226895695067));
#84586=CARTESIAN_POINT('Ctrl Pts',(12.567703083318,25.1613746817244,5.94347399748075));
#84587=CARTESIAN_POINT('Ctrl Pts',(12.5956894602339,24.9953398077307,5.91767244072533));
#84588=CARTESIAN_POINT('Ctrl Pts',(12.6236758371498,24.8306627399789,5.88495117841487));
#84589=CARTESIAN_POINT('Ctrl Pts',(12.6516572680958,24.6660147752372,5.85223569885995));
#84590=CARTESIAN_POINT('Ctrl Pts',(12.6796386990419,24.5027244443468,5.8126030152568));
#84591=CARTESIAN_POINT('Ctrl Pts',(12.7076201299879,24.341374370111,5.76619120562919));
#84592=CARTESIAN_POINT('Ctrl Pts',(12.735600998011,24.1800275418727,5.71978032970193));
#84593=CARTESIAN_POINT('Ctrl Pts',(12.7635818660341,24.0206211936116,5.66659068357758));
#84594=CARTESIAN_POINT('Ctrl Pts',(12.7915627340573,23.8637238777225,5.60681053089786));
#84595=CARTESIAN_POINT('Ctrl Pts',(12.8195414707123,23.7068385130682,5.54703493181191));
#84596=CARTESIAN_POINT('Ctrl Pts',(12.8475202073674,23.5524620907059,5.48066994143202));
#84597=CARTESIAN_POINT('Ctrl Pts',(12.8754989440225,23.401144546287,5.40795250817776));
#84598=CARTESIAN_POINT('Ctrl Pts',(12.9034804347397,23.2498121070596,5.3352279170474));
#84599=CARTESIAN_POINT('Ctrl Pts',(12.931461925457,23.1015394291952,5.25614976907973));
#84600=CARTESIAN_POINT('Ctrl Pts',(12.9594434161742,22.9568538160383,5.17100196316335));
#84601=CARTESIAN_POINT('Ctrl Pts',(12.9691341630878,22.9067452755995,5.1415129753992));
#84602=CARTESIAN_POINT('Ctrl Pts',(12.9788249100014,22.8570667564696,5.11129638076749));
#84603=CARTESIAN_POINT('Ctrl Pts',(12.988515656915,22.8078394319705,5.08036523371278));
#84604=CARTESIAN_POINT('Ctrl Pts',(13.0164680731131,22.6658459741917,4.99114607406818));
#84605=CARTESIAN_POINT('Ctrl Pts',(13.0444204893112,22.5275810196469,4.89596132380272));
#84606=CARTESIAN_POINT('Ctrl Pts',(13.0723729055094,22.3935386215211,4.79514716411706));
#84607=CARTESIAN_POINT('Ctrl Pts',(13.1003223822074,22.2595103194088,4.69434360613489));
#84608=CARTESIAN_POINT('Ctrl Pts',(13.1282718589055,22.1297039381378,4.5879120092559));
#84609=CARTESIAN_POINT('Ctrl Pts',(13.1562213356036,22.0045823550702,4.47623031607892));
#84610=CARTESIAN_POINT('Ctrl Pts',(13.1841734808165,21.879448825847,4.36453795993828));
#84611=CARTESIAN_POINT('Ctrl Pts',(13.2121256260294,21.7590012245333,4.24759471320073));
#84612=CARTESIAN_POINT('Ctrl Pts',(13.2400777712423,21.6436678730077,4.12581754314647));
#84613=CARTESIAN_POINT('Ctrl Pts',(13.2680297331437,21.5283352778435,4.00404117171243));
#84614=CARTESIAN_POINT('Ctrl Pts',(13.2959816950452,21.4181170792243,3.87743117038718));
#84615=CARTESIAN_POINT('Ctrl Pts',(13.3239336569466,21.3134035364645,3.7464401220327));
#84616=CARTESIAN_POINT('Ctrl Pts',(13.3518914166417,21.2086682740303,3.61542190352579));
#84617=CARTESIAN_POINT('Ctrl Pts',(13.3798491763368,21.1094401440338,3.48002106836329));
#84618=CARTESIAN_POINT('Ctrl Pts',(13.4078069360319,21.0160685245648,3.34072253384904));
#84619=CARTESIAN_POINT('Ctrl Pts',(13.4176428264972,20.9832192179079,3.29171556253219));
#84620=CARTESIAN_POINT('Ctrl Pts',(13.4274787169625,20.9510943985716,3.24222643678125));
#84621=CARTESIAN_POINT('Ctrl Pts',(13.4373146074278,20.9197080045838,3.19227712476694));
#84622=CARTESIAN_POINT('Ctrl Pts',(13.4652408560882,20.8305951534243,3.05046008108928));
#84623=CARTESIAN_POINT('Ctrl Pts',(13.4931671047486,20.7474094820965,2.90488583932483));
#84624=CARTESIAN_POINT('Ctrl Pts',(13.521093353409,20.670451891929,2.75606911447389));
#84625=CARTESIAN_POINT('Ctrl Pts',(13.5490141331088,20.5935093728166,2.60728153327268));
#84626=CARTESIAN_POINT('Ctrl Pts',(13.5769349128086,20.5227926458232,2.45525301625869));
#84627=CARTESIAN_POINT('Ctrl Pts',(13.6048556925083,20.4585565338858,2.30052261711549));
#84628=CARTESIAN_POINT('Ctrl Pts',(13.6327756835982,20.3943222362684,2.14579658826282));
#84629=CARTESIAN_POINT('Ctrl Pts',(13.6606956746882,20.3365683121772,1.98836911978582));
#84630=CARTESIAN_POINT('Ctrl Pts',(13.6886156657781,20.285501596723,1.82879960601062));
#84631=CARTESIAN_POINT('Ctrl Pts',(13.716533549007,20.2344387366259,1.66924213917137));
#84632=CARTESIAN_POINT('Ctrl Pts',(13.744451432236,20.1900621716632,1.50754325093376));
#84633=CARTESIAN_POINT('Ctrl Pts',(13.772369315465,20.1525290746619,1.3442781621844));
#84634=CARTESIAN_POINT('Ctrl Pts',(13.8002904324655,20.114991630144,1.18099416218751));
#84635=CARTESIAN_POINT('Ctrl Pts',(13.828211549466,20.0842993080221,1.01614390674698));
#84636=CARTESIAN_POINT('Ctrl Pts',(13.8561326664665,20.0605584651393,0.850314208967497));
#84637=CARTESIAN_POINT('Ctrl Pts',(13.8661262969579,20.0520610539749,0.790959824109951));
#84638=CARTESIAN_POINT('Ctrl Pts',(13.8761199274493,20.0444537144423,0.731480047084558));
#84639=CARTESIAN_POINT('Ctrl Pts',(13.8861135579406,20.0377397179015,0.671902022999197));
#84640=CARTESIAN_POINT('Ctrl Pts',(13.9141098296732,20.0189310505478,0.504999459108637));
#84641=CARTESIAN_POINT('Ctrl Pts',(13.9421061014057,20.007133197672,0.337291560570052));
#84642=CARTESIAN_POINT('Ctrl Pts',(13.9701023731383,20.0023911635219,0.169376044941101));
#84643=CARTESIAN_POINT('Ctrl Pts',(13.9980958459408,19.9976496034572,0.00147731668254816));
#84644=CARTESIAN_POINT('Ctrl Pts',(14.0260893187433,19.9999624625727,-0.166628675507993));
#84645=CARTESIAN_POINT('Ctrl Pts',(14.0540827915458,20.0093226559032,-0.334342577195271));
#84646=CARTESIAN_POINT('Ctrl Pts',(14.0820787349788,20.0186836753399,-0.502071280871779));
#84647=CARTESIAN_POINT('Ctrl Pts',(14.1100746784119,20.0350932568096,-0.669407513282511));
#84648=CARTESIAN_POINT('Ctrl Pts',(14.1380706218449,20.0584922609913,-0.835754621464816));
#84649=CARTESIAN_POINT('Ctrl Pts',(14.166066153618,20.0818909211078,-1.00209928363457));
#84650=CARTESIAN_POINT('Ctrl Pts',(14.1940616853912,20.1122787524207,-1.1674545421123));
#84651=CARTESIAN_POINT('Ctrl Pts',(14.2220572171643,20.1495450374183,-1.33123128373824));
#84652=CARTESIAN_POINT('Ctrl Pts',(14.2500578838426,20.1868181577509,-1.49503806508736));
#84653=CARTESIAN_POINT('Ctrl Pts',(14.2780585505208,20.2309721824841,-1.65726544708081));
#84654=CARTESIAN_POINT('Ctrl Pts',(14.3060592171991,20.2818456218139,-1.81733610188963));
#84655=CARTESIAN_POINT('Ctrl Pts',(14.3156769809505,20.2993198029226,-1.87231771212));
#84656=CARTESIAN_POINT('Ctrl Pts',(14.325294744702,20.3175863117563,-1.92704499565031));
#84657=CARTESIAN_POINT('Ctrl Pts',(14.3349125084534,20.336637251111,-1.98149498472645));
#84658=CARTESIAN_POINT('Ctrl Pts',(14.3628441574153,20.3919644731347,-2.13962716806488));
#84659=CARTESIAN_POINT('Ctrl Pts',(14.3907758063772,20.4539281739677,-2.29546734104614));
#84660=CARTESIAN_POINT('Ctrl Pts',(14.418707455339,20.5223135815338,-2.44845900536453));
#84661=CARTESIAN_POINT('Ctrl Pts',(14.4466334504916,20.5906851468074,-2.60141970174059));
#84662=CARTESIAN_POINT('Ctrl Pts',(14.4745594456442,20.6654756963905,-2.75153275242649));
#84663=CARTESIAN_POINT('Ctrl Pts',(14.5024854407967,20.7464226935679,-2.89826249420958));
#84664=CARTESIAN_POINT('Ctrl Pts',(14.5304103112368,20.8273664306252,-3.04498632648893));
#84665=CARTESIAN_POINT('Ctrl Pts',(14.5583351816769,20.9144659707642,-3.18832684446607));
#84666=CARTESIAN_POINT('Ctrl Pts',(14.586260052117,21.0074129489881,-3.32777321013146));
#84667=CARTESIAN_POINT('Ctrl Pts',(14.614182602064,21.10035220353,-3.46720798812171));
#84668=CARTESIAN_POINT('Ctrl Pts',(14.642105152011,21.1991377498711,-3.60274899853495));
#84669=CARTESIAN_POINT('Ctrl Pts',(14.670027701958,21.3034178718238,-3.73391434198695));
#84670=CARTESIAN_POINT('Ctrl Pts',(14.6979531263377,21.4077087286912,-3.86509318800059));
#84671=CARTESIAN_POINT('Ctrl Pts',(14.7258785507174,21.5174950952018,-3.99189522028667));
#84672=CARTESIAN_POINT('Ctrl Pts',(14.7538039750971,21.6323844959379,-4.11387102479843));
#84673=CARTESIAN_POINT('Ctrl Pts',(14.7637731363868,21.6733991265786,-4.15741544697404));
#84674=CARTESIAN_POINT('Ctrl Pts',(14.7737422976766,21.7150637435764,-4.200345117815));
#84675=CARTESIAN_POINT('Ctrl Pts',(14.7837114589663,21.7573593128807,-4.24264068711927));
#84676=CARTESIAN_POINT('Ctrl Pts',(14.7837115517867,21.7573593128807,-4.24264068711927));
#84677=CARTESIAN_POINT('Ctrl Pts',(14.8118396368998,21.8766966712322,-4.36197804547074));
#84678=CARTESIAN_POINT('Ctrl Pts',(14.8399677220128,22.0010778773211,-4.47628291578594));
#84679=CARTESIAN_POINT('Ctrl Pts',(14.8680958071259,22.130058445085,-4.58514474815595));
#84680=CARTESIAN_POINT('Ctrl Pts',(14.8962221107649,22.2590308439481,-4.69399968583229));
#84681=CARTESIAN_POINT('Ctrl Pts',(14.9243484144039,22.3926017892773,-4.7974120773116));
#84682=CARTESIAN_POINT('Ctrl Pts',(14.9524747180429,22.5302931406659,-4.89501116549187));
#84683=CARTESIAN_POINT('Ctrl Pts',(14.9806036705035,22.6679974592694,-4.99261944515966));
#84684=CARTESIAN_POINT('Ctrl Pts',(15.0087326229641,22.8098227113067,-5.08441314936828));
#84685=CARTESIAN_POINT('Ctrl Pts',(15.0368615754247,22.9552604861664,-5.17006395443035));
#84686=CARTESIAN_POINT('Ctrl Pts',(15.064989830364,23.1006946545664,-5.25571263558638));
#84687=CARTESIAN_POINT('Ctrl Pts',(15.0931180853034,23.2497409024661,-5.33521856906017));
#84688=CARTESIAN_POINT('Ctrl Pts',(15.1212463402428,23.4018645747706,-5.40829846737105));
#84689=CARTESIAN_POINT('Ctrl Pts',(15.1493782575177,23.5540080537758,-5.48138788078008));
#84690=CARTESIAN_POINT('Ctrl Pts',(15.1775101747925,23.7092294822999,-5.54804945550753));
#84691=CARTESIAN_POINT('Ctrl Pts',(15.2056420920674,23.8669717619628,-5.60804694485841));
#84692=CARTESIAN_POINT('Ctrl Pts',(15.2145982288115,23.9171909280855,-5.62714787259382));
#84693=CARTESIAN_POINT('Ctrl Pts',(15.2235543655555,23.96766544203,-5.64557373131554));
#84694=CARTESIAN_POINT('Ctrl Pts',(15.2325105022996,24.018376925954,-5.66331793142573));
#84695=CARTESIAN_POINT('Ctrl Pts',(15.2603850114755,24.1762081163835,-5.71854384890847));
#84696=CARTESIAN_POINT('Ctrl Pts',(15.2882595206514,24.3363713158732,-5.76717543811175));
#84697=CARTESIAN_POINT('Ctrl Pts',(15.3161340298273,24.4982992551085,-5.80903562330205));
#84698=CARTESIAN_POINT('Ctrl Pts',(15.3440045203059,24.6602038490224,-5.85088977346538));
#84699=CARTESIAN_POINT('Ctrl Pts',(15.3718750107844,24.8238723673531,-5.88597438845085));
#84700=CARTESIAN_POINT('Ctrl Pts',(15.399745501263,24.9887241948697,-5.91416276796285));
#84701=CARTESIAN_POINT('Ctrl Pts',(15.4276177702719,25.1535865422579,-5.94235294629101));
#84702=CARTESIAN_POINT('Ctrl Pts',(15.4554900392808,25.3196320369453,-5.96364595333837));
#84703=CARTESIAN_POINT('Ctrl Pts',(15.4833623082898,25.4862710064242,-5.9779664202101));
#84704=CARTESIAN_POINT('Ctrl Pts',(15.5112340698435,25.6529069419985,-5.99228662635691));
#84705=CARTESIAN_POINT('Ctrl Pts',(15.5391058313972,25.8201360139034,-5.99963452146785));
#84706=CARTESIAN_POINT('Ctrl Pts',(15.566977592951,25.9873643627478,-5.99998669504118));
#84707=CARTESIAN_POINT('Ctrl Pts',(15.594855266211,26.1546281813588,-6.00033894331185));
#84708=CARTESIAN_POINT('Ctrl Pts',(15.622732939471,26.32189095874,-5.99369250574667));
#84709=CARTESIAN_POINT('Ctrl Pts',(15.650610612731,26.4885590004376,-5.98007609509204));
#84710=CARTESIAN_POINT('Ctrl Pts',(15.6608435594248,26.5497371759023,-5.97507797336611));
#84711=CARTESIAN_POINT('Ctrl Pts',(15.6710765061185,26.6108352473121,-5.96914124102974));
#84712=CARTESIAN_POINT('Ctrl Pts',(15.6813094528123,26.6718240007242,-5.96226907410684));
#84713=CARTESIAN_POINT('Ctrl Pts',(15.7092958108749,26.8386237644539,-5.94347420202107));
#84714=CARTESIAN_POINT('Ctrl Pts',(15.7372821689374,27.004658163261,-5.91767277224285));
#84715=CARTESIAN_POINT('Ctrl Pts',(15.765268527,27.1693347969323,-5.88495166782899));
#84716=CARTESIAN_POINT('Ctrl Pts',(15.79324993121,27.3339822812672,-5.85223635536303));
#84717=CARTESIAN_POINT('Ctrl Pts',(15.8212313354199,27.4972721736021,-5.81260387364708));
#84718=CARTESIAN_POINT('Ctrl Pts',(15.8492127396299,27.6586218525161,-5.76619229217652));
#84719=CARTESIAN_POINT('Ctrl Pts',(15.8771935699863,27.8199682224078,-5.71978166253284));
#84720=CARTESIAN_POINT('Ctrl Pts',(15.9051744003426,27.9793741570644,-5.66659229425009));
#84721=CARTESIAN_POINT('Ctrl Pts',(15.933155230699,28.1362711049113,-5.60681244258456));
#84722=CARTESIAN_POINT('Ctrl Pts',(15.9611339235647,28.2931560672036,-5.54703715757685));
#84723=CARTESIAN_POINT('Ctrl Pts',(15.9891126164303,28.447532133851,-5.480672507322));
#84724=CARTESIAN_POINT('Ctrl Pts',(16.017091309296,28.5988493692395,-5.40795543213917));
#84725=CARTESIAN_POINT('Ctrl Pts',(16.0450727479037,28.7501814544316,-5.33523122072833));
#84726=CARTESIAN_POINT('Ctrl Pts',(16.0730541865114,28.8984538267661,-5.25615347420067));
#84727=CARTESIAN_POINT('Ctrl Pts',(16.1010356251191,29.0431391823601,-5.17100608361514));
#84728=CARTESIAN_POINT('Ctrl Pts',(16.1107265511878,29.0932486532825,-5.14151663960646));
#84729=CARTESIAN_POINT('Ctrl Pts',(16.1204174772565,29.1429280911377,-5.11129956078575));
#84730=CARTESIAN_POINT('Ctrl Pts',(16.1301084033251,29.1921563212657,-5.0803679020917));
#84731=CARTESIAN_POINT('Ctrl Pts',(16.1581991428504,29.334852424818,-4.99070741337258));
#84732=CARTESIAN_POINT('Ctrl Pts',(16.1862898823756,29.4737818985722,-4.89502292008477));
#84733=CARTESIAN_POINT('Ctrl Pts',(16.2143806219008,29.6084459130554,-4.79365393959071));
#84734=CARTESIAN_POINT('Ctrl Pts',(16.2424694201627,29.7431006213289,-4.69229196439055));
#84735=CARTESIAN_POINT('Ctrl Pts',(16.2705582184246,29.8734902121934,-4.58524646945369));
#84736=CARTESIAN_POINT('Ctrl Pts',(16.2986470166865,29.9991469388092,-4.4728988096997));
#84737=CARTESIAN_POINT('Ctrl Pts',(16.317267303762,30.0824457791775,-4.39842265527768));
#84738=CARTESIAN_POINT('Ctrl Pts',(16.3358875908376,30.1636654206877,-4.32161733901386));
#84739=CARTESIAN_POINT('Ctrl Pts',(16.3545078779131,30.2426778921868,-4.24260348172551));
#84740=CARTESIAN_POINT('Origin',(-31.4159265358979,26.,7.7715611723761E-15));
#84741=CARTESIAN_POINT('',(17.341,31.8790943677938,1.19843623717527));
#84742=CARTESIAN_POINT('Ctrl Pts',(16.354507877922,30.2426778922245,-4.24260348168784));
#84743=CARTESIAN_POINT('Ctrl Pts',(16.382888439425,30.3631066642285,-4.12217259749732));
#84744=CARTESIAN_POINT('Ctrl Pts',(16.4112690009281,30.4783901528095,-3.99662544639589));
#84745=CARTESIAN_POINT('Ctrl Pts',(16.4396495624311,30.5881154211411,-3.86641912915385));
#84746=CARTESIAN_POINT('Ctrl Pts',(16.4680386771246,30.6978737579205,-3.73617357098893));
#84747=CARTESIAN_POINT('Ctrl Pts',(16.4964277918181,30.8020703391995,-3.6012662649802));
#84748=CARTESIAN_POINT('Ctrl Pts',(16.5248169065115,30.9003322675621,-3.46218769963297));
#84749=CARTESIAN_POINT('Ctrl Pts',(16.5428470556204,30.9627391879337,-3.37385781340274));
#84750=CARTESIAN_POINT('Ctrl Pts',(16.5608772047292,31.0227531159613,-3.28384605151104));
#84751=CARTESIAN_POINT('Ctrl Pts',(16.578907353838,31.080287476321,-3.1922843165884));
#84752=CARTESIAN_POINT('Ctrl Pts',(16.6068336288268,31.1694004591925,-3.05046750894783));
#84753=CARTESIAN_POINT('Ctrl Pts',(16.6347599038155,31.2525863029309,-2.90489345895294));
#84754=CARTESIAN_POINT('Ctrl Pts',(16.6626861788043,31.3295440951455,-2.75607687445397));
#84755=CARTESIAN_POINT('Ctrl Pts',(16.6906069725765,31.4064867825055,-2.60728949886027));
#84756=CARTESIAN_POINT('Ctrl Pts',(16.7185277663487,31.4772037128205,-2.45526113889313));
#84757=CARTESIAN_POINT('Ctrl Pts',(16.746448560121,31.5414400514461,-2.30053084226862));
#84758=CARTESIAN_POINT('Ctrl Pts',(16.7743685472131,31.6056745341725,-2.14580501607051));
#84759=CARTESIAN_POINT('Ctrl Pts',(16.8022885343052,31.6634286751131,-1.98837769921453));
#84760=CARTESIAN_POINT('Ctrl Pts',(16.8302085213973,31.7144956270484,-1.82880828094286));
#84761=CARTESIAN_POINT('Ctrl Pts',(16.8581263901798,31.765558704497,-1.66925096931824));
#84762=CARTESIAN_POINT('Ctrl Pts',(16.8860442589624,31.8099355114292,-1.50755218178439));
#84763=CARTESIAN_POINT('Ctrl Pts',(16.9139621277449,31.8474688624454,-1.34428713552236));
#84764=CARTESIAN_POINT('Ctrl Pts',(16.9418832151492,31.8850065406423,-1.18100326660467));
#84765=CARTESIAN_POINT('Ctrl Pts',(16.9698043025534,31.9156991159039,-1.01615308570994));
#84766=CARTESIAN_POINT('Ctrl Pts',(16.9977253899577,31.9394402185479,-0.850323403356513));
#84767=CARTESIAN_POINT('Ctrl Pts',(17.0077190280888,31.9479377381903,-0.790968915731159));
#84768=CARTESIAN_POINT('Ctrl Pts',(17.0177126662198,31.9555451837976,-0.731489027925986));
#84769=CARTESIAN_POINT('Ctrl Pts',(17.0277063043508,31.9622592833946,-0.671910885144261));
#84770=CARTESIAN_POINT('Ctrl Pts',(17.0556074415748,31.9810043101541,-0.505575270875629));
#84771=CARTESIAN_POINT('Ctrl Pts',(17.0835085787988,31.9927864702583,-0.338435950515601));
#84772=CARTESIAN_POINT('Ctrl Pts',(17.1114097160228,31.9975602832382,-0.171086670796819));
#84773=CARTESIAN_POINT('Ctrl Pts',(17.1393069093683,32.0023334214305,-0.00376104621528817));
#84774=CARTESIAN_POINT('Ctrl Pts',(17.1672041027137,32.0001001819432,0.163774162066368));
#84775=CARTESIAN_POINT('Ctrl Pts',(17.1951012960592,31.9908671824224,0.330923560016396));
#84776=CARTESIAN_POINT('Ctrl Pts',(17.2230008709851,31.9816333946815,0.498087227492853));
#84777=CARTESIAN_POINT('Ctrl Pts',(17.250900445911,31.9653986681724,0.664864702559548));
#84778=CARTESIAN_POINT('Ctrl Pts',(17.278800020837,31.9422216809555,0.830663285803638));
#84779=CARTESIAN_POINT('Ctrl Pts',(17.2995333472246,31.9249979045387,0.95387506054006));
#84780=CARTESIAN_POINT('Ctrl Pts',(17.3202666736123,31.903941282576,1.0765462673785));
#84781=CARTESIAN_POINT('Ctrl Pts',(17.341,31.8790943677938,1.19843623717527));
#84782=CARTESIAN_POINT('Origin',(17.341,26.,7.7715611723761E-15));
#84783=CARTESIAN_POINT('Origin',(-17.341,26.,-5.55111512312578E-14));
#84784=CARTESIAN_POINT('',(-17.341094308639,36.2772926947297,2.14768526278092));
#84785=CARTESIAN_POINT('',(-17.341,31.8402307203765,5.84023072037652));
#84786=CARTESIAN_POINT('Ctrl Pts',(-17.341,36.2776062547427,2.14782924427302));
#84787=CARTESIAN_POINT('Ctrl Pts',(-17.341,36.1615316286314,2.33343382237898));
#84788=CARTESIAN_POINT('Ctrl Pts',(-17.341,36.0393803151467,2.51488353100729));
#84789=CARTESIAN_POINT('Ctrl Pts',(-17.341,35.9113297455572,2.6918644841006));
#84790=CARTESIAN_POINT('Ctrl Pts',(-17.341,35.785655731614,2.86556075767459));
#84791=CARTESIAN_POINT('Ctrl Pts',(-17.341,35.6542987314585,3.03495263305023));
#84792=CARTESIAN_POINT('Ctrl Pts',(-17.341,35.5174264520561,3.19969356394901));
#84793=CARTESIAN_POINT('Ctrl Pts',(-17.341,35.3824035821343,3.36220852593145));
#84794=CARTESIAN_POINT('Ctrl Pts',(-17.341,35.2420128499351,3.52019737874567));
#84795=CARTESIAN_POINT('Ctrl Pts',(-17.341,35.0964247300032,3.67327830325533));
#84796=CARTESIAN_POINT('Ctrl Pts',(-17.341,34.954049320268,3.82298117296687));
#84797=CARTESIAN_POINT('Ctrl Pts',(-17.341,34.8067028384009,3.96799019837233));
#84798=CARTESIAN_POINT('Ctrl Pts',(-17.341,34.6545622767166,4.10790209060223));
#84799=CARTESIAN_POINT('Ctrl Pts',(-17.341,34.550707649757,4.20340914811465));
#84800=CARTESIAN_POINT('Ctrl Pts',(-17.341,34.444619466998,4.29654011779324));
#84801=CARTESIAN_POINT('Ctrl Pts',(-17.341,34.3363608382622,4.38715446085138));
#84802=CARTESIAN_POINT('Ctrl Pts',(-17.341,34.3064917774342,4.41215538092857));
#84803=CARTESIAN_POINT('Ctrl Pts',(-17.341,34.2764559097218,4.43696598947311));
#84804=CARTESIAN_POINT('Ctrl Pts',(-17.341,34.2462598533269,4.46157896982436));
#84805=CARTESIAN_POINT('Ctrl Pts',(-17.341,34.2238656295209,4.47983263127309));
#84806=CARTESIAN_POINT('Ctrl Pts',(-17.341,34.201386247286,4.49797519500983));
#84807=CARTESIAN_POINT('Ctrl Pts',(-17.341,34.1788257701953,4.51600289953751));
#84808=CARTESIAN_POINT('Ctrl Pts',(-17.341,34.0263322655447,4.63785793980052));
#84809=CARTESIAN_POINT('Ctrl Pts',(-17.341,33.8700735855436,4.75451722463535));
#84810=CARTESIAN_POINT('Ctrl Pts',(-17.341,33.7102131419073,4.86568485778385));
#84811=CARTESIAN_POINT('Ctrl Pts',(-17.341,33.5537632563168,4.97448077434605));
#84812=CARTESIAN_POINT('Ctrl Pts',(-17.341,33.3938630916286,5.07801666714861));
#84813=CARTESIAN_POINT('Ctrl Pts',(-17.341,33.2306846425595,5.17596932344744));
#84814=CARTESIAN_POINT('Ctrl Pts',(-17.341,33.0697047439569,5.27260223526146));
#84815=CARTESIAN_POINT('Ctrl Pts',(-17.341,32.905533764824,5.36380114677409));
#84816=CARTESIAN_POINT('Ctrl Pts',(-17.341,32.7383634686604,5.44921344499573));
#84817=CARTESIAN_POINT('Ctrl Pts',(-17.341,32.5748642160718,5.5327500973891));
#84818=CARTESIAN_POINT('Ctrl Pts',(-17.341,32.408495487699,5.61075117905066));
#84819=CARTESIAN_POINT('Ctrl Pts',(-17.341,32.2394694502253,5.68284993327241));
#84820=CARTESIAN_POINT('Ctrl Pts',(-17.341,32.1079590152306,5.73894625234844));
#84821=CARTESIAN_POINT('Ctrl Pts',(-17.341,31.9748405139997,5.79146876643761));
#84822=CARTESIAN_POINT('Ctrl Pts',(-17.341,31.8402307203765,5.84023072037652));
#84823=CARTESIAN_POINT('',(-17.341,22.5935394840313,-9.9320706176077));
#84824=CARTESIAN_POINT('Ctrl Pts',(-17.341,22.5935394840313,-9.9320706176077));
#84825=CARTESIAN_POINT('Ctrl Pts',(-17.341,22.8358088333483,-10.0151631573662));
#84826=CARTESIAN_POINT('Ctrl Pts',(-17.341,23.080781809034,-10.0890669438635));
#84827=CARTESIAN_POINT('Ctrl Pts',(-17.341,23.3279547104505,-10.1538369902452));
#84828=CARTESIAN_POINT('Ctrl Pts',(-17.341,23.5907422034553,-10.2226987384906));
#84829=CARTESIAN_POINT('Ctrl Pts',(-17.341,23.8560168656464,-10.2812369185677));
#84830=CARTESIAN_POINT('Ctrl Pts',(-17.341,24.1231943750741,-10.3294578205659));
#84831=CARTESIAN_POINT('Ctrl Pts',(-17.341,24.3779390436958,-10.3754348106445));
#84832=CARTESIAN_POINT('Ctrl Pts',(-17.341,24.6344143202987,-10.4120320079489));
#84833=CARTESIAN_POINT('Ctrl Pts',(-17.341,24.8921223713494,-10.4392020733278));
#84834=CARTESIAN_POINT('Ctrl Pts',(-17.341,25.0304094986267,-10.4537816344779));
#84835=CARTESIAN_POINT('Ctrl Pts',(-17.341,25.1690516819469,-10.4656458282875));
#84836=CARTESIAN_POINT('Ctrl Pts',(-17.341,25.3079720394225,-10.4747811465506));
#84837=CARTESIAN_POINT('Ctrl Pts',(-17.341,25.3442642541695,-10.4771677005317));
#84838=CARTESIAN_POINT('Ctrl Pts',(-17.341,25.3805764111684,-10.4793680417995));
#84839=CARTESIAN_POINT('Ctrl Pts',(-17.341,25.4169041904599,-10.4813817179015));
#84840=CARTESIAN_POINT('Ctrl Pts',(-17.341,25.5258995833598,-10.4874234144263));
#84841=CARTESIAN_POINT('Ctrl Pts',(-17.341,25.6349403439897,-10.4917796357836));
#84842=CARTESIAN_POINT('Ctrl Pts',(-17.341,25.7439841375295,-10.4944519751268));
#84843=CARTESIAN_POINT('Ctrl Pts',(-17.341,26.0159511590823,-10.501117078643));
#84844=CARTESIAN_POINT('Ctrl Pts',(-17.341,26.2879465285844,-10.4973124016406));
#84845=CARTESIAN_POINT('Ctrl Pts',(-17.341,26.559393029141,-10.4830228194042));
#84846=CARTESIAN_POINT('Ctrl Pts',(-17.341,26.8181381329473,-10.4694018685668));
#84847=CARTESIAN_POINT('Ctrl Pts',(-17.341,27.0763852070207,-10.4462538416015));
#84848=CARTESIAN_POINT('Ctrl Pts',(-17.341,27.3335713168633,-10.4136535248962));
#84849=CARTESIAN_POINT('Ctrl Pts',(-17.341,27.6028277744426,-10.3795231988167));
#84850=CARTESIAN_POINT('Ctrl Pts',(-17.341,27.8709222300644,-10.3350328829493));
#84851=CARTESIAN_POINT('Ctrl Pts',(-17.341,28.1371965948931,-10.2802081881677));
#84852=CARTESIAN_POINT('Ctrl Pts',(-17.341,28.1827018784682,-10.2708388548316));
#84853=CARTESIAN_POINT('Ctrl Pts',(-17.341,28.2281549242296,-10.2611673443991));
#84854=CARTESIAN_POINT('Ctrl Pts',(-17.341,28.2735493716128,-10.2511942711831));
#84855=CARTESIAN_POINT('Ctrl Pts',(-17.341,28.3081605165915,-10.2435902688687));
#84856=CARTESIAN_POINT('Ctrl Pts',(-17.341,28.3427305407739,-10.235812482136));
#84857=CARTESIAN_POINT('Ctrl Pts',(-17.341,28.3772488537953,-10.2278633236637));
#84858=CARTESIAN_POINT('Ctrl Pts',(-17.341,28.6304099297094,-10.1695633276522));
#84859=CARTESIAN_POINT('Ctrl Pts',(-17.341,28.8809513566271,-10.1020141715181));
#84860=CARTESIAN_POINT('Ctrl Pts',(-17.341,29.1283233348882,-10.0253414139435));
#84861=CARTESIAN_POINT('Ctrl Pts',(-17.341,29.3750732479331,-9.94886146501217));
#84862=CARTESIAN_POINT('Ctrl Pts',(-17.341,29.6186702931669,-9.86330361846533));
#84863=CARTESIAN_POINT('Ctrl Pts',(-17.341,29.8585620425732,-9.76874141915599));
#84864=CARTESIAN_POINT('Ctrl Pts',(-17.341,30.0573570415716,-9.6903790229356));
#84865=CARTESIAN_POINT('Ctrl Pts',(-17.341,30.2536075928598,-9.60583221153325));
#84866=CARTESIAN_POINT('Ctrl Pts',(-17.341,30.4469909186711,-9.51511701868236));
#84867=CARTESIAN_POINT('Ctrl Pts',(-17.341,30.6809973108109,-9.40534573978716));
#84868=CARTESIAN_POINT('Ctrl Pts',(-17.341,30.9108063750555,-9.28654330808442));
#84869=CARTESIAN_POINT('Ctrl Pts',(-17.341,31.1360653900894,-9.15912023482861));
#84870=CARTESIAN_POINT('Ctrl Pts',(-17.341,31.3624225939535,-9.03107594516669));
#84871=CARTESIAN_POINT('Ctrl Pts',(-17.341,31.5841857695078,-8.89432631678317));
#84872=CARTESIAN_POINT('Ctrl Pts',(-17.341,31.8009651035927,-8.74924628711789));
#84873=CARTESIAN_POINT('Ctrl Pts',(-17.341,31.8443517478387,-8.72020968332513));
#84874=CARTESIAN_POINT('Ctrl Pts',(-17.341,31.8875386396169,-8.69083926973578));
#84875=CARTESIAN_POINT('Ctrl Pts',(-17.341,31.930522473861,-8.6611378774681));
#84876=CARTESIAN_POINT('Ctrl Pts',(-17.341,31.9566250905296,-8.64310123484369));
#84877=CARTESIAN_POINT('Ctrl Pts',(-17.341,31.9826551439777,-8.62494089745138));
#84878=CARTESIAN_POINT('Ctrl Pts',(-17.341,32.0086040372382,-8.6066630275424));
#84879=CARTESIAN_POINT('Ctrl Pts',(-17.341,32.0559898745325,-8.57328541251676));
#84880=CARTESIAN_POINT('Ctrl Pts',(-17.341,32.1030883056765,-8.5395277586763));
#84881=CARTESIAN_POINT('Ctrl Pts',(-17.341,32.1498919137234,-8.50539854264918));
#84882=CARTESIAN_POINT('Ctrl Pts',(-17.341,32.3589826980336,-8.3529294308696));
#84883=CARTESIAN_POINT('Ctrl Pts',(-17.341,32.5622213807345,-8.19302739276201));
#84884=CARTESIAN_POINT('Ctrl Pts',(-17.341,32.7592977225623,-8.02615983750127));
#84885=CARTESIAN_POINT('Ctrl Pts',(-17.341,32.9580802244621,-7.85784765039154));
#84886=CARTESIAN_POINT('Ctrl Pts',(-17.341,33.1505937118948,-7.682448388491));
#84887=CARTESIAN_POINT('Ctrl Pts',(-17.341,33.3364921131307,-7.50039575408498));
#84888=CARTESIAN_POINT('Ctrl Pts',(-17.341,33.5226147373004,-7.31812353534938));
#84889=CARTESIAN_POINT('Ctrl Pts',(-17.341,33.7021067751131,-7.12918140070557));
#84890=CARTESIAN_POINT('Ctrl Pts',(-17.341,33.8745861108141,-6.9339657231966));
#84891=CARTESIAN_POINT('Ctrl Pts',(-17.341,34.0459474637866,-6.74001540164983));
#84892=CARTESIAN_POINT('Ctrl Pts',(-17.341,34.2103871455161,-6.53987209449813));
#84893=CARTESIAN_POINT('Ctrl Pts',(-17.341,34.3674895883909,-6.33389361035062));
#84894=CARTESIAN_POINT('Ctrl Pts',(-17.341,34.517366833392,-6.13738815080077));
#84895=CARTESIAN_POINT('Ctrl Pts',(-17.341,34.6605662781383,-5.93557133757178));
#84896=CARTESIAN_POINT('Ctrl Pts',(-17.341,34.7966867681353,-5.72873359083955));
#84897=CARTESIAN_POINT('Ctrl Pts',(-17.341,34.8194088706324,-5.6942069117067));
#84898=CARTESIAN_POINT('Ctrl Pts',(-17.341,34.8419351844103,-5.65953767929054));
#84899=CARTESIAN_POINT('Ctrl Pts',(-17.341,34.8642455796673,-5.62475603283737));
#84900=CARTESIAN_POINT('Ctrl Pts',(-17.341,35.0050863633287,-5.40518689087187));
#84901=CARTESIAN_POINT('Ctrl Pts',(-17.341,35.137490961629,-5.18089281592262));
#84902=CARTESIAN_POINT('Ctrl Pts',(-17.341,35.2611152866583,-4.95229237399867));
#84903=CARTESIAN_POINT('Ctrl Pts',(-17.341,35.3838450176568,-4.72534617439922));
#84904=CARTESIAN_POINT('Ctrl Pts',(-17.341,35.4979214784785,-4.49415518369225));
#84905=CARTESIAN_POINT('Ctrl Pts',(-17.341,35.6029675828494,-4.25909790208043));
#84906=CARTESIAN_POINT('Ctrl Pts',(-17.341,35.6765857757336,-4.0943655457481));
#84907=CARTESIAN_POINT('Ctrl Pts',(-17.341,35.7457679170749,-3.9277336259582));
#84908=CARTESIAN_POINT('Ctrl Pts',(-17.341,35.8103706829352,-3.75932527825395));
#84909=CARTESIAN_POINT('Ctrl Pts',(-17.341,35.9028113585593,-3.51834826689536));
#84910=CARTESIAN_POINT('Ctrl Pts',(-17.341,35.9858779941333,-3.27373439840514));
#84911=CARTESIAN_POINT('Ctrl Pts',(-17.341,36.0596175129558,-3.02603073497669));
#84912=CARTESIAN_POINT('Ctrl Pts',(-17.341,36.1201532965813,-2.82268067774835));
#84913=CARTESIAN_POINT('Ctrl Pts',(-17.341,36.1744021874915,-2.61724776464813));
#84914=CARTESIAN_POINT('Ctrl Pts',(-17.341,36.222364326136,-2.41002990804256));
#84915=CARTESIAN_POINT('Ctrl Pts',(-17.341,36.243347761793,-2.31937209577762));
#84916=CARTESIAN_POINT('Ctrl Pts',(-17.341,36.2631275735294,-2.2283726039198));
#84917=CARTESIAN_POINT('Ctrl Pts',(-17.341,36.2817023711122,-2.13705632026244));
#84918=CARTESIAN_POINT('Ctrl Pts',(-17.341,36.2945135782287,-2.07407464749687));
#84919=CARTESIAN_POINT('Ctrl Pts',(-17.341,36.3067515439926,-2.01094227700125));
#84920=CARTESIAN_POINT('Ctrl Pts',(-17.341,36.3184155754271,-1.94766738554708));
#84921=CARTESIAN_POINT('Ctrl Pts',(-17.341,36.3246021142257,-1.91410672745434));
#84922=CARTESIAN_POINT('Ctrl Pts',(-17.341,36.3306268079126,-1.88050770831468));
#84923=CARTESIAN_POINT('Ctrl Pts',(-17.341,36.3364864178808,-1.84689081480382));
#84924=CARTESIAN_POINT('Ctrl Pts',(-17.341,36.380510407315,-1.59432284991413));
#84925=CARTESIAN_POINT('Ctrl Pts',(-17.341,36.4152740876249,-1.34045762649642));
#84926=CARTESIAN_POINT('Ctrl Pts',(-17.341,36.4408913376544,-1.08583872086898));
#84927=CARTESIAN_POINT('Ctrl Pts',(-17.341,36.4669799578256,-0.82653470073817));
#84928=CARTESIAN_POINT('Ctrl Pts',(-17.341,36.4835825777201,-0.566448386721993));
#84929=CARTESIAN_POINT('Ctrl Pts',(-17.341,36.4907673755878,-0.306138836329885));
#84930=CARTESIAN_POINT('Ctrl Pts',(-17.341,36.4979550685448,-0.0457243951114861));
#84931=CARTESIAN_POINT('Ctrl Pts',(-17.341,36.4957173304509,0.214914140407855));
#84932=CARTESIAN_POINT('Ctrl Pts',(-17.341,36.4840701763494,0.475222111787335));
#84933=CARTESIAN_POINT('Ctrl Pts',(-17.341,36.4724300591827,0.735372811253935));
#84934=CARTESIAN_POINT('Ctrl Pts',(-17.341,36.451391878011,0.995194022519522));
#84935=CARTESIAN_POINT('Ctrl Pts',(-17.341,36.4209197011799,1.25412700844002));
#84936=CARTESIAN_POINT('Ctrl Pts',(-17.341,36.3904475243488,1.51305999436052));
#84937=CARTESIAN_POINT('Ctrl Pts',(-17.341,36.350541354477,1.77110543783372));
#84938=CARTESIAN_POINT('Ctrl Pts',(-17.341,36.3011134072668,2.02768932866362));
#84939=CARTESIAN_POINT('Ctrl Pts',(-17.341,36.2934016269672,2.06772171329963));
#84940=CARTESIAN_POINT('Ctrl Pts',(-17.341,36.285457960639,2.10771847797819));
#84941=CARTESIAN_POINT('Ctrl Pts',(-17.341,36.2772819608986,2.14767739224408));
#84942=CARTESIAN_POINT('',(-17.3410000124526,19.8194155612307,-6.18058438813164));
#84943=CARTESIAN_POINT('Origin',(-17.3410000000001,27.3621811742135,-4.63182998232183));
#84944=CARTESIAN_POINT('Ctrl Pts',(-17.341,20.0176003675788,-0.459232662172889));
#84945=CARTESIAN_POINT('Ctrl Pts',(-17.341,19.9517322064179,-0.581001446356886));
#84946=CARTESIAN_POINT('Ctrl Pts',(-17.341,19.8905997935081,-0.705156493938228));
#84947=CARTESIAN_POINT('Ctrl Pts',(-17.341,19.8341231382621,-0.831315420025));
#84948=CARTESIAN_POINT('Ctrl Pts',(-17.341,19.775995155109,-0.961163122553425));
#84949=CARTESIAN_POINT('Ctrl Pts',(-17.341,19.7227985260101,-1.09313356461186));
#84950=CARTESIAN_POINT('Ctrl Pts',(-17.341,19.6744339467518,-1.22686438721676));
#84951=CARTESIAN_POINT('Ctrl Pts',(-17.341,19.6385288680426,-1.32614397953659));
#84952=CARTESIAN_POINT('Ctrl Pts',(-17.341,19.6052866062593,-1.42639494775124));
#84953=CARTESIAN_POINT('Ctrl Pts',(-17.341,19.574665475194,-1.52748750025652));
#84954=CARTESIAN_POINT('Ctrl Pts',(-17.341,19.5542445293948,-1.59490517764461));
#84955=CARTESIAN_POINT('Ctrl Pts',(-17.341,19.5349891052483,-1.66269819855154));
#84956=CARTESIAN_POINT('Ctrl Pts',(-17.341,19.516887615846,-1.73082984977366));
#84957=CARTESIAN_POINT('Ctrl Pts',(-17.341,19.5050712366903,-1.7753051636802));
#84958=CARTESIAN_POINT('Ctrl Pts',(-17.341,19.4937484932404,-1.81991806378669));
#84959=CARTESIAN_POINT('Ctrl Pts',(-17.341,19.4829189525045,-1.86464426777467));
#84960=CARTESIAN_POINT('Ctrl Pts',(-17.341,19.4469174164301,-2.01333127912788));
#84961=CARTESIAN_POINT('Ctrl Pts',(-17.341,19.4163550630892,-2.16330885224486));
#84962=CARTESIAN_POINT('Ctrl Pts',(-17.341,19.3910863712414,-2.31419943608681));
#84963=CARTESIAN_POINT('Ctrl Pts',(-17.341,19.3651542274392,-2.46905178626642));
#84964=CARTESIAN_POINT('Ctrl Pts',(-17.341,19.3447967764344,-2.62486586549222));
#84965=CARTESIAN_POINT('Ctrl Pts',(-17.341,19.3298623828192,-2.781288963794));
#84966=CARTESIAN_POINT('Ctrl Pts',(-17.341,19.317433960963,-2.91146447033498));
#84967=CARTESIAN_POINT('Ctrl Pts',(-17.341,19.3087612989332,-3.04206287948856));
#84968=CARTESIAN_POINT('Ctrl Pts',(-17.341,19.3037641109837,-3.17290743017106));
#84969=CARTESIAN_POINT('Ctrl Pts',(-17.341,19.3019398254421,-3.22067385889559));
#84970=CARTESIAN_POINT('Ctrl Pts',(-17.341,19.3006054749907,-3.2684782057861));
#84971=CARTESIAN_POINT('Ctrl Pts',(-17.341,19.2997576672998,-3.31628153991435));
#84972=CARTESIAN_POINT('Ctrl Pts',(-17.341,19.2967922872302,-3.48348343700968));
#84973=CARTESIAN_POINT('Ctrl Pts',(-17.341,19.2997749992745,-3.65073112523236));
#84974=CARTESIAN_POINT('Ctrl Pts',(-17.341,19.3085060414163,-3.81763388962603));
#84975=CARTESIAN_POINT('Ctrl Pts',(-17.341,19.3174019514415,-3.9876882715531));
#84976=CARTESIAN_POINT('Ctrl Pts',(-17.341,19.3322648327157,-4.15738486193371));
#84977=CARTESIAN_POINT('Ctrl Pts',(-17.341,19.3528972700962,-4.32636292421868));
#84978=CARTESIAN_POINT('Ctrl Pts',(-17.341,19.3741185543832,-4.50016359700939));
#84979=CARTESIAN_POINT('Ctrl Pts',(-17.341,19.4014428903213,-4.67320444045425));
#84980=CARTESIAN_POINT('Ctrl Pts',(-17.341,19.4346780013984,-4.84514365891977));
#84981=CARTESIAN_POINT('Ctrl Pts',(-17.341,19.4683919621552,-5.01956016832891));
#84982=CARTESIAN_POINT('Ctrl Pts',(-17.341,19.5081877984253,-5.19284357814337));
#84983=CARTESIAN_POINT('Ctrl Pts',(-17.341,19.5538951091161,-5.36468229142512));
#84984=CARTESIAN_POINT('Ctrl Pts',(-17.341,19.6004418917034,-5.53967703748047));
#84985=CARTESIAN_POINT('Ctrl Pts',(-17.341,19.6531188357664,-5.71317409403076));
#84986=CARTESIAN_POINT('Ctrl Pts',(-17.341,19.7117841117731,-5.88488284291019));
#84987=CARTESIAN_POINT('Ctrl Pts',(-17.341,19.7456696241611,-5.98406313035338));
#84988=CARTESIAN_POINT('Ctrl Pts',(-17.341,19.781553769508,-6.08264744949897));
#84989=CARTESIAN_POINT('Ctrl Pts',(-17.341,19.8194156939928,-6.18058430600717));
#84990=CARTESIAN_POINT('Ctrl Pts',(-17.341,31.8402307203765,5.84023072037652));
#84991=CARTESIAN_POINT('Ctrl Pts',(-17.341,31.6772449817606,5.89927176683509));
#84992=CARTESIAN_POINT('Ctrl Pts',(-17.341,31.5124860737517,5.95267777531149));
#84993=CARTESIAN_POINT('Ctrl Pts',(-17.341,31.3462177804631,6.00028119451195));
#84994=CARTESIAN_POINT('Ctrl Pts',(-17.341,31.1839939581346,6.04672666205036));
#84995=CARTESIAN_POINT('Ctrl Pts',(-17.341,31.0203328080484,6.0876479752421));
#84996=CARTESIAN_POINT('Ctrl Pts',(-17.341,30.8555135488753,6.12285427372568));
#84997=CARTESIAN_POINT('Ctrl Pts',(-17.341,30.6932702801199,6.15751032651596));
#84998=CARTESIAN_POINT('Ctrl Pts',(-17.341,30.5299043691695,6.18662820695463));
#84999=CARTESIAN_POINT('Ctrl Pts',(-17.341,30.3657226044152,6.20999729895849));
#85000=CARTESIAN_POINT('Ctrl Pts',(-17.341,30.2057956270301,6.23276077853254));
#85001=CARTESIAN_POINT('Ctrl Pts',(-17.341,30.0450942444858,6.25006910703489));
#85002=CARTESIAN_POINT('Ctrl Pts',(-17.341,29.8839459666204,6.26170670088772));
#85003=CARTESIAN_POINT('Ctrl Pts',(-17.341,29.7384970744284,6.27221053720602));
#85004=CARTESIAN_POINT('Ctrl Pts',(-17.341,29.5926844366067,6.27809422970468));
#85005=CARTESIAN_POINT('Ctrl Pts',(-17.341,29.4467839047476,6.27918890117428));
#85006=CARTESIAN_POINT('Ctrl Pts',(-17.341,29.4214408789879,6.27937904638416));
#85007=CARTESIAN_POINT('Ctrl Pts',(-17.341,29.3960942595598,6.2794246753895));
#85008=CARTESIAN_POINT('Ctrl Pts',(-17.341,29.3707487936054,6.27932489687429));
#85009=CARTESIAN_POINT('Ctrl Pts',(-17.341,29.2195272607711,6.27872957698387));
#85010=CARTESIAN_POINT('Ctrl Pts',(-17.341,29.0685973566615,6.27296155917988));
#85011=CARTESIAN_POINT('Ctrl Pts',(-17.341,28.9182153028243,6.26188279249635));
#85012=CARTESIAN_POINT('Ctrl Pts',(-17.341,28.771341749382,6.25106249985473));
#85013=CARTESIAN_POINT('Ctrl Pts',(-17.341,28.6249904852149,6.23517583557146));
#85014=CARTESIAN_POINT('Ctrl Pts',(-17.341,28.4794453702235,6.21407478427408));
#85015=CARTESIAN_POINT('Ctrl Pts',(-17.341,28.3707028106173,6.19830934736062));
#85016=CARTESIAN_POINT('Ctrl Pts',(-17.341,28.2624111412361,6.17963269235642));
#85017=CARTESIAN_POINT('Ctrl Pts',(-17.341,28.1547072927676,6.15797858226784));
#85018=CARTESIAN_POINT('Ctrl Pts',(-17.341,28.0155058302988,6.12999180337691));
#85019=CARTESIAN_POINT('Ctrl Pts',(-17.341,27.877284360162,6.09703110233222));
#85020=CARTESIAN_POINT('Ctrl Pts',(-17.341,27.7404123010864,6.05902908146687));
#85021=CARTESIAN_POINT('Ctrl Pts',(-17.341,27.6071004973527,6.02201555232658));
#85022=CARTESIAN_POINT('Ctrl Pts',(-17.341,27.4750687666256,5.98021902236883));
#85023=CARTESIAN_POINT('Ctrl Pts',(-17.341,27.3447076507239,5.9335817990719));
#85024=CARTESIAN_POINT('Ctrl Pts',(-17.341,27.2957305755044,5.91606004975545));
#85025=CARTESIAN_POINT('Ctrl Pts',(-17.341,27.2469898227419,5.89785511112464));
#85026=CARTESIAN_POINT('Ctrl Pts',(-17.341,27.1985079825373,5.87896434107663));
#85027=CARTESIAN_POINT('',(-17.341,21.5,-6.08441629692198E-14));
#85028=CARTESIAN_POINT('Origin',(-17.341,26.,-6.02930719096035E-14));
#85029=CARTESIAN_POINT('Ctrl Pts',(-17.341,20.0176003675788,-0.459232662172788));
#85030=CARTESIAN_POINT('Ctrl Pts',(-17.1047385136779,20.1260993589114,-1.87264329110142));
#85031=CARTESIAN_POINT('Ctrl Pts',(-16.8684770273558,20.7549867182113,-3.24026809244986));
#85032=CARTESIAN_POINT('Ctrl Pts',(-16.6322155410337,21.7573593128807,-4.24264068711928));
#85033=CARTESIAN_POINT('Ctrl Pts',(-17.5772614863221,19.1067248030209,-0.529155073934297));
#85034=CARTESIAN_POINT('Ctrl Pts',(-17.341,19.2317437672835,-2.15777051759985));
#85035=CARTESIAN_POINT('Ctrl Pts',(-17.1047385136779,19.9563850319797,-3.7336288188102));
#85036=CARTESIAN_POINT('Ctrl Pts',(-16.8684770273558,21.1113781065848,-4.88862189341524));
#85037=CARTESIAN_POINT('Ctrl Pts',(-17.8135229726442,18.195849238463,-0.599077485695805));
#85038=CARTESIAN_POINT('Ctrl Pts',(-17.5772614863221,18.3373881756556,-2.44289774409829));
#85039=CARTESIAN_POINT('Ctrl Pts',(-17.341,19.1577833457481,-4.22698954517053));
#85040=CARTESIAN_POINT('Ctrl Pts',(-17.1047385136779,20.4653969002888,-5.53460309971121));
#85041=CARTESIAN_POINT('Ctrl Pts',(-18.0497844589663,17.2849736739051,-0.668999897457314));
#85042=CARTESIAN_POINT('Ctrl Pts',(-17.8135229726442,17.4430325840277,-2.72802497059672));
#85043=CARTESIAN_POINT('Ctrl Pts',(-17.5772614863221,18.3591816595165,-4.72035027153087));
#85044=CARTESIAN_POINT('Ctrl Pts',(-17.341,19.8194156939928,-6.18058430600717));
#85045=CARTESIAN_POINT('',(-16.6063537825981,21.8280699909994,-4.17193000900062));
#85046=CARTESIAN_POINT('Ctrl Pts',(-16.6324666134455,21.756063321237,-4.24050691752413));
#85047=CARTESIAN_POINT('Ctrl Pts',(-16.4827322162892,22.3910092147368,-4.87597515128349));
#85048=CARTESIAN_POINT('Ctrl Pts',(-16.1833981689618,23.9499461437912,-5.85575312624584));
#85049=CARTESIAN_POINT('Ctrl Pts',(-15.7344644714635,26.6949162487901,-6.1663874940781));
#85050=CARTESIAN_POINT('Ctrl Pts',(-15.2856655209507,29.3005941525251,-5.25296914865542));
#85051=CARTESIAN_POINT('Ctrl Pts',(-14.8368665704379,31.2541515525533,-3.30156178378519));
#85052=CARTESIAN_POINT('Ctrl Pts',(-14.3880676199251,32.164786766515,-0.694649642063505));
#85053=CARTESIAN_POINT('Ctrl Pts',(-13.9379057895215,31.8558977514204,2.05741712339704));
#85054=CARTESIAN_POINT('Ctrl Pts',(-13.6373436092891,30.8679132696699,3.62177982099857));
#85055=CARTESIAN_POINT('Ctrl Pts',(-13.4863810792274,30.2248412548482,4.25953100287412));
#85056=CARTESIAN_POINT('Ctrl Pts',(-17.0209601030214,20.6934232598663,-5.30228820036689));
#85057=CARTESIAN_POINT('Ctrl Pts',(-16.8712257058651,21.4873533688026,-6.09687143843352));
#85058=CARTESIAN_POINT('Ctrl Pts',(-16.5718916585378,23.4366327933644,-7.32197619516751));
#85059=CARTESIAN_POINT('Ctrl Pts',(-16.1229579610395,26.8689164521759,-7.71039035772407));
#85060=CARTESIAN_POINT('Ctrl Pts',(-15.6741590105267,30.1270305106238,-6.56826102999712));
#85061=CARTESIAN_POINT('Ctrl Pts',(-15.2253600600138,32.5697394962176,-4.12824042724765));
#85062=CARTESIAN_POINT('Ctrl Pts',(-14.776561109501,33.7083888237012,-0.868583089743648));
#85063=CARTESIAN_POINT('Ctrl Pts',(-14.3263992790975,33.3221570330652,2.57257416360736));
#85064=CARTESIAN_POINT('Ctrl Pts',(-14.025837098865,32.086790940846,4.52863791586972));
#85065=CARTESIAN_POINT('Ctrl Pts',(-13.8748745688034,31.2827000096214,5.32607572983823));
#85066=CARTESIAN_POINT('Ctrl Pts',(-17.4094535925974,19.6307831984957,-6.36406948320964));
#85067=CARTESIAN_POINT('Ctrl Pts',(-17.259719195441,20.5836975228685,-7.31776772558355));
#85068=CARTESIAN_POINT('Ctrl Pts',(-16.9603851481138,22.9233194429377,-8.78819926408918));
#85069=CARTESIAN_POINT('Ctrl Pts',(-16.5114514506154,27.0429166555619,-9.25439322137004));
#85070=CARTESIAN_POINT('Ctrl Pts',(-16.0626525001026,30.9534668687226,-7.88355291133882));
#85071=CARTESIAN_POINT('Ctrl Pts',(-15.6138535495898,33.885327439882,-4.95491907071012));
#85072=CARTESIAN_POINT('Ctrl Pts',(-15.1650545990769,35.2519908808874,-1.04251653742379));
#85073=CARTESIAN_POINT('Ctrl Pts',(-14.7148927686735,34.78841631471,3.08773120381769));
#85074=CARTESIAN_POINT('Ctrl Pts',(-14.4143305884409,33.3056686120219,5.43549601074087));
#85075=CARTESIAN_POINT('Ctrl Pts',(-14.2633680583793,32.3405587643947,6.39262045680234));
#85076=CARTESIAN_POINT('Ctrl Pts',(-17.7979470821733,18.568143137125,-7.4258507660524));
#85077=CARTESIAN_POINT('Ctrl Pts',(-17.648212685017,19.6800416769345,-8.53866401273357));
#85078=CARTESIAN_POINT('Ctrl Pts',(-17.3488786376897,22.4100060925109,-10.2544223330108));
#85079=CARTESIAN_POINT('Ctrl Pts',(-16.8999449401914,27.2169168589478,-10.798396085016));
#85080=CARTESIAN_POINT('Ctrl Pts',(-16.4511459896785,31.7799032268214,-9.19884479268053));
#85081=CARTESIAN_POINT('Ctrl Pts',(-16.0023470391657,35.2009153835464,-5.7815977141726));
#85082=CARTESIAN_POINT('Ctrl Pts',(-15.553548088653,36.7955929380736,-1.21644998510393));
#85083=CARTESIAN_POINT('Ctrl Pts',(-15.1033862582494,36.254675596355,3.60288824402801));
#85084=CARTESIAN_POINT('Ctrl Pts',(-14.8028240780169,34.5245462831979,6.34235410561202));
#85085=CARTESIAN_POINT('Ctrl Pts',(-14.6518615479552,33.398417519168,7.45916518376644));
#85086=CARTESIAN_POINT('',(-14.654401924225,33.4246212024587,7.42462120245876));
#85087=CARTESIAN_POINT('Ctrl Pts',(-17.341,22.5935394840313,-9.9320706176077));
#85088=CARTESIAN_POINT('Ctrl Pts',(-17.2130667582964,23.8641814749706,-10.3678701541508));
#85089=CARTESIAN_POINT('Ctrl Pts',(-16.9572002748893,26.5709740036708,-10.7394481103171));
#85090=CARTESIAN_POINT('Ctrl Pts',(-16.445467308075,31.8919112648329,-9.43120169534687));
#85091=CARTESIAN_POINT('Ctrl Pts',(-15.8058010995572,36.8227923782163,-4.14869947052776));
#85092=CARTESIAN_POINT('Ctrl Pts',(-15.1661348910393,36.6915650151942,3.0806737156604));
#85093=CARTESIAN_POINT('Ctrl Pts',(-14.7823351659286,34.3744770613104,6.47476534360713));
#85094=CARTESIAN_POINT('Ctrl Pts',(-14.654401924225,33.4246212024587,7.42462120245876));
#85095=CARTESIAN_POINT('',(-13.4647610361879,30.1719300090006,4.17193000900064));
#85096=CARTESIAN_POINT('Ctrl Pts',(-17.341,22.5935394840313,-9.9320706176077));
#85097=CARTESIAN_POINT('Ctrl Pts',(-17.2130667582964,23.8641814749706,-10.3678701541508));
#85098=CARTESIAN_POINT('Ctrl Pts',(-16.9572002748893,26.5709740036708,-10.7394481103171));
#85099=CARTESIAN_POINT('Ctrl Pts',(-16.445467308075,31.8919112648329,-9.43120169534687));
#85100=CARTESIAN_POINT('Ctrl Pts',(-15.8058010995572,36.8227923782163,-4.14869947052776));
#85101=CARTESIAN_POINT('Ctrl Pts',(-15.1661197260623,36.691561904103,3.08084510704696));
#85102=CARTESIAN_POINT('Ctrl Pts',(-14.7823048359745,34.3742939488486,6.47503356182392));
#85103=CARTESIAN_POINT('Ctrl Pts',(-14.6543564292939,33.4242834123465,7.42495897743765));
#85104=CARTESIAN_POINT('Ctrl Pts',(-18.0433842768097,22.5935394840313,-9.9320706176077));
#85105=CARTESIAN_POINT('Ctrl Pts',(-17.9154510351062,23.8641814749706,-10.3678701541508));
#85106=CARTESIAN_POINT('Ctrl Pts',(-17.659584551699,26.5709740036708,-10.7394481103171));
#85107=CARTESIAN_POINT('Ctrl Pts',(-17.1478515848848,31.8919112648329,-9.43120169534687));
#85108=CARTESIAN_POINT('Ctrl Pts',(-16.5081853763669,36.8227923782163,-4.14869947052775));
#85109=CARTESIAN_POINT('Ctrl Pts',(-15.868504002872,36.691561904103,3.08084510704696));
#85110=CARTESIAN_POINT('Ctrl Pts',(-15.4846891127842,34.3742939488486,6.47503356182392));
#85111=CARTESIAN_POINT('Ctrl Pts',(-15.3567407061037,33.4242834123465,7.42495897743765));
#85112=CARTESIAN_POINT('Ctrl Pts',(-18.7457685536195,22.5935394840313,-9.9320706176077));
#85113=CARTESIAN_POINT('Ctrl Pts',(-18.6178353119159,23.8641814749706,-10.3678701541508));
#85114=CARTESIAN_POINT('Ctrl Pts',(-18.3619688285088,26.5709740036708,-10.7394481103171));
#85115=CARTESIAN_POINT('Ctrl Pts',(-17.8502358616945,31.8919112648329,-9.43120169534687));
#85116=CARTESIAN_POINT('Ctrl Pts',(-17.2105696531766,36.8227923782163,-4.14869947052776));
#85117=CARTESIAN_POINT('Ctrl Pts',(-16.5708882796818,36.691561904103,3.08084510704696));
#85118=CARTESIAN_POINT('Ctrl Pts',(-16.1870733895941,34.3742939488486,6.47503356182392));
#85119=CARTESIAN_POINT('Ctrl Pts',(-16.0591249829134,33.4242834123465,7.42495897743765));
#85120=CARTESIAN_POINT('Ctrl Pts',(-19.4481528304293,22.5935394840313,-9.9320706176077));
#85121=CARTESIAN_POINT('Ctrl Pts',(-19.3202195887258,23.8641814749706,-10.3678701541508));
#85122=CARTESIAN_POINT('Ctrl Pts',(-19.0643531053186,26.5709740036708,-10.7394481103171));
#85123=CARTESIAN_POINT('Ctrl Pts',(-18.5526201385043,31.8919112648329,-9.43120169534687));
#85124=CARTESIAN_POINT('Ctrl Pts',(-17.9129539299865,36.8227923782163,-4.14869947052776));
#85125=CARTESIAN_POINT('Ctrl Pts',(-17.2732725564915,36.691561904103,3.08084510704696));
#85126=CARTESIAN_POINT('Ctrl Pts',(-16.8894576664038,34.3742939488486,6.47503356182392));
#85127=CARTESIAN_POINT('Ctrl Pts',(-16.7615092597232,33.4242834123465,7.42495897743765));
#85128=CARTESIAN_POINT('',(-16.7615242403913,33.4246212024587,7.42462120245876));
#85129=CARTESIAN_POINT('Ctrl Pts',(-17.341094308639,36.2772926947297,2.14768526278091));
#85130=CARTESIAN_POINT('Ctrl Pts',(-17.3074845396453,36.205660317479,2.49222032891058));
#85131=CARTESIAN_POINT('Ctrl Pts',(-17.273944378382,36.1161264432318,2.83269742905984));
#85132=CARTESIAN_POINT('Ctrl Pts',(-17.2404435591107,36.009671232445,3.16762466466842));
#85133=CARTESIAN_POINT('Ctrl Pts',(-17.208700986421,35.9088031838391,3.48497368338849));
#85134=CARTESIAN_POINT('Ctrl Pts',(-17.1769937344665,35.7927434822782,3.79734082231336));
#85135=CARTESIAN_POINT('Ctrl Pts',(-17.1452960571528,35.6622975920403,4.10348960834603));
#85136=CARTESIAN_POINT('Ctrl Pts',(-17.1082962555543,35.5100317963359,4.4608484214461));
#85137=CARTESIAN_POINT('Ctrl Pts',(-17.0712703535404,35.3379954474769,4.81011526676917));
#85138=CARTESIAN_POINT('Ctrl Pts',(-17.0342293500534,35.1473064814038,5.14906385221752));
#85139=CARTESIAN_POINT('Ctrl Pts',(-16.9969240103757,34.9552566992045,5.49043128082452));
#85140=CARTESIAN_POINT('Ctrl Pts',(-16.9596033529182,34.7442875207048,5.82133178564715));
#85141=CARTESIAN_POINT('Ctrl Pts',(-16.9222786137831,34.5155918346289,6.13950603627829));
#85142=CARTESIAN_POINT('Ctrl Pts',(-16.885276572442,34.2888733785379,6.45492945378458));
#85143=CARTESIAN_POINT('Ctrl Pts',(-16.848270519696,34.0447341171065,6.75784492409598));
#85144=CARTESIAN_POINT('Ctrl Pts',(-16.8112714027285,33.78437909671,7.04607825580267));
#85145=CARTESIAN_POINT('Ctrl Pts',(-16.7946872932033,33.6676801988014,7.1752730456687));
#85146=CARTESIAN_POINT('Ctrl Pts',(-16.7781045771455,33.5477239222676,7.30151848264989));
#85147=CARTESIAN_POINT('Ctrl Pts',(-16.7615242403913,33.4246212024587,7.42462120245876));
#85148=CARTESIAN_POINT('',(-16.7615242403913,33.4246212024587,7.42462120245876));
#85149=CARTESIAN_POINT('Origin',(17.341,26.,-5.55111512312578E-14));
#85150=CARTESIAN_POINT('',(17.341,31.8402330044652,5.84023300446519));
#85151=CARTESIAN_POINT('Ctrl Pts',(17.341,31.8402330044652,5.8402330044652));
#85152=CARTESIAN_POINT('Ctrl Pts',(17.341,31.8992685593566,5.67726250202317));
#85153=CARTESIAN_POINT('Ctrl Pts',(17.341,31.9526810918222,5.51251754969076));
#85154=CARTESIAN_POINT('Ctrl Pts',(17.341,32.0002995254776,5.3462623959511));
#85155=CARTESIAN_POINT('Ctrl Pts',(17.341,32.0467530017636,5.18407457814962));
#85156=CARTESIAN_POINT('Ctrl Pts',(17.341,32.0876919849256,5.0204490675178));
#85157=CARTESIAN_POINT('Ctrl Pts',(17.341,32.1229224002175,4.85566538347096));
#85158=CARTESIAN_POINT('Ctrl Pts',(17.341,32.1576023005175,4.69345663042466));
#85159=CARTESIAN_POINT('Ctrl Pts',(17.341,32.1867502430916,4.53012516617391));
#85160=CARTESIAN_POINT('Ctrl Pts',(17.341,32.2101525002504,4.36597803817485));
#85161=CARTESIAN_POINT('Ctrl Pts',(17.341,32.2329501218819,4.20607191926426));
#85162=CARTESIAN_POINT('Ctrl Pts',(17.341,32.2502946593677,4.04539145045367));
#85163=CARTESIAN_POINT('Ctrl Pts',(17.341,32.2619675366177,3.88426442880339));
#85164=CARTESIAN_POINT('Ctrl Pts',(17.341,32.2725061960161,3.73879362801657));
#85165=CARTESIAN_POINT('Ctrl Pts',(17.341,32.2784213451913,3.59295915344904));
#85166=CARTESIAN_POINT('Ctrl Pts',(17.341,32.2795417065118,3.44703729053366));
#85167=CARTESIAN_POINT('Ctrl Pts',(17.341,32.2797575956532,3.41891873170909));
#85168=CARTESIAN_POINT('Ctrl Pts',(17.341,32.2797954074234,3.39079437858622));
#85169=CARTESIAN_POINT('Ctrl Pts',(17.341,32.2796539422494,3.36267510215636));
#85170=CARTESIAN_POINT('Ctrl Pts',(17.341,32.2788934262934,3.21150603495092));
#85171=CARTESIAN_POINT('Ctrl Pts',(17.341,32.2729554998115,3.06063343258084));
#85172=CARTESIAN_POINT('Ctrl Pts',(17.341,32.2616992396755,2.91031447087161));
#85173=CARTESIAN_POINT('Ctrl Pts',(17.341,32.2507045736095,2.7634889029276));
#85174=CARTESIAN_POINT('Ctrl Pts',(17.341,32.2346353579727,2.61719124631499));
#85175=CARTESIAN_POINT('Ctrl Pts',(17.341,32.2133409878654,2.47170640449163));
#85176=CARTESIAN_POINT('Ctrl Pts',(17.341,32.1978029806876,2.36554949517109));
#85177=CARTESIAN_POINT('Ctrl Pts',(17.341,32.1794825144783,2.25982625781697));
#85178=CARTESIAN_POINT('Ctrl Pts',(17.341,32.1583169602484,2.15466449074636));
#85179=CARTESIAN_POINT('Ctrl Pts',(17.341,32.1302989771486,2.01545620068619));
#85180=CARTESIAN_POINT('Ctrl Pts',(17.341,32.0972951601529,1.87722976698276));
#85181=CARTESIAN_POINT('Ctrl Pts',(17.341,32.0592418386405,1.74035383175913));
#85182=CARTESIAN_POINT('Ctrl Pts',(17.341,32.022182235483,1.60705225282758));
#85183=CARTESIAN_POINT('Ctrl Pts',(17.341,31.9803328729637,1.47503151017727));
#85184=CARTESIAN_POINT('Ctrl Pts',(17.341,31.9336396253331,1.34468130064232));
#85185=CARTESIAN_POINT('Ctrl Pts',(17.341,31.9160986730874,1.29571347517094));
#85186=CARTESIAN_POINT('Ctrl Pts',(17.341,31.897874225919,1.24698191069875));
#85187=CARTESIAN_POINT('Ctrl Pts',(17.341,31.8789638354448,1.19850914458424));
#85188=CARTESIAN_POINT('',(17.341,28.1469046708622,10.2782246994423));
#85189=CARTESIAN_POINT('Ctrl Pts',(17.341,28.1469452949575,10.2781625741404));
#85190=CARTESIAN_POINT('Ctrl Pts',(17.341,28.3325279067454,10.1621292850198));
#85191=CARTESIAN_POINT('Ctrl Pts',(17.341,28.5139576804591,10.0400213276751));
#85192=CARTESIAN_POINT('Ctrl Pts',(17.341,28.6909209962493,9.91201604150413));
#85193=CARTESIAN_POINT('Ctrl Pts',(17.341,28.864524013336,9.78644140597534));
#85194=CARTESIAN_POINT('Ctrl Pts',(17.341,29.0338286034143,9.65519060909531));
#85195=CARTESIAN_POINT('Ctrl Pts',(17.341,29.1984889795133,9.51843103193587));
#85196=CARTESIAN_POINT('Ctrl Pts',(17.341,29.3609129200115,9.383528938613));
#85197=CARTESIAN_POINT('Ctrl Pts',(17.341,29.5188179436805,9.24326607244863));
#85198=CARTESIAN_POINT('Ctrl Pts',(17.341,29.6718231704292,9.09781251105125));
#85199=CARTESIAN_POINT('Ctrl Pts',(17.341,29.8213281162527,8.9556864721006));
#85200=CARTESIAN_POINT('Ctrl Pts',(17.341,29.9661547456581,8.80860398474598));
#85201=CARTESIAN_POINT('Ctrl Pts',(17.341,30.1059017960368,8.65674114496278));
#85202=CARTESIAN_POINT('Ctrl Pts',(17.341,30.2254261203405,8.52685430110651));
#85203=CARTESIAN_POINT('Ctrl Pts',(17.341,30.3412338611254,8.39347059630592));
#85204=CARTESIAN_POINT('Ctrl Pts',(17.341,30.4530475545969,8.25671513771186));
#85205=CARTESIAN_POINT('Ctrl Pts',(17.341,30.4741841444228,8.23086370623684));
#85206=CARTESIAN_POINT('Ctrl Pts',(17.341,30.495173125642,8.2048976877583));
#85207=CARTESIAN_POINT('Ctrl Pts',(17.341,30.5160086779073,8.17882334113199));
#85208=CARTESIAN_POINT('Ctrl Pts',(17.341,30.6378636386358,8.02632973579267));
#85209=CARTESIAN_POINT('Ctrl Pts',(17.341,30.754522841015,7.87007095642442));
#85210=CARTESIAN_POINT('Ctrl Pts',(17.341,30.8656903884429,7.71021041498222));
#85211=CARTESIAN_POINT('Ctrl Pts',(17.341,30.9744862217097,7.55376043281476));
#85212=CARTESIAN_POINT('Ctrl Pts',(17.341,31.0780220280316,7.39386017300758));
#85213=CARTESIAN_POINT('Ctrl Pts',(17.341,31.1759745943601,7.23068163057763));
#85214=CARTESIAN_POINT('Ctrl Pts',(17.341,31.2726074170979,7.06970164040195));
#85215=CARTESIAN_POINT('Ctrl Pts',(17.341,31.3638062361732,6.90553057142836));
#85216=CARTESIAN_POINT('Ctrl Pts',(17.341,31.4492184383387,6.73836018750939));
#85217=CARTESIAN_POINT('Ctrl Pts',(17.341,31.5327550010927,6.5748608406618));
#85218=CARTESIAN_POINT('Ctrl Pts',(17.341,31.6107559890823,6.40849201972888));
#85219=CARTESIAN_POINT('Ctrl Pts',(17.341,31.682854645339,6.23946589181676));
#85220=CARTESIAN_POINT('Ctrl Pts',(17.341,31.7389500478517,6.10795735653098));
#85221=CARTESIAN_POINT('Ctrl Pts',(17.341,31.7914717498238,5.97484080451409));
#85222=CARTESIAN_POINT('Ctrl Pts',(17.341,31.8402330044652,5.84023300446519));
#85223=CARTESIAN_POINT('',(17.341,16.0679265366941,-3.4064522188774));
#85224=CARTESIAN_POINT('Ctrl Pts',(17.341,16.0679265366941,-3.4064522188774));
#85225=CARTESIAN_POINT('Ctrl Pts',(17.341,15.9845961443224,-3.16348871151483));
#85226=CARTESIAN_POINT('Ctrl Pts',(17.341,15.9103740268908,-2.91768390374845));
#85227=CARTESIAN_POINT('Ctrl Pts',(17.341,15.8452640134803,-2.66959981594315));
#85228=CARTESIAN_POINT('Ctrl Pts',(17.341,15.7762851031214,-2.40677434321136));
#85229=CARTESIAN_POINT('Ctrl Pts',(17.341,15.717532718057,-2.14139009190298));
#85230=CARTESIAN_POINT('Ctrl Pts',(17.341,15.6690701999576,-1.87409349011832));
#85231=CARTESIAN_POINT('Ctrl Pts',(17.341,15.6229786729691,-1.61987416726227));
#85232=CARTESIAN_POINT('Ctrl Pts',(17.341,15.586195137224,-1.36392425427929));
#85233=CARTESIAN_POINT('Ctrl Pts',(17.341,15.5588262867574,-1.10679133129087));
#85234=CARTESIAN_POINT('Ctrl Pts',(17.341,15.5440859521401,-0.968304501870222));
#85235=CARTESIAN_POINT('Ctrl Pts',(17.341,15.5320774096911,-0.829474436419078));
#85236=CARTESIAN_POINT('Ctrl Pts',(17.341,15.522823606219,-0.690386720854866));
#85237=CARTESIAN_POINT('Ctrl Pts',(17.341,15.5204881459522,-0.655283983447918));
#85238=CARTESIAN_POINT('Ctrl Pts',(17.341,15.5183281478679,-0.620164434365577));
#85239=CARTESIAN_POINT('Ctrl Pts',(17.341,15.5163440946815,-0.58503067513978));
#85240=CARTESIAN_POINT('Ctrl Pts',(17.341,15.5118071418151,-0.504689981294506));
#85241=CARTESIAN_POINT('Ctrl Pts',(17.341,15.5081932973467,-0.424329734635187));
#85242=CARTESIAN_POINT('Ctrl Pts',(17.341,15.5055038583947,-0.343972754343596));
#85243=CARTESIAN_POINT('Ctrl Pts',(17.341,15.4968333929881,-0.0849103884541162));
#85244=CARTESIAN_POINT('Ctrl Pts',(17.341,15.4977656324917,0.174138796742486));
#85245=CARTESIAN_POINT('Ctrl Pts',(17.341,15.5083661305816,0.432621246943835));
#85246=CARTESIAN_POINT('Ctrl Pts',(17.341,15.5101320321375,0.47568097462022));
#85247=CARTESIAN_POINT('Ctrl Pts',(17.341,15.5121663553424,0.518724985663109));
#85248=CARTESIAN_POINT('Ctrl Pts',(17.341,15.5144695437764,0.561750729678525));
#85249=CARTESIAN_POINT('Ctrl Pts',(17.341,15.528277558698,0.819697542286757));
#85250=CARTESIAN_POINT('Ctrl Pts',(17.341,15.5517449206594,1.07698819160038));
#85251=CARTESIAN_POINT('Ctrl Pts',(17.341,15.5847062718016,1.33315042288893));
#85252=CARTESIAN_POINT('Ctrl Pts',(17.341,15.6193150905622,1.60211610326126));
#85253=CARTESIAN_POINT('Ctrl Pts',(17.341,15.6643903836506,1.86983854205682));
#85254=CARTESIAN_POINT('Ctrl Pts',(17.341,15.7198009821417,2.1357590308058));
#85255=CARTESIAN_POINT('Ctrl Pts',(17.341,15.7286446160712,2.1782004322866));
#85256=CARTESIAN_POINT('Ctrl Pts',(17.341,15.7377516426895,2.22059589419355));
#85257=CARTESIAN_POINT('Ctrl Pts',(17.341,15.7471216689552,2.26294309641981));
#85258=CARTESIAN_POINT('Ctrl Pts',(17.341,15.7550108842892,2.29859787343784));
#85259=CARTESIAN_POINT('Ctrl Pts',(17.341,15.7630852570301,2.33421241764003));
#85260=CARTESIAN_POINT('Ctrl Pts',(17.341,15.7713411716081,2.36977215384259));
#85261=CARTESIAN_POINT('Ctrl Pts',(17.341,15.829782966907,2.62149167012282));
#85262=CARTESIAN_POINT('Ctrl Pts',(17.341,15.8973609940489,2.87066335406102));
#85263=CARTESIAN_POINT('Ctrl Pts',(17.341,15.9738605229754,3.11682986990915));
#85264=CARTESIAN_POINT('Ctrl Pts',(17.341,16.050813888197,3.36445677775033));
#85265=CARTESIAN_POINT('Ctrl Pts',(17.341,16.1367950601888,3.60904335199101));
#85266=CARTESIAN_POINT('Ctrl Pts',(17.341,16.2316376645728,3.85011695443059));
#85267=CARTESIAN_POINT('Ctrl Pts',(17.341,16.3107225750279,4.05113720673006));
#85268=CARTESIAN_POINT('Ctrl Pts',(17.341,16.3959699274851,4.24971488739541));
#85269=CARTESIAN_POINT('Ctrl Pts',(17.341,16.4873097035077,4.44556767895105));
#85270=CARTESIAN_POINT('Ctrl Pts',(17.341,16.5966493783922,4.68001625640994));
#85271=CARTESIAN_POINT('Ctrl Pts',(17.341,16.7147183649624,4.91056122178516));
#85272=CARTESIAN_POINT('Ctrl Pts',(17.341,16.8412379141657,5.13669090393161));
#85273=CARTESIAN_POINT('Ctrl Pts',(17.341,16.9668462010638,5.36119187765551));
#85274=CARTESIAN_POINT('Ctrl Pts',(17.341,17.1007841394184,5.58134149474401));
#85275=CARTESIAN_POINT('Ctrl Pts',(17.341,17.2428193477291,5.79660754331022));
#85276=CARTESIAN_POINT('Ctrl Pts',(17.341,17.2761955888083,5.84719198373571));
#85277=CARTESIAN_POINT('Ctrl Pts',(17.341,17.3100191098424,5.89750660346259));
#85278=CARTESIAN_POINT('Ctrl Pts',(17.341,17.3442871876066,5.94754419044709));
#85279=CARTESIAN_POINT('Ctrl Pts',(17.341,17.3706168923142,5.98599031802523));
#85280=CARTESIAN_POINT('Ctrl Pts',(17.341,17.3972133137863,6.02427877787285));
#85281=CARTESIAN_POINT('Ctrl Pts',(17.341,17.4240491903923,6.06236977651445));
#85282=CARTESIAN_POINT('Ctrl Pts',(17.341,17.5735436314461,6.27456305175956));
#85283=CARTESIAN_POINT('Ctrl Pts',(17.341,17.7305971258366,6.48082832820043));
#85284=CARTESIAN_POINT('Ctrl Pts',(17.341,17.8948640063635,6.68069808976308));
#85285=CARTESIAN_POINT('Ctrl Pts',(17.341,18.0589715640803,6.88037399720268));
#85286=CARTESIAN_POINT('Ctrl Pts',(17.341,18.2302788952672,7.07366736772761));
#85287=CARTESIAN_POINT('Ctrl Pts',(17.341,18.4084863697564,7.26008663890563));
#85288=CARTESIAN_POINT('Ctrl Pts',(17.341,18.5489289706688,7.40700083192413));
#85289=CARTESIAN_POINT('Ctrl Pts',(17.341,18.6936580371364,7.54964527618223));
#85290=CARTESIAN_POINT('Ctrl Pts',(17.341,18.8425443966315,7.68776467945016));
#85291=CARTESIAN_POINT('Ctrl Pts',(17.341,19.0319051885732,7.86343154157266));
#85292=CARTESIAN_POINT('Ctrl Pts',(17.341,19.2279900886259,8.03178022504402));
#85293=CARTESIAN_POINT('Ctrl Pts',(17.341,19.43030103464,8.19265160060018));
#85294=CARTESIAN_POINT('Ctrl Pts',(17.341,19.6337043980953,8.35439163254851));
#85295=CARTESIAN_POINT('Ctrl Pts',(17.341,19.8434017995546,8.50857367461105));
#85296=CARTESIAN_POINT('Ctrl Pts',(17.341,20.0589140327271,8.65499096131215));
#85297=CARTESIAN_POINT('Ctrl Pts',(17.341,20.1170226522608,8.69446949244159));
#85298=CARTESIAN_POINT('Ctrl Pts',(17.341,20.1755541364194,8.73338325663078));
#85299=CARTESIAN_POINT('Ctrl Pts',(17.341,20.2344993406077,8.7717276020584));
#85300=CARTESIAN_POINT('Ctrl Pts',(17.341,20.2608991208657,8.78890087861871));
#85301=CARTESIAN_POINT('Ctrl Pts',(17.341,20.2873835813077,8.80596101132696));
#85302=CARTESIAN_POINT('Ctrl Pts',(17.341,20.3139465106913,8.82290412783024));
#85303=CARTESIAN_POINT('Ctrl Pts',(17.341,20.3744302829357,8.86148359265122));
#85304=CARTESIAN_POINT('Ctrl Pts',(17.341,20.4352834531749,8.89943257445888));
#85305=CARTESIAN_POINT('Ctrl Pts',(17.341,20.4964892231803,8.93674624652325));
#85306=CARTESIAN_POINT('Ctrl Pts',(17.341,20.7173534911754,9.0713946116361));
#85307=CARTESIAN_POINT('Ctrl Pts',(17.341,20.9428288522432,9.19778755624999));
#85308=CARTESIAN_POINT('Ctrl Pts',(17.341,21.1723828801861,9.31582124528712));
#85309=CARTESIAN_POINT('Ctrl Pts',(17.341,21.4038163979976,9.43482134351639));
#85310=CARTESIAN_POINT('Ctrl Pts',(17.341,21.6393962155438,9.54532502020363));
#85311=CARTESIAN_POINT('Ctrl Pts',(17.341,21.8786080889347,9.64718249239929));
#85312=CARTESIAN_POINT('Ctrl Pts',(17.341,22.118070891722,9.74914681144021));
#85313=CARTESIAN_POINT('Ctrl Pts',(17.341,22.361173983963,9.84244701763524));
#85314=CARTESIAN_POINT('Ctrl Pts',(17.341,22.6074238642972,9.92688573515372));
#85315=CARTESIAN_POINT('Ctrl Pts',(17.341,22.8521249582807,10.0107933761374));
#85316=CARTESIAN_POINT('Ctrl Pts',(17.341,23.0999339927884,10.0859508329837));
#85317=CARTESIAN_POINT('Ctrl Pts',(17.341,23.3503796394041,10.1521148249929));
#85318=CARTESIAN_POINT('Ctrl Pts',(17.341,23.5813869667577,10.2131435039404));
#85319=CARTESIAN_POINT('Ctrl Pts',(17.341,23.8146380016544,10.2665202226159));
#85320=CARTESIAN_POINT('Ctrl Pts',(17.341,24.0497660152581,10.3120140744538));
#85321=CARTESIAN_POINT('Ctrl Pts',(17.341,24.080163066604,10.3178954619118));
#85322=CARTESIAN_POINT('Ctrl Pts',(17.341,24.1105928674216,10.323645259904));
#85323=CARTESIAN_POINT('Ctrl Pts',(17.341,24.141036215458,10.3292596547578));
#85324=CARTESIAN_POINT('Ctrl Pts',(17.341,24.3979233185446,10.3766350494692));
#85325=CARTESIAN_POINT('Ctrl Pts',(17.341,24.6560576019166,10.4144296911714));
#85326=CARTESIAN_POINT('Ctrl Pts',(17.341,24.9149377889596,10.4424928180281));
#85327=CARTESIAN_POINT('Ctrl Pts',(17.341,25.171976331243,10.4703563069322));
#85328=CARTESIAN_POINT('Ctrl Pts',(17.341,25.4297503170471,10.4886263071145));
#85329=CARTESIAN_POINT('Ctrl Pts',(17.341,25.6877814236054,10.4971057263321));
#85330=CARTESIAN_POINT('Ctrl Pts',(17.341,25.8537611339476,10.5025601522128));
#85331=CARTESIAN_POINT('Ctrl Pts',(17.341,26.0198474887083,10.5039624655609));
#85332=CARTESIAN_POINT('Ctrl Pts',(17.341,26.1859144523977,10.5012488452782));
#85333=CARTESIAN_POINT('Ctrl Pts',(17.341,26.4435060609303,10.4970396648485));
#85334=CARTESIAN_POINT('Ctrl Pts',(17.341,26.7010514637349,10.4829300428959));
#85335=CARTESIAN_POINT('Ctrl Pts',(17.341,26.9580017760534,10.4591240892664));
#85336=CARTESIAN_POINT('Ctrl Pts',(17.341,27.2156042235232,10.4352577165658));
#85337=CARTESIAN_POINT('Ctrl Pts',(17.341,27.4726092240827,10.4016455486853));
#85338=CARTESIAN_POINT('Ctrl Pts',(17.341,27.7284529044781,10.3584422735481));
#85339=CARTESIAN_POINT('Ctrl Pts',(17.341,27.8681170757507,10.3348577565924));
#85340=CARTESIAN_POINT('Ctrl Pts',(17.341,28.0074349233039,10.3084141893606));
#85341=CARTESIAN_POINT('Ctrl Pts',(17.341,28.146312267496,10.2791306454767));
#85342=CARTESIAN_POINT('',(17.3409999839613,19.8194178862033,-6.18058216019384));
#85343=CARTESIAN_POINT('Origin',(17.3409999999995,21.3441513567948,1.29316405882314));
#85344=CARTESIAN_POINT('Ctrl Pts',(17.341,25.540762340228,-5.98239924878362));
#85345=CARTESIAN_POINT('Ctrl Pts',(17.341,25.4183996188332,-6.04858855516172));
#85346=CARTESIAN_POINT('Ctrl Pts',(17.341,25.293627346394,-6.10999579303368));
#85347=CARTESIAN_POINT('Ctrl Pts',(17.341,25.1668334048713,-6.16670216610432));
#85348=CARTESIAN_POINT('Ctrl Pts',(17.341,25.0371649034307,-6.22469413583013));
#85349=CARTESIAN_POINT('Ctrl Pts',(17.341,24.9053820043425,-6.27777033516398));
#85350=CARTESIAN_POINT('Ctrl Pts',(17.341,24.771845187989,-6.32602964024892));
#85351=CARTESIAN_POINT('Ctrl Pts',(17.341,24.6729857355588,-6.36175677981713));
#85352=CARTESIAN_POINT('Ctrl Pts',(17.341,24.5731638536018,-6.39484421795225));
#85353=CARTESIAN_POINT('Ctrl Pts',(17.341,24.4725076277925,-6.42533310314458));
#85354=CARTESIAN_POINT('Ctrl Pts',(17.341,24.4137637069362,-6.44312670353376));
#85355=CARTESIAN_POINT('Ctrl Pts',(17.341,24.3547359339088,-6.46003507521374));
#85356=CARTESIAN_POINT('Ctrl Pts',(17.341,24.2954455073458,-6.47606676524652));
#85357=CARTESIAN_POINT('Ctrl Pts',(17.341,24.2467280160254,-6.48923961228606));
#85358=CARTESIAN_POINT('Ctrl Pts',(17.341,24.1978356308289,-6.50181966029287));
#85359=CARTESIAN_POINT('Ctrl Pts',(17.341,24.1488067498374,-6.51380557918685));
#85360=CARTESIAN_POINT('Ctrl Pts',(17.341,24.0007014245001,-6.55001236957977));
#85361=CARTESIAN_POINT('Ctrl Pts',(17.341,23.8513020969686,-6.5808123761519));
#85362=CARTESIAN_POINT('Ctrl Pts',(17.341,23.7009841745541,-6.60634967722337));
#85363=CARTESIAN_POINT('Ctrl Pts',(17.341,23.5476129800787,-6.63240569440416));
#85364=CARTESIAN_POINT('Ctrl Pts',(17.341,23.3932853069637,-6.65298361480213));
#85365=CARTESIAN_POINT('Ctrl Pts',(17.341,23.2383461904164,-6.66823130644756));
#85366=CARTESIAN_POINT('Ctrl Pts',(17.341,23.1373547140553,-6.67816996444875));
#85367=CARTESIAN_POINT('Ctrl Pts',(17.341,23.0361023630569,-6.68584387994372));
#85368=CARTESIAN_POINT('Ctrl Pts',(17.341,22.934673477861,-6.69129118893674));
#85369=CARTESIAN_POINT('Ctrl Pts',(17.341,22.8806851312291,-6.69419067073187));
#85370=CARTESIAN_POINT('Ctrl Pts',(17.341,22.8266453434879,-6.69645930799709));
#85371=CARTESIAN_POINT('Ctrl Pts',(17.341,22.7725693409315,-6.69810238552906));
#85372=CARTESIAN_POINT('Ctrl Pts',(17.341,22.7271872751647,-6.69948130129744));
#85373=CARTESIAN_POINT('Ctrl Pts',(17.341,22.6817878595131,-6.70041931464329));
#85374=CARTESIAN_POINT('Ctrl Pts',(17.341,22.6363912203757,-6.70092013375722));
#85375=CARTESIAN_POINT('Ctrl Pts',(17.341,22.4688853069381,-6.70276807150637));
#85376=CARTESIAN_POINT('Ctrl Pts',(17.341,22.3013726898151,-6.69866601218014));
#85377=CARTESIAN_POINT('Ctrl Pts',(17.341,22.1342411971029,-6.68881383255924));
#85378=CARTESIAN_POINT('Ctrl Pts',(17.341,21.9639554414572,-6.67877571332584));
#85379=CARTESIAN_POINT('Ctrl Pts',(17.341,21.7940650425909,-6.66276887957955));
#85380=CARTESIAN_POINT('Ctrl Pts',(17.341,21.6249279438386,-6.64099010569175));
#85381=CARTESIAN_POINT('Ctrl Pts',(17.341,21.4510285893043,-6.61859812457362));
#85382=CARTESIAN_POINT('Ctrl Pts',(17.341,21.2779252433068,-6.59010512149647));
#85383=CARTESIAN_POINT('Ctrl Pts',(17.341,21.1059567043584,-6.55570169646653));
#85384=CARTESIAN_POINT('Ctrl Pts',(17.341,20.9315335584359,-6.52080721134196));
#85385=CARTESIAN_POINT('Ctrl Pts',(17.341,20.7582773397082,-6.47983282131137));
#85386=CARTESIAN_POINT('Ctrl Pts',(17.341,20.5864970100379,-6.43294640530162));
#85387=CARTESIAN_POINT('Ctrl Pts',(17.341,20.4116858195953,-6.38523273392849));
#85388=CARTESIAN_POINT('Ctrl Pts',(17.341,20.2384024855397,-6.33139701701376));
#85389=CARTESIAN_POINT('Ctrl Pts',(17.341,20.0669350139262,-6.27157747171442));
#85390=CARTESIAN_POINT('Ctrl Pts',(17.341,19.9839949222142,-6.24264231260461));
#85391=CARTESIAN_POINT('Ctrl Pts',(17.341,19.9014791913052,-6.21230648506642));
#85392=CARTESIAN_POINT('Ctrl Pts',(17.341,19.8194179780815,-6.18058202191849));
#85393=CARTESIAN_POINT('',(17.341,21.5,-6.08441629692198E-14));
#85394=CARTESIAN_POINT('Origin',(17.341,26.,-6.02930719096035E-14));
#85395=CARTESIAN_POINT('Ctrl Pts',(16.7615124374135,33.4249061655004,7.42433622827797));
#85396=CARTESIAN_POINT('Ctrl Pts',(16.8894584331897,32.474992220184,8.37432443882492));
#85397=CARTESIAN_POINT('Ctrl Pts',(17.1453376308892,30.2091713978346,9.89763205493));
#85398=CARTESIAN_POINT('Ctrl Pts',(17.6570832324356,24.8471265934024,11.0609731255039));
#85399=CARTESIAN_POINT('Ctrl Pts',(18.1688160401292,19.4649378970143,8.99752970904879));
#85400=CARTESIAN_POINT('Ctrl Pts',(18.6805488478228,16.2522102217688,4.55237376613912));
#85401=CARTESIAN_POINT('Ctrl Pts',(19.064348453593,15.2532613557681,0.57767028582841));
#85402=CARTESIAN_POINT('Ctrl Pts',(19.3202148574397,15.6321281971341,-2.13581025897831));
#85403=CARTESIAN_POINT('Ctrl Pts',(19.4481480593631,16.0679265366941,-3.4064522188774));
#85404=CARTESIAN_POINT('Ctrl Pts',(16.0591297509591,33.4249061655004,7.42433622827797));
#85405=CARTESIAN_POINT('Ctrl Pts',(16.1870757467353,32.474992220184,8.37432443882492));
#85406=CARTESIAN_POINT('Ctrl Pts',(16.4429549444349,30.2091713978346,9.89763205493));
#85407=CARTESIAN_POINT('Ctrl Pts',(16.9547005459813,24.8471265934024,11.0609731255039));
#85408=CARTESIAN_POINT('Ctrl Pts',(17.4664333536749,19.4649378970143,8.99752970904879));
#85409=CARTESIAN_POINT('Ctrl Pts',(17.9781661613684,16.2522102217688,4.55237376613912));
#85410=CARTESIAN_POINT('Ctrl Pts',(18.3619657671386,15.2532613557681,0.577670285828411));
#85411=CARTESIAN_POINT('Ctrl Pts',(18.6178321709854,15.6321281971341,-2.13581025897831));
#85412=CARTESIAN_POINT('Ctrl Pts',(18.7457653729088,16.0679265366941,-3.4064522188774));
#85413=CARTESIAN_POINT('Ctrl Pts',(15.3567470645047,33.4249061655004,7.42433622827797));
#85414=CARTESIAN_POINT('Ctrl Pts',(15.4846930602809,32.474992220184,8.37432443882493));
#85415=CARTESIAN_POINT('Ctrl Pts',(15.7405722579805,30.2091713978346,9.89763205493));
#85416=CARTESIAN_POINT('Ctrl Pts',(16.2523178595268,24.8471265934024,11.060973125504));
#85417=CARTESIAN_POINT('Ctrl Pts',(16.7640506672204,19.4649378970143,8.99752970904879));
#85418=CARTESIAN_POINT('Ctrl Pts',(17.275783474914,16.2522102217688,4.55237376613912));
#85419=CARTESIAN_POINT('Ctrl Pts',(17.6595830806842,15.2532613557681,0.577670285828411));
#85420=CARTESIAN_POINT('Ctrl Pts',(17.915449484531,15.6321281971341,-2.13581025897831));
#85421=CARTESIAN_POINT('Ctrl Pts',(18.0433826864543,16.0679265366941,-3.4064522188774));
#85422=CARTESIAN_POINT('Ctrl Pts',(14.6543643780503,33.4249061655004,7.42433622827796));
#85423=CARTESIAN_POINT('Ctrl Pts',(14.7823103738265,32.474992220184,8.37432443882492));
#85424=CARTESIAN_POINT('Ctrl Pts',(15.0381895715261,30.2091713978346,9.89763205493));
#85425=CARTESIAN_POINT('Ctrl Pts',(15.5499351730725,24.8471265934024,11.0609731255039));
#85426=CARTESIAN_POINT('Ctrl Pts',(16.0616679807661,19.4649378970143,8.99752970904879));
#85427=CARTESIAN_POINT('Ctrl Pts',(16.5734007884596,16.2522102217688,4.55237376613912));
#85428=CARTESIAN_POINT('Ctrl Pts',(16.9572003942298,15.2532613557681,0.57767028582841));
#85429=CARTESIAN_POINT('Ctrl Pts',(17.2130667980766,15.6321281971341,-2.13581025897831));
#85430=CARTESIAN_POINT('Ctrl Pts',(17.341,16.0679265366941,-3.4064522188774));
#85431=CARTESIAN_POINT('',(16.761525075775,33.4246212024587,7.42462120245876));
#85432=CARTESIAN_POINT('Ctrl Pts',(16.761525075775,33.4246212024587,7.42462120245875));
#85433=CARTESIAN_POINT('Ctrl Pts',(16.796415203332,33.1655752216426,7.68366718327491));
#85434=CARTESIAN_POINT('Ctrl Pts',(16.8312868468052,32.8928326264494,7.92856820410911));
#85435=CARTESIAN_POINT('Ctrl Pts',(16.8661515162646,32.6080803815643,8.15849134617175));
#85436=CARTESIAN_POINT('Ctrl Pts',(16.9013571533157,32.3205433322152,8.39066307803096));
#85437=CARTESIAN_POINT('Ctrl Pts',(16.9365556792779,32.0207598439169,8.60756302871267));
#85438=CARTESIAN_POINT('Ctrl Pts',(16.9717589452313,31.710429563843,8.80829510701351));
#85439=CARTESIAN_POINT('Ctrl Pts',(17.0068253488282,31.4013057778907,9.0082467842771));
#85440=CARTESIAN_POINT('Ctrl Pts',(17.0418964556319,31.0817162363085,9.19215646243076));
#85441=CARTESIAN_POINT('Ctrl Pts',(17.0769839790363,30.7533157721565,9.3590938754793));
#85442=CARTESIAN_POINT('Ctrl Pts',(17.0996969030388,30.5407349439604,9.46715612689669));
#85443=CARTESIAN_POINT('Ctrl Pts',(17.1224167060189,30.3244616354424,9.56810564435477));
#85444=CARTESIAN_POINT('Ctrl Pts',(17.1451465651708,30.1049414928425,9.66167885853807));
#85445=CARTESIAN_POINT('Ctrl Pts',(17.1720213888841,29.8453901645892,9.77231586770984));
#85446=CARTESIAN_POINT('Ctrl Pts',(17.1989367351104,29.5812233705055,9.87257656592876));
#85447=CARTESIAN_POINT('Ctrl Pts',(17.2258528491582,29.3134003424746,9.9620468904518));
#85448=CARTESIAN_POINT('Ctrl Pts',(17.252643297162,29.0468277274996,10.0510994956222));
#85449=CARTESIAN_POINT('Ctrl Pts',(17.2794345058345,28.7766335588408,10.1294624424491));
#85450=CARTESIAN_POINT('Ctrl Pts',(17.3061872747089,28.5037474425124,10.1967762920531));
#85451=CARTESIAN_POINT('Ctrl Pts',(17.3177998278266,28.3852959829343,10.2259951612382));
#85452=CARTESIAN_POINT('Ctrl Pts',(17.3294051382684,28.2663370545596,10.2531328098949));
#85453=CARTESIAN_POINT('Ctrl Pts',(17.341,28.1469452949575,10.2781625741404));
#85454=CARTESIAN_POINT('',(14.6544027596087,33.4246212024587,7.42462120245876));
#85455=CARTESIAN_POINT('',(14.6544027596087,33.4246212024587,7.42462120245876));
#85456=CARTESIAN_POINT('Ctrl Pts',(14.6544027596087,33.4246212024587,7.42462120245875));
#85457=CARTESIAN_POINT('Ctrl Pts',(14.7823359615321,32.4747656389599,8.37447676595761));
#85458=CARTESIAN_POINT('Ctrl Pts',(15.0382023653789,30.2090373444851,9.89766113894045));
#85459=CARTESIAN_POINT('Ctrl Pts',(15.5499351730725,24.8471265934024,11.0609731255039));
#85460=CARTESIAN_POINT('Ctrl Pts',(16.0616679807661,19.4649378970143,8.99752970904879));
#85461=CARTESIAN_POINT('Ctrl Pts',(16.5734007884596,16.2522102217688,4.55237376613912));
#85462=CARTESIAN_POINT('Ctrl Pts',(16.9572003942298,15.2532613557681,0.57767028582841));
#85463=CARTESIAN_POINT('Ctrl Pts',(17.2130667980766,15.6321281971341,-2.13581025897831));
#85464=CARTESIAN_POINT('Ctrl Pts',(17.341,16.0679265366941,-3.4064522188774));
#85465=CARTESIAN_POINT('Ctrl Pts',(17.341,31.8402330044652,5.84023300446519));
#85466=CARTESIAN_POINT('Ctrl Pts',(17.534158308075,30.7121434785588,6.96832253037151));
#85467=CARTESIAN_POINT('Ctrl Pts',(17.72731661615,29.250448427975,7.75863390468211));
#85468=CARTESIAN_POINT('Ctrl Pts',(17.920474924225,27.6887946776651,8.08483862730598));
#85469=CARTESIAN_POINT('Ctrl Pts',(17.147841691925,32.3683624037964,6.36836240379638));
#85470=CARTESIAN_POINT('Ctrl Pts',(17.341,31.1382602966705,7.59846451092218));
#85471=CARTESIAN_POINT('Ctrl Pts',(17.534158308075,29.5443848812828,8.460243354267));
#85472=CARTESIAN_POINT('Ctrl Pts',(17.72731661615,27.8415115500959,8.81594660958411));
#85473=CARTESIAN_POINT('Ctrl Pts',(16.95468338385,32.8964918031275,6.89649180312756));
#85474=CARTESIAN_POINT('Ctrl Pts',(17.147841691925,31.5643771147823,8.22860649147286));
#85475=CARTESIAN_POINT('Ctrl Pts',(17.341,29.8383213345905,9.1618528038519));
#85476=CARTESIAN_POINT('Ctrl Pts',(17.534158308075,27.9942284225267,9.54705459186225));
#85477=CARTESIAN_POINT('Ctrl Pts',(16.761525075775,33.4246212024587,7.42462120245875));
#85478=CARTESIAN_POINT('Ctrl Pts',(16.95468338385,31.990493932894,8.85874847202353));
#85479=CARTESIAN_POINT('Ctrl Pts',(17.147841691925,30.1322577878983,9.86346225343679));
#85480=CARTESIAN_POINT('Ctrl Pts',(17.341,28.1469452949574,10.2781625741404));
#85481=CARTESIAN_POINT('',(17.9511659638121,30.1719300090006,4.17193000900064));
#85482=CARTESIAN_POINT('Ctrl Pts',(14.7834604024327,21.7560634031344,-4.24050705242816));
#85483=CARTESIAN_POINT('Ctrl Pts',(14.9331947910706,22.3910092806787,-4.87597523762566));
#85484=CARTESIAN_POINT('Ctrl Pts',(15.2325288298794,23.9499464904882,-5.8557529849313));
#85485=CARTESIAN_POINT('Ctrl Pts',(15.6814625188592,26.6949161928493,-6.16638799654186));
#85486=CARTESIAN_POINT('Ctrl Pts',(16.1302614693721,29.3005937404032,-5.25296922685046));
#85487=CARTESIAN_POINT('Ctrl Pts',(16.5790604198849,31.2541512947311,-3.30156243078436));
#85488=CARTESIAN_POINT('Ctrl Pts',(17.0278593703977,32.1647858337878,-0.694650259068251));
#85489=CARTESIAN_POINT('Ctrl Pts',(17.4766583209106,31.8568326061558,2.04908452357241));
#85490=CARTESIAN_POINT('Ctrl Pts',(17.7758576212524,30.876857130788,3.60758722349281));
#85491=CARTESIAN_POINT('Ctrl Pts',(17.9254572714234,30.2422221771405,4.24222217714045));
#85492=CARTESIAN_POINT('Ctrl Pts',(14.3954830038832,20.6948350244358,-5.30087784765443));
#85493=CARTESIAN_POINT('Ctrl Pts',(14.5452173925211,21.4885539111445,-6.09524964898742));
#85494=CARTESIAN_POINT('Ctrl Pts',(14.84455143133,23.4373151369117,-7.32002821723511));
#85495=CARTESIAN_POINT('Ctrl Pts',(15.2934851203098,26.8686852320035,-7.70833985812943));
#85496=CARTESIAN_POINT('Ctrl Pts',(15.7422840708226,30.1259321176207,-6.56651383071689));
#85497=CARTESIAN_POINT('Ctrl Pts',(16.1910830213355,32.5679914835932,-4.12714303634316));
#85498=CARTESIAN_POINT('Ctrl Pts',(16.6398819718483,33.7063370624859,-0.868352799473312));
#85499=CARTESIAN_POINT('Ctrl Pts',(17.0886809223611,33.3213778058956,2.5614735749011));
#85500=CARTESIAN_POINT('Ctrl Pts',(17.387880222703,32.0963520661915,4.5096916383016));
#85501=CARTESIAN_POINT('Ctrl Pts',(17.5374798728739,31.3030218522465,5.30302185224656));
#85502=CARTESIAN_POINT('Ctrl Pts',(14.0075056053337,19.6336066457373,-6.3612486428807));
#85503=CARTESIAN_POINT('Ctrl Pts',(14.1572399939717,20.5860985416104,-7.31452406034918));
#85504=CARTESIAN_POINT('Ctrl Pts',(14.4565740327805,22.9246837833351,-8.78430344953894));
#85505=CARTESIAN_POINT('Ctrl Pts',(14.9055077217603,27.0424542711577,-9.250291719717));
#85506=CARTESIAN_POINT('Ctrl Pts',(15.3543066722731,30.9512704948381,-7.88005843458333));
#85507=CARTESIAN_POINT('Ctrl Pts',(15.8031056227859,33.8818316724552,-4.95272364190195));
#85508=CARTESIAN_POINT('Ctrl Pts',(16.2519045732988,35.2478882911839,-1.04205533987837));
#85509=CARTESIAN_POINT('Ctrl Pts',(16.7007035238116,34.7859230056355,3.0738626262298));
#85510=CARTESIAN_POINT('Ctrl Pts',(16.9999028241535,33.3158470015949,5.41179605311038));
#85511=CARTESIAN_POINT('Ctrl Pts',(17.1495024743244,32.3638215273526,6.36382152735266));
#85512=CARTESIAN_POINT('Ctrl Pts',(13.6195282067842,18.5723782670386,-7.42161943810697));
#85513=CARTESIAN_POINT('Ctrl Pts',(13.7692625954221,19.6836431720763,-8.53379847171094));
#85514=CARTESIAN_POINT('Ctrl Pts',(14.068596634231,22.4120524297584,-10.2485786818427));
#85515=CARTESIAN_POINT('Ctrl Pts',(14.5175303232108,27.2162233103119,-10.7922435813046));
#85516=CARTESIAN_POINT('Ctrl Pts',(14.9663292737237,31.7766088720556,-9.19360303844975));
#85517=CARTESIAN_POINT('Ctrl Pts',(15.4151282242365,35.1956718613173,-5.77830424746075));
#85518=CARTESIAN_POINT('Ctrl Pts',(15.8639271747493,36.7894395198819,-1.21575788028343));
#85519=CARTESIAN_POINT('Ctrl Pts',(16.3127261252621,36.2504682053753,3.58625167755849));
#85520=CARTESIAN_POINT('Ctrl Pts',(16.611925425604,34.5353419369983,6.31390046791915));
#85521=CARTESIAN_POINT('Ctrl Pts',(16.761525075775,33.4246212024587,7.42462120245876));
#85522=CARTESIAN_POINT('',(13.6199323608887,18.5753787991571,-7.42462120084289));
#85523=CARTESIAN_POINT('',(14.8095732174019,21.8280699909994,-4.17193000900062));
#85524=CARTESIAN_POINT('Ctrl Pts',(13.6199324221852,18.5753787975412,-7.42462120245874));
#85525=CARTESIAN_POINT('Ctrl Pts',(13.7695320723561,19.6860995320808,-8.53534193699833));
#85526=CARTESIAN_POINT('Ctrl Pts',(14.068731372698,22.4134943055532,-10.2487418519877));
#85527=CARTESIAN_POINT('Ctrl Pts',(14.5175303232108,27.2162233103119,-10.7922435813046));
#85528=CARTESIAN_POINT('Ctrl Pts',(14.9663292737237,31.7766088720556,-9.19360303844976));
#85529=CARTESIAN_POINT('Ctrl Pts',(15.4151282242365,35.1956718613173,-5.77830424746075));
#85530=CARTESIAN_POINT('Ctrl Pts',(15.8639271747493,36.7894395198819,-1.21575788028344));
#85531=CARTESIAN_POINT('Ctrl Pts',(16.3127261252621,36.2504682053753,3.58625167755849));
#85532=CARTESIAN_POINT('Ctrl Pts',(16.611925425604,34.5353419369983,6.31390046791915));
#85533=CARTESIAN_POINT('Ctrl Pts',(16.761525075775,33.4246212024587,7.42462120245876));
#85534=CARTESIAN_POINT('Origin',(-36.3408714641021,26.,7.7715611723761E-15));
#85535=CARTESIAN_POINT('',(-36.6591285358979,21.5,8.3226522319924E-15));
#85536=CARTESIAN_POINT('Origin',(-36.6591285358979,26.,7.7715611723761E-15));
#85537=CARTESIAN_POINT('',(-36.3408714641021,21.5,8.32265223199241E-15));
#85538=CARTESIAN_POINT('Origin',(36.3408714641021,26.,7.7715611723761E-15));
#85539=CARTESIAN_POINT('',(36.3408714641021,21.5,7.22047011275979E-15));
#85540=CARTESIAN_POINT('',(36.3408714641021,21.5,8.32265223199241E-15));
#85541=CARTESIAN_POINT('Origin',(36.3408714641021,26.,7.7715611723761E-15));
#85542=CARTESIAN_POINT('Origin',(36.3408714641021,26.,7.7715611723761E-15));
#85543=CARTESIAN_POINT('Ctrl Pts',(17.3410000905454,19.8194177305141,-6.18058226948589));
#85544=CARTESIAN_POINT('Ctrl Pts',(17.5772612984063,21.2796495627862,-7.64081410175804));
#85545=CARTESIAN_POINT('Ctrl Pts',(17.8135225062671,23.2719712067439,-8.55696250376816));
#85546=CARTESIAN_POINT('Ctrl Pts',(18.049783714128,25.3309930425917,-8.71502289559277));
#85547=CARTESIAN_POINT('Ctrl Pts',(17.1047388505631,20.465398263273,-5.53460173672703));
#85548=CARTESIAN_POINT('Ctrl Pts',(17.341000058424,21.7730099546209,-6.84221342807497));
#85549=CARTESIAN_POINT('Ctrl Pts',(17.5772612662848,23.5570986294383,-7.66260806336661));
#85550=CARTESIAN_POINT('Ctrl Pts',(17.8135224741457,25.4009161423779,-7.80414833917836));
#85551=CARTESIAN_POINT('Ctrl Pts',(16.8684776105808,21.1113787960318,-4.88862120396816));
#85552=CARTESIAN_POINT('Ctrl Pts',(17.1047388184417,22.2663703464555,-6.04361275439188));
#85553=CARTESIAN_POINT('Ctrl Pts',(17.3410000263025,23.8422260521326,-6.76825362296505));
#85554=CARTESIAN_POINT('Ctrl Pts',(17.5772612341634,25.470839242164,-6.89327378276394));
#85555=CARTESIAN_POINT('Ctrl Pts',(16.6322163705985,21.7573593287907,-4.24264067120929));
#85556=CARTESIAN_POINT('Ctrl Pts',(16.8684775784594,22.7597307382902,-5.24501208070881));
#85557=CARTESIAN_POINT('Ctrl Pts',(17.1047387863202,24.127353474827,-5.8738991825635));
#85558=CARTESIAN_POINT('Ctrl Pts',(17.3409999941811,25.5407623419502,-5.98239922634953));
#85559=CARTESIAN_POINT('',(17.7959954131985,18.5753787975412,-7.42462120245874));
#85560=CARTESIAN_POINT('Ctrl Pts',(11.5124058800916,18.5723781889139,-7.42161935992234));
#85561=CARTESIAN_POINT('Ctrl Pts',(11.6621402722384,19.6836431101435,-8.53379843028192));
#85562=CARTESIAN_POINT('Ctrl Pts',(11.961474314556,22.4120501365063,-10.2485800412561));
#85563=CARTESIAN_POINT('Ctrl Pts',(12.4104080070446,27.2162237256492,-10.7922402146103));
#85564=CARTESIAN_POINT('Ctrl Pts',(12.8592069575574,31.7766119901629,-9.19360275595219));
#85565=CARTESIAN_POINT('Ctrl Pts',(13.3080059080703,35.1956739272439,-5.77829971989694));
#85566=CARTESIAN_POINT('Ctrl Pts',(13.7568048585831,36.7894465571738,-1.21575346390194));
#85567=CARTESIAN_POINT('Ctrl Pts',(14.2057182183514,36.2503333440016,3.58748045005371));
#85568=CARTESIAN_POINT('Ctrl Pts',(14.5050319279488,34.5340300604887,6.31598641782465));
#85569=CARTESIAN_POINT('Ctrl Pts',(14.6547459873753,33.4220724221517,7.42716909445542));
#85570=CARTESIAN_POINT('Ctrl Pts',(11.1244284782739,19.6336065877144,-6.3612485669342));
#85571=CARTESIAN_POINT('Ctrl Pts',(11.2741628704205,20.5860984961286,-7.31452401456818));
#85572=CARTESIAN_POINT('Ctrl Pts',(11.5734969127382,22.9246818220518,-8.78430460238974));
#85573=CARTESIAN_POINT('Ctrl Pts',(12.0224306052268,27.0424546256895,-9.25028882105291));
#85574=CARTESIAN_POINT('Ctrl Pts',(12.4712295557397,30.9512731604903,-7.88005818138255));
#85575=CARTESIAN_POINT('Ctrl Pts',(12.9200285062525,33.8818334321429,-4.95271975426335));
#85576=CARTESIAN_POINT('Ctrl Pts',(13.3688274567653,35.2478943100302,-1.04205155302823));
#85577=CARTESIAN_POINT('Ctrl Pts',(13.8177408165336,34.785807400369,3.07491583239152));
#85578=CARTESIAN_POINT('Ctrl Pts',(14.117054526131,33.314722550393,5.41358396337687));
#85579=CARTESIAN_POINT('Ctrl Pts',(14.2667685855575,32.3616368974747,6.36600537796603));
#85580=CARTESIAN_POINT('Ctrl Pts',(10.736451076456,20.6948349865149,-5.30087777394604));
#85581=CARTESIAN_POINT('Ctrl Pts',(10.8861854686027,21.4885538821137,-6.09524959885446));
#85582=CARTESIAN_POINT('Ctrl Pts',(11.1855195109204,23.4373135075974,-7.3200291635234));
#85583=CARTESIAN_POINT('Ctrl Pts',(11.6344532034089,26.8686855257297,-7.7083374274955));
#85584=CARTESIAN_POINT('Ctrl Pts',(12.0832521539218,30.1259343308177,-6.5665136068129));
#85585=CARTESIAN_POINT('Ctrl Pts',(12.5320511044346,32.5679929370418,-4.12713978862975));
#85586=CARTESIAN_POINT('Ctrl Pts',(12.9808500549474,33.7063420628864,-0.86834964215453));
#85587=CARTESIAN_POINT('Ctrl Pts',(13.4297634147159,33.3212814567364,2.56235121472933));
#85588=CARTESIAN_POINT('Ctrl Pts',(13.7290771243132,32.0954150402973,4.51118150892909));
#85589=CARTESIAN_POINT('Ctrl Pts',(13.8787911837397,31.3012013727976,5.30484166147665));
#85590=CARTESIAN_POINT('Ctrl Pts',(10.3484736746382,21.7560633853155,-4.2405069809579));
#85591=CARTESIAN_POINT('Ctrl Pts',(10.498208066785,22.3910092680988,-4.87597518314072));
#85592=CARTESIAN_POINT('Ctrl Pts',(10.7975421091025,23.9499451931429,-5.85575372465707));
#85593=CARTESIAN_POINT('Ctrl Pts',(11.2464758015912,26.69491642577,-6.16638603393809));
#85594=CARTESIAN_POINT('Ctrl Pts',(11.695274752104,29.3005955011451,-5.25296903224326));
#85595=CARTESIAN_POINT('Ctrl Pts',(12.1440737026168,31.2541524419408,-3.30155982299616));
#85596=CARTESIAN_POINT('Ctrl Pts',(12.5928726531297,32.1647898157427,-0.694647731280824));
#85597=CARTESIAN_POINT('Ctrl Pts',(13.041786012898,31.856755513104,2.04978659706714));
#85598=CARTESIAN_POINT('Ctrl Pts',(13.3410997224955,30.8761075302016,3.60877905448131));
#85599=CARTESIAN_POINT('Ctrl Pts',(13.4908137819219,30.2407658481206,4.24367794498727));
#85600=CARTESIAN_POINT('',(14.6544027596087,33.4246212024587,7.42462120245876));
#85601=CARTESIAN_POINT('',(11.5128100581662,18.5753788014852,-7.42462119851477));
#85602=CARTESIAN_POINT('Ctrl Pts',(11.5128101060189,18.5753787975412,-7.42462120245874));
#85603=CARTESIAN_POINT('Ctrl Pts',(11.6624097561899,19.6860995320808,-8.53534193699833));
#85604=CARTESIAN_POINT('Ctrl Pts',(11.9616090565318,22.4134943055532,-10.2487418519877));
#85605=CARTESIAN_POINT('Ctrl Pts',(12.4104080070446,27.2162233103119,-10.7922435813046));
#85606=CARTESIAN_POINT('Ctrl Pts',(12.8592069575574,31.7766088720556,-9.19360303844976));
#85607=CARTESIAN_POINT('Ctrl Pts',(13.3080059080703,35.1956718613173,-5.77830424746075));
#85608=CARTESIAN_POINT('Ctrl Pts',(13.7568048585831,36.7894395198819,-1.21575788028344));
#85609=CARTESIAN_POINT('Ctrl Pts',(14.2056038090959,36.2504682053753,3.58625167755849));
#85610=CARTESIAN_POINT('Ctrl Pts',(14.5048031094378,34.5353419369983,6.31390046791915));
#85611=CARTESIAN_POINT('Ctrl Pts',(14.6544027596087,33.4246212024587,7.42462120245876));
#85612=CARTESIAN_POINT('',(11.5128100131985,18.5753787975412,-7.42462120245874));
#85613=CARTESIAN_POINT('Ctrl Pts',(13.6199324221852,18.5753787975412,-7.42462120245874));
#85614=CARTESIAN_POINT('Ctrl Pts',(13.7695320723561,19.6860995320808,-8.53534193699833));
#85615=CARTESIAN_POINT('Ctrl Pts',(14.068731372698,22.4134943055532,-10.2487418519877));
#85616=CARTESIAN_POINT('Ctrl Pts',(14.5175303232108,27.2162233103119,-10.7922435813046));
#85617=CARTESIAN_POINT('Ctrl Pts',(14.9663292737237,31.7766088720556,-9.19360303844976));
#85618=CARTESIAN_POINT('Ctrl Pts',(15.4151282242365,35.1956718613173,-5.77830424746075));
#85619=CARTESIAN_POINT('Ctrl Pts',(15.8639271747493,36.7894395198819,-1.21575788028344));
#85620=CARTESIAN_POINT('Ctrl Pts',(16.3127261252621,36.2504682053753,3.58625167755849));
#85621=CARTESIAN_POINT('Ctrl Pts',(16.611925425604,34.5353419369983,6.31390046791915));
#85622=CARTESIAN_POINT('Ctrl Pts',(16.761525075775,33.4246212024587,7.42462120245876));
#85623=CARTESIAN_POINT('Ctrl Pts',(12.9175583167964,18.5753787975412,-7.42462120245874));
#85624=CARTESIAN_POINT('Ctrl Pts',(13.0671579669674,19.6860995320808,-8.53534193699833));
#85625=CARTESIAN_POINT('Ctrl Pts',(13.3663572673093,22.4134943055532,-10.2487418519877));
#85626=CARTESIAN_POINT('Ctrl Pts',(13.8151562178221,27.2162233103119,-10.7922435813046));
#85627=CARTESIAN_POINT('Ctrl Pts',(14.2639551683349,31.7766088720556,-9.19360303844975));
#85628=CARTESIAN_POINT('Ctrl Pts',(14.7127541188477,35.1956718613173,-5.77830424746075));
#85629=CARTESIAN_POINT('Ctrl Pts',(15.1615530693606,36.7894395198819,-1.21575788028343));
#85630=CARTESIAN_POINT('Ctrl Pts',(15.6103520198734,36.2504682053753,3.58625167755849));
#85631=CARTESIAN_POINT('Ctrl Pts',(15.9095513202153,34.5353419369983,6.31390046791915));
#85632=CARTESIAN_POINT('Ctrl Pts',(16.0591509703862,33.4246212024587,7.42462120245876));
#85633=CARTESIAN_POINT('Ctrl Pts',(12.2151842114077,18.5753787975412,-7.42462120245874));
#85634=CARTESIAN_POINT('Ctrl Pts',(12.3647838615786,19.6860995320808,-8.53534193699833));
#85635=CARTESIAN_POINT('Ctrl Pts',(12.6639831619205,22.4134943055532,-10.2487418519877));
#85636=CARTESIAN_POINT('Ctrl Pts',(13.1127821124333,27.2162233103119,-10.7922435813046));
#85637=CARTESIAN_POINT('Ctrl Pts',(13.5615810629462,31.7766088720556,-9.19360303844976));
#85638=CARTESIAN_POINT('Ctrl Pts',(14.010380013459,35.1956718613173,-5.77830424746075));
#85639=CARTESIAN_POINT('Ctrl Pts',(14.4591789639718,36.7894395198819,-1.21575788028344));
#85640=CARTESIAN_POINT('Ctrl Pts',(14.9079779144847,36.2504682053753,3.5862516775585));
#85641=CARTESIAN_POINT('Ctrl Pts',(15.2071772148265,34.5353419369983,6.31390046791915));
#85642=CARTESIAN_POINT('Ctrl Pts',(15.3567768649975,33.4246212024587,7.42462120245876));
#85643=CARTESIAN_POINT('Ctrl Pts',(11.5128101060189,18.5753787975412,-7.42462120245874));
#85644=CARTESIAN_POINT('Ctrl Pts',(11.6624097561899,19.6860995320808,-8.53534193699833));
#85645=CARTESIAN_POINT('Ctrl Pts',(11.9616090565318,22.4134943055532,-10.2487418519877));
#85646=CARTESIAN_POINT('Ctrl Pts',(12.4104080070446,27.2162233103119,-10.7922435813046));
#85647=CARTESIAN_POINT('Ctrl Pts',(12.8592069575574,31.7766088720556,-9.19360303844976));
#85648=CARTESIAN_POINT('Ctrl Pts',(13.3080059080703,35.1956718613173,-5.77830424746075));
#85649=CARTESIAN_POINT('Ctrl Pts',(13.7568048585831,36.7894395198819,-1.21575788028344));
#85650=CARTESIAN_POINT('Ctrl Pts',(14.2056038090959,36.2504682053753,3.58625167755849));
#85651=CARTESIAN_POINT('Ctrl Pts',(14.5048031094378,34.5353419369983,6.31390046791915));
#85652=CARTESIAN_POINT('Ctrl Pts',(14.6544027596087,33.4246212024587,7.42462120245876));
#85653=CARTESIAN_POINT('',(11.5128100131985,18.5753787975412,-7.42462120245874));
#85654=CARTESIAN_POINT('Ctrl Pts',(8.50027478292078,21.7560622709221,-4.24050518741127));
#85655=CARTESIAN_POINT('Ctrl Pts',(8.65000928932408,22.3910083689704,-4.87597404391553));
#85656=CARTESIAN_POINT('Ctrl Pts',(8.94934344589831,23.9499417862674,-5.85575499156164));
#85657=CARTESIAN_POINT('Ctrl Pts',(9.39827725264349,26.6949167687136,-6.1663814341434));
#85658=CARTESIAN_POINT('Ctrl Pts',(9.84707620315632,29.3005989330943,-5.25296850297538));
#85659=CARTESIAN_POINT('Ctrl Pts',(10.2958751536691,31.2541543256308,-3.30155412730028));
#85660=CARTESIAN_POINT('Ctrl Pts',(10.7446741041819,32.164797852443,-0.694642440642849));
#85661=CARTESIAN_POINT('Ctrl Pts',(11.193587522373,31.8567579459617,2.0497923910259));
#85662=CARTESIAN_POINT('Ctrl Pts',(11.492901290393,30.8761067554945,3.60877937042535));
#85663=CARTESIAN_POINT('Ctrl Pts',(11.6426154082421,30.2407647654735,4.2436783491607));
#85664=CARTESIAN_POINT('Ctrl Pts',(8.11229733977657,20.6948333956204,-5.30087572958818));
#85665=CARTESIAN_POINT('Ctrl Pts',(8.26203184617986,21.488552589912,-6.09524840205955));
#85666=CARTESIAN_POINT('Ctrl Pts',(8.56136600275409,23.4373091532399,-7.32003102020338));
#85667=CARTESIAN_POINT('Ctrl Pts',(9.01029980949927,26.8686859868238,-7.70833196494417));
#85668=CARTESIAN_POINT('Ctrl Pts',(9.4590987600121,30.125938774815,-6.56651319007399));
#85669=CARTESIAN_POINT('Ctrl Pts',(9.90789771052492,32.5679955366945,-4.12713282258988));
#85670=CARTESIAN_POINT('Ctrl Pts',(10.3566966610378,33.7063523966073,-0.868343060934558));
#85671=CARTESIAN_POINT('Ctrl Pts',(10.8056100792287,33.3212847709717,2.56235855306593));
#85672=CARTESIAN_POINT('Ctrl Pts',(11.1049238472488,32.0954142991773,4.51118207210694));
#85673=CARTESIAN_POINT('Ctrl Pts',(11.254637965098,31.3012002171171,5.30484236454325));
#85674=CARTESIAN_POINT('Ctrl Pts',(7.72431989663235,19.6336045203188,-6.36124627176508));
#85675=CARTESIAN_POINT('Ctrl Pts',(7.87405440303564,20.5860968108534,-7.31452276020356));
#85676=CARTESIAN_POINT('Ctrl Pts',(8.17338855960988,22.9246765202122,-8.78430704884514));
#85677=CARTESIAN_POINT('Ctrl Pts',(8.62232236635506,27.042455204934,-9.25028249574493));
#85678=CARTESIAN_POINT('Ctrl Pts',(9.07112131686788,30.9512786165357,-7.88005787717262));
#85679=CARTESIAN_POINT('Ctrl Pts',(9.51992026738071,33.8818367477582,-4.95271151787948));
#85680=CARTESIAN_POINT('Ctrl Pts',(9.96871921789354,35.2479069407715,-1.04204368122627));
#85681=CARTESIAN_POINT('Ctrl Pts',(10.4176326360845,34.7858115959818,3.07492471510595));
#85682=CARTESIAN_POINT('Ctrl Pts',(10.7169464041046,33.3147218428599,5.41358477378853));
#85683=CARTESIAN_POINT('Ctrl Pts',(10.8666605219537,32.3616356687608,6.3660063799258));
#85684=CARTESIAN_POINT('Ctrl Pts',(7.33634245348814,18.572375645017,-7.42161681394198));
#85685=CARTESIAN_POINT('Ctrl Pts',(7.48607695989143,19.6836410317949,-8.53379711834756));
#85686=CARTESIAN_POINT('Ctrl Pts',(7.78541111646566,22.4120438871847,-10.2485830774869));
#85687=CARTESIAN_POINT('Ctrl Pts',(8.23434492321084,27.2162244230442,-10.7922330265457));
#85688=CARTESIAN_POINT('Ctrl Pts',(8.68314387372367,31.7766184582563,-9.19360256427123));
#85689=CARTESIAN_POINT('Ctrl Pts',(9.13194282423649,35.1956779588219,-5.77829021316908));
#85690=CARTESIAN_POINT('Ctrl Pts',(9.58074177474933,36.7894614849358,-1.21574430151798));
#85691=CARTESIAN_POINT('Ctrl Pts',(10.0296551929403,36.2503384209919,3.58749087714597));
#85692=CARTESIAN_POINT('Ctrl Pts',(10.3289689609603,34.5340293865426,6.31598747547012));
#85693=CARTESIAN_POINT('Ctrl Pts',(10.4786830788095,33.4220711204044,7.42717039530835));
#85694=CARTESIAN_POINT('',(7.33674696088869,18.5753787991571,-7.42462120084289));
#85695=CARTESIAN_POINT('',(8.52638781740187,21.8280699909994,-4.17193000900062));
#85696=CARTESIAN_POINT('',(10.478339675775,33.4246212024587,7.42462120245876));
#85697=CARTESIAN_POINT('Ctrl Pts',(7.33674702218519,18.5753787975412,-7.42462120245874));
#85698=CARTESIAN_POINT('Ctrl Pts',(7.48634667235613,19.6860995320808,-8.53534193699833));
#85699=CARTESIAN_POINT('Ctrl Pts',(7.78554597269801,22.4134870257429,-10.2487463857135));
#85700=CARTESIAN_POINT('Ctrl Pts',(8.23434492321084,27.2162244230442,-10.7922330265457));
#85701=CARTESIAN_POINT('Ctrl Pts',(8.68314387372367,31.7766184582563,-9.19360256427123));
#85702=CARTESIAN_POINT('Ctrl Pts',(9.13194282423649,35.1956779588219,-5.77829021316908));
#85703=CARTESIAN_POINT('Ctrl Pts',(9.58074177474933,36.7894614849358,-1.21574430151798));
#85704=CARTESIAN_POINT('Ctrl Pts',(10.0295407252621,36.250475891076,3.58626610827892));
#85705=CARTESIAN_POINT('Ctrl Pts',(10.328740025604,34.5353419369983,6.31390046791915));
#85706=CARTESIAN_POINT('Ctrl Pts',(10.478339675775,33.4246212024587,7.42462120245876));
#85707=CARTESIAN_POINT('',(11.6679805638121,30.1719300090006,4.17193000900064));
#85708=CARTESIAN_POINT('Ctrl Pts',(5.22922008610955,18.5723752649374,-7.42161643355513));
#85709=CARTESIAN_POINT('Ctrl Pts',(5.37895460958362,19.6836407231716,-8.53379692106834));
#85710=CARTESIAN_POINT('Ctrl Pts',(5.67828878322864,22.4120408496955,-10.2485849356457));
#85711=CARTESIAN_POINT('Ctrl Pts',(6.12722260704461,27.2162246994806,-10.7922291011963));
#85712=CARTESIAN_POINT('Ctrl Pts',(6.57602155755744,31.7766218825448,-9.19360269140816));
#85713=CARTESIAN_POINT('Ctrl Pts',(7.02482050807027,35.1956799398728,-5.77828511785068));
#85714=CARTESIAN_POINT('Ctrl Pts',(7.4736194585831,36.7894695685334,-1.21573946002377));
#85715=CARTESIAN_POINT('Ctrl Pts',(7.9225324577569,36.2503415768864,3.58749169207723));
#85716=CARTESIAN_POINT('Ctrl Pts',(8.22184580675976,34.5340341899288,6.31597983204138));
#85717=CARTESIAN_POINT('Ctrl Pts',(8.37155950559168,33.4220804567874,7.42716106543041));
#85718=CARTESIAN_POINT('Ctrl Pts',(4.84124263456142,19.6336042175304,-6.36124592275786));
#85719=CARTESIAN_POINT('Ctrl Pts',(4.99097715803549,20.5860965658729,-7.3145225647003));
#85720=CARTESIAN_POINT('Ctrl Pts',(5.29031133168052,22.9246739278113,-8.78430860980025));
#85721=CARTESIAN_POINT('Ctrl Pts',(5.73924515549648,27.0424554381102,-9.25027909783365));
#85722=CARTESIAN_POINT('Ctrl Pts',(6.18804410600931,30.9512815336981,-7.88005795769227));
#85723=CARTESIAN_POINT('Ctrl Pts',(6.63684305652214,33.8818384173056,-4.95270713267683));
#85724=CARTESIAN_POINT('Ctrl Pts',(7.08564200703497,35.2479138360262,-1.04203952770266));
#85725=CARTESIAN_POINT('Ctrl Pts',(7.53455500620877,34.785814269252,3.07492540250052));
#85726=CARTESIAN_POINT('Ctrl Pts',(7.83386835521163,33.3147259335466,5.41357820287516));
#85727=CARTESIAN_POINT('Ctrl Pts',(7.98358205404355,32.3616436482293,6.36599836007736));
#85728=CARTESIAN_POINT('Ctrl Pts',(4.45326518301329,20.6948331701234,-5.30087541196059));
#85729=CARTESIAN_POINT('Ctrl Pts',(4.60299970648736,21.4885524085742,-6.09524820833226));
#85730=CARTESIAN_POINT('Ctrl Pts',(4.90233388013239,23.437307005927,-7.32003228395488));
#85731=CARTESIAN_POINT('Ctrl Pts',(5.35126770394836,26.86868617674,-7.70832909447099));
#85732=CARTESIAN_POINT('Ctrl Pts',(5.80006665446118,30.1259411848514,-6.56651322397638));
#85733=CARTESIAN_POINT('Ctrl Pts',(6.24886560497401,32.5679968947386,-4.12712914750298));
#85734=CARTESIAN_POINT('Ctrl Pts',(6.69766455548684,33.7063581035188,-0.868339595381541));
#85735=CARTESIAN_POINT('Ctrl Pts',(7.14657755466065,33.3212869616176,2.56235911292381));
#85736=CARTESIAN_POINT('Ctrl Pts',(7.4458909036635,32.0954176771643,4.51117657370893));
#85737=CARTESIAN_POINT('Ctrl Pts',(7.59560460249543,31.3012068396711,5.3048356547243));
#85738=CARTESIAN_POINT('Ctrl Pts',(4.06528773146516,21.7560621227164,-4.24050490116332));
#85739=CARTESIAN_POINT('Ctrl Pts',(4.21502225493925,22.3910082512754,-4.87597385196422));
#85740=CARTESIAN_POINT('Ctrl Pts',(4.51435642858426,23.9499400840428,-5.8557559581095));
#85741=CARTESIAN_POINT('Ctrl Pts',(4.96329025240023,26.6949169153697,-6.16637909110834));
#85742=CARTESIAN_POINT('Ctrl Pts',(5.41208920291306,29.3006008360047,-5.25296849026049));
#85743=CARTESIAN_POINT('Ctrl Pts',(5.86088815342589,31.2541553721714,-3.30155116232912));
#85744=CARTESIAN_POINT('Ctrl Pts',(6.30968710393871,32.1648023710115,-0.694639663060422));
#85745=CARTESIAN_POINT('Ctrl Pts',(6.75860010311252,31.8567596539832,2.0497928233471));
#85746=CARTESIAN_POINT('Ctrl Pts',(7.05791345211538,30.876109420782,3.60877494454271));
#85747=CARTESIAN_POINT('Ctrl Pts',(7.2076271509473,30.2407700311129,4.24367294937125));
#85748=CARTESIAN_POINT('',(8.37121735960874,33.4246212024587,7.42462120245876));
#85749=CARTESIAN_POINT('',(8.37121735960875,33.4246212024587,7.42462120245876));
#85750=CARTESIAN_POINT('',(5.22962465816628,18.5753788014852,-7.42462119851477));
#85751=CARTESIAN_POINT('Ctrl Pts',(5.22962470601896,18.5753787975412,-7.42462120245874));
#85752=CARTESIAN_POINT('Ctrl Pts',(5.3792243561899,19.6860995320808,-8.53534193699833));
#85753=CARTESIAN_POINT('Ctrl Pts',(5.67842365653178,22.4134870257429,-10.2487463857135));
#85754=CARTESIAN_POINT('Ctrl Pts',(6.12722260704461,27.2162244230442,-10.7922330265457));
#85755=CARTESIAN_POINT('Ctrl Pts',(6.57602155755744,31.7766184582563,-9.19360256427123));
#85756=CARTESIAN_POINT('Ctrl Pts',(7.02482050807026,35.1956779588219,-5.77829021316908));
#85757=CARTESIAN_POINT('Ctrl Pts',(7.47361945858309,36.7894614849358,-1.21574430151798));
#85758=CARTESIAN_POINT('Ctrl Pts',(7.92241840909592,36.250475891076,3.58626610827892));
#85759=CARTESIAN_POINT('Ctrl Pts',(8.22161770943781,34.5353419369983,6.31390046791915));
#85760=CARTESIAN_POINT('Ctrl Pts',(8.37121735960875,33.4246212024587,7.42462120245876));
#85761=CARTESIAN_POINT('',(5.22962461319854,18.5753787975412,-7.42462120245874));
#85762=CARTESIAN_POINT('Ctrl Pts',(7.33674702218519,18.5753787975412,-7.42462120245874));
#85763=CARTESIAN_POINT('Ctrl Pts',(7.48634667235613,19.6860995320808,-8.53534193699833));
#85764=CARTESIAN_POINT('Ctrl Pts',(7.78554597269801,22.4134870257429,-10.2487463857135));
#85765=CARTESIAN_POINT('Ctrl Pts',(8.23434492321084,27.2162244230442,-10.7922330265457));
#85766=CARTESIAN_POINT('Ctrl Pts',(8.68314387372367,31.7766184582563,-9.19360256427123));
#85767=CARTESIAN_POINT('Ctrl Pts',(9.13194282423649,35.1956779588219,-5.77829021316908));
#85768=CARTESIAN_POINT('Ctrl Pts',(9.58074177474933,36.7894614849358,-1.21574430151798));
#85769=CARTESIAN_POINT('Ctrl Pts',(10.0295407252621,36.250475891076,3.58626610827892));
#85770=CARTESIAN_POINT('Ctrl Pts',(10.328740025604,34.5353419369983,6.31390046791915));
#85771=CARTESIAN_POINT('Ctrl Pts',(10.478339675775,33.4246212024587,7.42462120245876));
#85772=CARTESIAN_POINT('Ctrl Pts',(6.63437291679644,18.5753787975412,-7.42462120245874));
#85773=CARTESIAN_POINT('Ctrl Pts',(6.78397256696739,19.6860995320808,-8.53534193699833));
#85774=CARTESIAN_POINT('Ctrl Pts',(7.08317186730927,22.4134870257429,-10.2487463857135));
#85775=CARTESIAN_POINT('Ctrl Pts',(7.5319708178221,27.2162244230442,-10.7922330265457));
#85776=CARTESIAN_POINT('Ctrl Pts',(7.98076976833493,31.7766184582563,-9.19360256427123));
#85777=CARTESIAN_POINT('Ctrl Pts',(8.42956871884775,35.1956779588219,-5.77829021316908));
#85778=CARTESIAN_POINT('Ctrl Pts',(8.87836766936058,36.7894614849358,-1.21574430151798));
#85779=CARTESIAN_POINT('Ctrl Pts',(9.3271666198734,36.250475891076,3.58626610827891));
#85780=CARTESIAN_POINT('Ctrl Pts',(9.62636592021529,34.5353419369983,6.31390046791915));
#85781=CARTESIAN_POINT('Ctrl Pts',(9.77596557038624,33.4246212024587,7.42462120245876));
#85782=CARTESIAN_POINT('Ctrl Pts',(5.9319988114077,18.5753787975412,-7.42462120245874));
#85783=CARTESIAN_POINT('Ctrl Pts',(6.08159846157864,19.6860995320808,-8.53534193699833));
#85784=CARTESIAN_POINT('Ctrl Pts',(6.38079776192053,22.4134870257429,-10.2487463857135));
#85785=CARTESIAN_POINT('Ctrl Pts',(6.82959671243335,27.2162244230442,-10.7922330265457));
#85786=CARTESIAN_POINT('Ctrl Pts',(7.27839566294618,31.7766184582563,-9.19360256427123));
#85787=CARTESIAN_POINT('Ctrl Pts',(7.72719461345901,35.1956779588219,-5.77829021316908));
#85788=CARTESIAN_POINT('Ctrl Pts',(8.17599356397184,36.7894614849358,-1.21574430151798));
#85789=CARTESIAN_POINT('Ctrl Pts',(8.62479251448466,36.250475891076,3.58626610827892));
#85790=CARTESIAN_POINT('Ctrl Pts',(8.92399181482655,34.5353419369983,6.31390046791915));
#85791=CARTESIAN_POINT('Ctrl Pts',(9.07359146499749,33.4246212024587,7.42462120245876));
#85792=CARTESIAN_POINT('Ctrl Pts',(5.22962470601896,18.5753787975412,-7.42462120245874));
#85793=CARTESIAN_POINT('Ctrl Pts',(5.3792243561899,19.6860995320808,-8.53534193699833));
#85794=CARTESIAN_POINT('Ctrl Pts',(5.67842365653178,22.4134870257429,-10.2487463857135));
#85795=CARTESIAN_POINT('Ctrl Pts',(6.12722260704461,27.2162244230442,-10.7922330265457));
#85796=CARTESIAN_POINT('Ctrl Pts',(6.57602155755744,31.7766184582563,-9.19360256427123));
#85797=CARTESIAN_POINT('Ctrl Pts',(7.02482050807026,35.1956779588219,-5.77829021316908));
#85798=CARTESIAN_POINT('Ctrl Pts',(7.47361945858309,36.7894614849358,-1.21574430151798));
#85799=CARTESIAN_POINT('Ctrl Pts',(7.92241840909592,36.250475891076,3.58626610827892));
#85800=CARTESIAN_POINT('Ctrl Pts',(8.22161770943781,34.5353419369983,6.31390046791915));
#85801=CARTESIAN_POINT('Ctrl Pts',(8.37121735960875,33.4246212024587,7.42462120245876));
#85802=CARTESIAN_POINT('',(5.22962461319854,18.5753787975412,-7.42462120245874));
#85803=CARTESIAN_POINT('',(8.37121735960875,33.4246212024587,7.42462120245876));
#85804=CARTESIAN_POINT('Ctrl Pts',(2.21708909116458,21.7560607660849,-4.24050270859201));
#85805=CARTESIAN_POINT('Ctrl Pts',(2.36682375409141,22.3910071569996,-4.8759724572093));
#85806=CARTESIAN_POINT('Ctrl Pts',(2.66615806718916,23.9499357751967,-5.85575779538566));
#85807=CARTESIAN_POINT('Ctrl Pts',(3.11509203045787,26.6949170540957,-6.16637363300278));
#85808=CARTESIAN_POINT('Ctrl Pts',(3.5638909809707,29.3006045977601,-5.25296843898344));
#85809=CARTESIAN_POINT('Ctrl Pts',(4.01268993148352,31.2541569977362,-3.30154467940645));
#85810=CARTESIAN_POINT('Ctrl Pts',(4.46148888199635,32.1648116395084,-0.694633848166408));
#85811=CARTESIAN_POINT('Ctrl Pts',(4.91040191516051,31.856762106403,2.04979928901456));
#85812=CARTESIAN_POINT('Ctrl Pts',(5.20971529815371,30.8761087161373,3.60877493875489));
#85813=CARTESIAN_POINT('Ctrl Pts',(5.35942903097598,30.2407691812814,4.2436729644246));
#85814=CARTESIAN_POINT('Ctrl Pts',(1.82911158874891,20.6948312307416,-5.3008729144373));
#85815=CARTESIAN_POINT('Ctrl Pts',(1.97884625167573,21.4885508335847,-6.09524674458824));
#85816=CARTESIAN_POINT('Ctrl Pts',(2.27818056477349,23.4373015019899,-7.3200349166553));
#85817=CARTESIAN_POINT('Ctrl Pts',(2.72711452804219,26.8686863900293,-7.70832262534693));
#85818=CARTESIAN_POINT('Ctrl Pts',(3.17591347855502,30.1259460766487,-6.56651346128885));
#85819=CARTESIAN_POINT('Ctrl Pts',(3.62471242906785,32.5679992282681,-4.12712123291655));
#85820=CARTESIAN_POINT('Ctrl Pts',(4.07351137958068,33.7063700434066,-0.868332366286651));
#85821=CARTESIAN_POINT('Ctrl Pts',(4.52242441274482,33.3212903633405,2.56236731299668));
#85822=CARTESIAN_POINT('Ctrl Pts',(4.82173779573804,32.0954170761057,4.51117677354287));
#85823=CARTESIAN_POINT('Ctrl Pts',(4.9714515285603,31.3012060206651,5.30483591704091));
#85824=CARTESIAN_POINT('Ctrl Pts',(1.44113408633323,19.6336016953983,-6.36124312028259));
#85825=CARTESIAN_POINT('Ctrl Pts',(1.59086874926006,20.5860945101698,-7.31452103196718));
#85826=CARTESIAN_POINT('Ctrl Pts',(1.89020306235781,22.924667228783,-8.78431203792493));
#85827=CARTESIAN_POINT('Ctrl Pts',(2.33913702562652,27.042455725963,-9.25027161769108));
#85828=CARTESIAN_POINT('Ctrl Pts',(2.78793597613934,30.9512875555375,-7.88005848359427));
#85829=CARTESIAN_POINT('Ctrl Pts',(3.23673492665217,33.8818414587999,-4.95269778642664));
#85830=CARTESIAN_POINT('Ctrl Pts',(3.685533877165,35.2479284473048,-1.0420308844069));
#85831=CARTESIAN_POINT('Ctrl Pts',(4.13444691032915,34.7858186202782,3.07493533697882));
#85832=CARTESIAN_POINT('Ctrl Pts',(4.43376029332236,33.314725436074,5.41357860833083));
#85833=CARTESIAN_POINT('Ctrl Pts',(4.58347402614463,32.3616428600489,6.36599886965723));
#85834=CARTESIAN_POINT('Ctrl Pts',(1.05315658391756,18.5723721600548,-7.42161332612787));
#85835=CARTESIAN_POINT('Ctrl Pts',(1.20289124684438,19.683638186755,-8.53379531934611));
#85836=CARTESIAN_POINT('Ctrl Pts',(1.50222555994213,22.4120329555762,-10.2485891591946));
#85837=CARTESIAN_POINT('Ctrl Pts',(1.95115952321084,27.2162250618967,-10.7922206100352));
#85838=CARTESIAN_POINT('Ctrl Pts',(2.39995847372367,31.7766290344261,-9.19360350589968));
#85839=CARTESIAN_POINT('Ctrl Pts',(2.8487574242365,35.1956836893318,-5.77827433993674));
#85840=CARTESIAN_POINT('Ctrl Pts',(3.29755637474933,36.7894868512029,-1.21572940252715));
#85841=CARTESIAN_POINT('Ctrl Pts',(3.74646940791347,36.2503468772158,3.58750336096094));
#85842=CARTESIAN_POINT('Ctrl Pts',(4.04578279090669,34.5340337960423,6.31598044311881));
#85843=CARTESIAN_POINT('Ctrl Pts',(4.19549652372895,33.4220796994326,7.42716182227354));
#85844=CARTESIAN_POINT('',(1.05356156088868,18.5753787991571,-7.42462120084289));
#85845=CARTESIAN_POINT('',(2.24320241740187,21.8280699909994,-4.17193000900062));
#85846=CARTESIAN_POINT('',(4.19515427577498,33.4246212024587,7.42462120245876));
#85847=CARTESIAN_POINT('Ctrl Pts',(1.05356162218519,18.5753787975412,-7.42462120245874));
#85848=CARTESIAN_POINT('Ctrl Pts',(1.20316127235613,19.6860995320808,-8.53534193699833));
#85849=CARTESIAN_POINT('Ctrl Pts',(1.50236057269802,22.4134777721174,-10.2487526513479));
#85850=CARTESIAN_POINT('Ctrl Pts',(1.95115952321084,27.2162250618967,-10.7922206100352));
#85851=CARTESIAN_POINT('Ctrl Pts',(2.39995847372367,31.7766290344261,-9.19360350589968));
#85852=CARTESIAN_POINT('Ctrl Pts',(2.8487574242365,35.1956836893318,-5.77827433993674));
#85853=CARTESIAN_POINT('Ctrl Pts',(3.29755637474932,36.7894868512029,-1.21572940252715));
#85854=CARTESIAN_POINT('Ctrl Pts',(3.74635532526215,36.2504838893164,3.58628271132926));
#85855=CARTESIAN_POINT('Ctrl Pts',(4.04555462560404,34.5353419369983,6.31390046791915));
#85856=CARTESIAN_POINT('Ctrl Pts',(4.19515427577498,33.4246212024587,7.42462120245876));
#85857=CARTESIAN_POINT('',(5.38479516381208,30.1719300090006,4.17193000900064));
#85858=CARTESIAN_POINT('Ctrl Pts',(-1.0539654241159,18.5723702242316,-7.42161366308853));
#85859=CARTESIAN_POINT('Ctrl Pts',(-0.904230725318819,19.683636569112,-8.53379621253979));
#85860=CARTESIAN_POINT('Ctrl Pts',(-0.60489637635079,22.4120283617824,-10.2485932995738));
#85861=CARTESIAN_POINT('Ctrl Pts',(-0.155962377211819,27.2162253197193,
-10.7922175564503));
#85862=CARTESIAN_POINT('Ctrl Pts',(0.292836573301009,31.7766337359551,-9.19360566949464));
#85863=CARTESIAN_POINT('Ctrl Pts',(0.741635523813836,35.1956868609254,-5.77826939950743));
#85864=CARTESIAN_POINT('Ctrl Pts',(1.19043447432666,36.789497943561,-1.21572426912529));
#85865=CARTESIAN_POINT('Ctrl Pts',(1.63934707394011,36.2503516882648,3.58750543382354));
#85866=CARTESIAN_POINT('Ctrl Pts',(1.93866002338263,34.5340400726463,6.31597350110576));
#85867=CARTESIAN_POINT('Ctrl Pts',(2.08837332265419,33.4220904959639,7.42715330588487));
#85868=CARTESIAN_POINT('Ctrl Pts',(-1.44194308063557,19.6336002952009,-6.36124315026631));
#85869=CARTESIAN_POINT('Ctrl Pts',(-1.29220838183848,20.5860933439363,-7.31452149992352));
#85870=CARTESIAN_POINT('Ctrl Pts',(-0.992874032870451,22.9246634164647,
-8.78431522931743));
#85871=CARTESIAN_POINT('Ctrl Pts',(-0.54394003373148,27.0424559045324,-9.25026862400477));
#85872=CARTESIAN_POINT('Ctrl Pts',(-0.0951410832186525,30.9512913838673,
-7.88006001743081));
#85873=CARTESIAN_POINT('Ctrl Pts',(0.353657867294175,33.8818438565437,-4.95269335034525));
#85874=CARTESIAN_POINT('Ctrl Pts',(0.802456817807003,35.247937578541,-1.04202644204568));
#85875=CARTESIAN_POINT('Ctrl Pts',(1.25136941742045,34.7858223864565,3.07493698856269));
#85876=CARTESIAN_POINT('Ctrl Pts',(1.55068236686297,33.3147305182722,5.41357243789115));
#85877=CARTESIAN_POINT('Ctrl Pts',(1.70039566613453,32.3616518551653,6.3659913110293));
#85878=CARTESIAN_POINT('Ctrl Pts',(-1.82992073715523,20.69483036617,-5.30087263744408));
#85879=CARTESIAN_POINT('Ctrl Pts',(-1.68018603835815,21.4885501187606,-6.09524678730726));
#85880=CARTESIAN_POINT('Ctrl Pts',(-1.38085168939011,23.4372984711471,-7.32003715906107));
#85881=CARTESIAN_POINT('Ctrl Pts',(-0.931917690251141,26.8686864893455,
-7.70831969155928));
#85882=CARTESIAN_POINT('Ctrl Pts',(-0.483118739738314,30.1259490317793,
-6.566514365367));
#85883=CARTESIAN_POINT('Ctrl Pts',(-0.0343197892254864,32.5680008521621,
-4.12711730118307));
#85884=CARTESIAN_POINT('Ctrl Pts',(0.414479161287341,33.706377213521,-0.868328614966077));
#85885=CARTESIAN_POINT('Ctrl Pts',(0.863391760900794,33.3212930846483,2.56236854330184));
#85886=CARTESIAN_POINT('Ctrl Pts',(1.1627047103433,32.0954209638981,4.51117137467655));
#85887=CARTESIAN_POINT('Ctrl Pts',(1.31241800961487,31.3012132143666,5.30482931617372));
#85888=CARTESIAN_POINT('Ctrl Pts',(-2.21789839367489,21.7560604371392,-4.24050212462184));
#85889=CARTESIAN_POINT('Ctrl Pts',(-2.0681636948778,22.3910068935847,-4.87597207469099));
#85890=CARTESIAN_POINT('Ctrl Pts',(-1.76882934590978,23.9499335258294,-5.8557590888047));
#85891=CARTESIAN_POINT('Ctrl Pts',(-1.3198953467708,26.6949170741586,-6.16637075911378));
#85892=CARTESIAN_POINT('Ctrl Pts',(-0.871096396257976,29.3006066796915,
-5.25296871330317));
#85893=CARTESIAN_POINT('Ctrl Pts',(-0.422297445745148,31.2541578477804,
-3.30154125202089));
#85894=CARTESIAN_POINT('Ctrl Pts',(0.0265015047676796,32.164816848501,-0.694630787886463));
#85895=CARTESIAN_POINT('Ctrl Pts',(0.475414104381133,31.8567637828401,2.04980009804098));
#85896=CARTESIAN_POINT('Ctrl Pts',(0.774727053823643,30.8761114095239,3.60877031146195));
#85897=CARTESIAN_POINT('Ctrl Pts',(0.924440353095209,30.240774573568,4.24366732131814));
#85898=CARTESIAN_POINT('',(2.08803195960875,33.4246212024587,7.42462120245876));
#85899=CARTESIAN_POINT('',(2.08803195960875,33.4246212024587,7.42462120245876));
#85900=CARTESIAN_POINT('',(-1.05356074183372,18.5753788014852,-7.42462119851477));
#85901=CARTESIAN_POINT('Ctrl Pts',(-1.05356069398104,18.5753787975412,-7.42462120245874));
#85902=CARTESIAN_POINT('Ctrl Pts',(-0.923480593410918,19.5411742702521,
-8.39041667516965));
#85903=CARTESIAN_POINT('Ctrl Pts',(-0.793390386445168,20.6983162097813,
-9.16424028291836));
#85904=CARTESIAN_POINT('Ctrl Pts',(-0.514417007370215,23.4005592311826,
-10.293571643669));
#85905=CARTESIAN_POINT('Ctrl Pts',(-0.383476568361032,24.789559828435,-10.495214302546));
#85906=CARTESIAN_POINT('Ctrl Pts',(-0.10475646414209,27.7160925620855,-10.508047074406));
#85907=CARTESIAN_POINT('Ctrl Pts',(0.0293830968989478,29.0939459047543,
-10.0808266335395));
#85908=CARTESIAN_POINT('Ctrl Pts',(0.2550250052573,31.2849952676692,-9.17859210179942));
#85909=CARTESIAN_POINT('Ctrl Pts',(0.385396446792777,32.4450836887615,-8.40289350048829));
#85910=CARTESIAN_POINT('Ctrl Pts',(0.649104132018911,34.4038383988825,-6.44526974701288));
#85911=CARTESIAN_POINT('Ctrl Pts',(0.779361426258769,35.1789943402779,-5.28667072334708));
#85912=CARTESIAN_POINT('Ctrl Pts',(1.00998133826083,36.099849591882,-3.04686683603461));
#85913=CARTESIAN_POINT('Ctrl Pts',(1.14347962089245,36.5054107499014,-1.67135405526916));
#85914=CARTESIAN_POINT('Ctrl Pts',(1.4145748299214,36.4953815121046,1.17517952963133));
#85915=CARTESIAN_POINT('Ctrl Pts',(1.54629654869269,36.3052557276413,2.5745604504923));
#85916=CARTESIAN_POINT('Ctrl Pts',(1.82814073845306,35.1632292264153,5.30408588680117));
#85917=CARTESIAN_POINT('Ctrl Pts',(1.95809258149138,34.3893718642633,6.45987054065415));
#85918=CARTESIAN_POINT('Ctrl Pts',(2.08803195960875,33.4246212024587,7.42462120245876));
#85919=CARTESIAN_POINT('',(-1.05356078680146,18.5753787975412,-7.42462120245874));
#85920=CARTESIAN_POINT('Ctrl Pts',(1.05356162218519,18.5753787975412,-7.42462120245874));
#85921=CARTESIAN_POINT('Ctrl Pts',(1.20316127235613,19.6860995320808,-8.53534193699833));
#85922=CARTESIAN_POINT('Ctrl Pts',(1.50236057269802,22.4134777721174,-10.2487526513479));
#85923=CARTESIAN_POINT('Ctrl Pts',(1.95115952321084,27.2162250618967,-10.7922206100352));
#85924=CARTESIAN_POINT('Ctrl Pts',(2.39995847372367,31.7766290344261,-9.19360350589968));
#85925=CARTESIAN_POINT('Ctrl Pts',(2.8487574242365,35.1956836893318,-5.77827433993674));
#85926=CARTESIAN_POINT('Ctrl Pts',(3.29755637474932,36.7894868512029,-1.21572940252715));
#85927=CARTESIAN_POINT('Ctrl Pts',(3.74635532526215,36.2504838893164,3.58628271132926));
#85928=CARTESIAN_POINT('Ctrl Pts',(4.04555462560404,34.5353419369983,6.31390046791915));
#85929=CARTESIAN_POINT('Ctrl Pts',(4.19515427577498,33.4246212024587,7.42462120245876));
#85930=CARTESIAN_POINT('Ctrl Pts',(0.35118671899054,18.5753787975412,-7.42462120245874));
#85931=CARTESIAN_POINT('Ctrl Pts',(0.500786369161483,19.6860995320808,-8.53534193699833));
#85932=CARTESIAN_POINT('Ctrl Pts',(0.799985669503367,22.4134777721174,-10.2487526513479));
#85933=CARTESIAN_POINT('Ctrl Pts',(1.2487846200162,27.2162250618967,-10.7922206100352));
#85934=CARTESIAN_POINT('Ctrl Pts',(1.69758357052903,31.7766290344261,-9.19360350589968));
#85935=CARTESIAN_POINT('Ctrl Pts',(2.14638252104185,35.1956836893318,-5.77827433993674));
#85936=CARTESIAN_POINT('Ctrl Pts',(2.59518147155468,36.7894868512029,-1.21572940252715));
#85937=CARTESIAN_POINT('Ctrl Pts',(3.04398042206751,36.2504838893164,3.58628271132925));
#85938=CARTESIAN_POINT('Ctrl Pts',(3.34317972240939,34.5353419369983,6.31390046791915));
#85939=CARTESIAN_POINT('Ctrl Pts',(3.49277937258034,33.4246212024587,7.42462120245876));
#85940=CARTESIAN_POINT('Ctrl Pts',(-0.351188184204108,18.5753787975412,
-7.42462120245874));
#85941=CARTESIAN_POINT('Ctrl Pts',(-0.201588534033165,19.6860995320808,
-8.53534193699833));
#85942=CARTESIAN_POINT('Ctrl Pts',(0.0976107663087195,22.4134777721174,
-10.2487526513479));
#85943=CARTESIAN_POINT('Ctrl Pts',(0.546409716821547,27.2162250618966,-10.7922206100352));
#85944=CARTESIAN_POINT('Ctrl Pts',(0.995208667334374,31.7766290344261,-9.19360350589968));
#85945=CARTESIAN_POINT('Ctrl Pts',(1.4440076178472,35.1956836893318,-5.77827433993674));
#85946=CARTESIAN_POINT('Ctrl Pts',(1.89280656836003,36.7894868512029,-1.21572940252715));
#85947=CARTESIAN_POINT('Ctrl Pts',(2.34160551887286,36.2504838893164,3.58628271132926));
#85948=CARTESIAN_POINT('Ctrl Pts',(2.64080481921474,34.5353419369983,6.31390046791915));
#85949=CARTESIAN_POINT('Ctrl Pts',(2.79040446938568,33.4246212024587,7.42462120245876));
#85950=CARTESIAN_POINT('Ctrl Pts',(-1.05356308739875,18.5753787975412,-7.42462120245874));
#85951=CARTESIAN_POINT('Ctrl Pts',(-0.903963437227813,19.6860995320808,
-8.53534193699833));
#85952=CARTESIAN_POINT('Ctrl Pts',(-0.604764136885928,22.4134777721174,
-10.2487526513479));
#85953=CARTESIAN_POINT('Ctrl Pts',(-0.1559651863731,27.2162250618967,-10.7922206100352));
#85954=CARTESIAN_POINT('Ctrl Pts',(0.292833764139727,31.7766290344261,-9.19360350589968));
#85955=CARTESIAN_POINT('Ctrl Pts',(0.741632714652555,35.1956836893318,-5.77827433993674));
#85956=CARTESIAN_POINT('Ctrl Pts',(1.19043166516538,36.7894868512029,-1.21572940252715));
#85957=CARTESIAN_POINT('Ctrl Pts',(1.63923061567821,36.2504838893164,3.58628271132926));
#85958=CARTESIAN_POINT('Ctrl Pts',(1.9384299160201,34.5353419369983,6.31390046791915));
#85959=CARTESIAN_POINT('Ctrl Pts',(2.08802956619104,33.4246212024587,7.42462120245876));
#85960=CARTESIAN_POINT('',(-1.05356078680146,18.5753787975412,-7.42462120245874));
#85961=CARTESIAN_POINT('',(2.08803195960875,33.4246212024587,7.42462120245876));
#85962=CARTESIAN_POINT('Ctrl Pts',(-4.06609633692487,21.7560606212036,-4.24050246993839));
#85963=CARTESIAN_POINT('Ctrl Pts',(-3.91636165892841,22.3910070403042,-4.87597230443958));
#85964=CARTESIAN_POINT('Ctrl Pts',(-3.61702733076101,23.9499352084937,-5.8557580717418));
#85965=CARTESIAN_POINT('Ctrl Pts',(-3.16809335242267,26.694917060818,-6.16637292099771));
#85966=CARTESIAN_POINT('Ctrl Pts',(-2.71929440190984,29.3006050890309,-5.25296847347605));
#85967=CARTESIAN_POINT('Ctrl Pts',(-2.27049545139702,31.2541571927175,-3.30154384028647));
#85968=CARTESIAN_POINT('Ctrl Pts',(-1.82169650088419,32.1648128688101,-0.694633102948697));
#85969=CARTESIAN_POINT('Ctrl Pts',(-1.37278350126161,31.8567624461033,2.04979990866951));
#85970=CARTESIAN_POINT('Ctrl Pts',(-1.07347015180998,30.8761088818321,3.60877454888744));
#85971=CARTESIAN_POINT('Ctrl Pts',(-0.923756452529281,30.2407695615107,
4.24367249087768));
#85972=CARTESIAN_POINT('Ctrl Pts',(-4.45407384504702,20.6948310223133,-5.30087264340261));
#85973=CARTESIAN_POINT('Ctrl Pts',(-4.30433916705057,21.4885506644777,-6.0952465850039));
#85974=CARTESIAN_POINT('Ctrl Pts',(-4.00500483888317,23.437300780382,-7.32003529980991));
#85975=CARTESIAN_POINT('Ctrl Pts',(-3.55607086054484,26.8686864029058,-7.70832177499247));
#85976=CARTESIAN_POINT('Ctrl Pts',(-3.10727191003201,30.1259467120115,-6.56651353821995));
#85977=CARTESIAN_POINT('Ctrl Pts',(-2.65847295951918,32.5679995058269,-4.12712020522022));
#85978=CARTESIAN_POINT('Ctrl Pts',(-2.20967400900635,33.7063716197874,-0.868331439192896));
#85979=CARTESIAN_POINT('Ctrl Pts',(-1.76076100938378,33.3212908256856,2.56236810079568));
#85980=CARTESIAN_POINT('Ctrl Pts',(-1.46144765993214,32.0954173146212,4.51117630941575));
#85981=CARTESIAN_POINT('Ctrl Pts',(-1.31173396065144,31.3012065232716,5.30483535239647));
#85982=CARTESIAN_POINT('Ctrl Pts',(-4.84205135316919,19.6336014234231,-6.36124281686683));
#85983=CARTESIAN_POINT('Ctrl Pts',(-4.69231667517274,20.5860942886512,-7.31452086556822));
#85984=CARTESIAN_POINT('Ctrl Pts',(-4.39298234700534,22.9246663522705,-8.78431252787802));
#85985=CARTESIAN_POINT('Ctrl Pts',(-3.94404836866699,27.0424557449935,-9.25027062898723));
#85986=CARTESIAN_POINT('Ctrl Pts',(-3.49524941815416,30.9512883349922,-7.88005860296385));
#85987=CARTESIAN_POINT('Ctrl Pts',(-3.04645046764134,33.8818418189363,-4.95269657015396));
#85988=CARTESIAN_POINT('Ctrl Pts',(-2.59765151712851,35.2479303707647,-1.04202977543709));
#85989=CARTESIAN_POINT('Ctrl Pts',(-2.14873851750593,34.7858192052677,3.07493629292183));
#85990=CARTESIAN_POINT('Ctrl Pts',(-1.8494251680543,33.3147257474102,5.41357806994405));
#85991=CARTESIAN_POINT('Ctrl Pts',(-1.6997114687736,32.3616434850324,6.36599821391526));
#85992=CARTESIAN_POINT('Ctrl Pts',(-5.23002886129135,18.5723718245327,-7.42161299033105));
#85993=CARTESIAN_POINT('Ctrl Pts',(-5.0802941832949,19.6836379128248,-8.53379514613253));
#85994=CARTESIAN_POINT('Ctrl Pts',(-4.7809598551275,22.4120319241589,-10.2485897559461));
#85995=CARTESIAN_POINT('Ctrl Pts',(-4.33202587678916,27.2162250870813,-10.792219482982));
#85996=CARTESIAN_POINT('Ctrl Pts',(-3.88322692627633,31.7766299579729,-9.19360366770775));
#85997=CARTESIAN_POINT('Ctrl Pts',(-3.4344279757635,35.1956841320457,-5.77827293508771));
#85998=CARTESIAN_POINT('Ctrl Pts',(-2.98562902525068,36.7894891217421,-1.21572811168129));
#85999=CARTESIAN_POINT('Ctrl Pts',(-2.5367160256281,36.25034758485,3.58750448504799));
#86000=CARTESIAN_POINT('Ctrl Pts',(-2.23740267617646,34.5340341801993,6.31597983047236));
#86001=CARTESIAN_POINT('Ctrl Pts',(-2.08768897689577,33.4220804467933,7.42716107543405));
#86002=CARTESIAN_POINT('',(-5.22962383911132,18.5753787991571,-7.42462120084288));
#86003=CARTESIAN_POINT('',(-4.03998298259813,21.8280699909994,-4.17193000900062));
#86004=CARTESIAN_POINT('',(-2.08803112422502,33.4246212024587,7.42462120245876));
#86005=CARTESIAN_POINT('Ctrl Pts',(-5.22962377781481,18.5753787975412,-7.42462120245874));
#86006=CARTESIAN_POINT('Ctrl Pts',(-5.08002412764387,19.6860995320808,-8.53534193699833));
#86007=CARTESIAN_POINT('Ctrl Pts',(-4.93042391721014,21.0497898200314,-9.39204650881968));
#86008=CARTESIAN_POINT('Ctrl Pts',(-4.78082437558953,22.5320924911443,-9.91097757957131));
#86009=CARTESIAN_POINT('Ctrl Pts',(-4.63122483396892,24.0143951622573,-10.4299086503229));
#86010=CARTESIAN_POINT('Ctrl Pts',(-4.4816254109829,25.6153102292322,-10.6110638876134));
#86011=CARTESIAN_POINT('Ctrl Pts',(-4.33202591030011,27.1758341851912,-10.4352058503029));
#86012=CARTESIAN_POINT('Ctrl Pts',(-4.18242640961732,28.7363581411502,-10.2593478129924));
#86013=CARTESIAN_POINT('Ctrl Pts',(-4.03282683881772,30.2564924773674,-9.72647664573263));
#86014=CARTESIAN_POINT('Ctrl Pts',(-3.88322710462072,31.5864020319258,-8.89081910296247));
#86015=CARTESIAN_POINT('Ctrl Pts',(-3.73362737042372,32.9163115864842,-8.05516156019232));
#86016=CARTESIAN_POINT('Ctrl Pts',(-3.58402803875759,34.0559964457548,-6.91671962854987));
#86017=CARTESIAN_POINT('Ctrl Pts',(-3.4344283002626,34.8914722949544,-5.58707487977672));
#86018=CARTESIAN_POINT('Ctrl Pts',(-3.28482856176761,35.7269481441539,-4.25743013100356));
#86019=CARTESIAN_POINT('Ctrl Pts',(-3.13522807006066,36.258214271152,-2.73658183224548));
#86020=CARTESIAN_POINT('Ctrl Pts',(-2.98562808753307,36.4340142951492,-1.17582236661662));
#86021=CARTESIAN_POINT('Ctrl Pts',(-2.83602810500547,36.6098143191465,0.384937099012241));
#86022=CARTESIAN_POINT('Ctrl Pts',(-2.68642868171361,36.4301482037352,1.98560771006104));
#86023=CARTESIAN_POINT('Ctrl Pts',(-2.53682930086399,35.9115301168794,3.46784855547023));
#86024=CARTESIAN_POINT('Ctrl Pts',(-2.38722992001438,35.3929120300235,4.95008940087942));
#86025=CARTESIAN_POINT('Ctrl Pts',(-2.23763077439596,34.5353419369983,6.31390046791915));
#86026=CARTESIAN_POINT('Ctrl Pts',(-2.08803112422502,33.4246212024587,7.42462120245876));
#86027=CARTESIAN_POINT('',(-0.898390236187925,30.1719300090006,4.17193000900064));
#86028=CARTESIAN_POINT('Ctrl Pts',(-7.33715091171646,18.5723737967529,-7.42161496416937));
#86029=CARTESIAN_POINT('Ctrl Pts',(-7.18741632230038,19.6836395245258,-8.53379616319783));
#86030=CARTESIAN_POINT('Ctrl Pts',(-6.88808208271336,22.412036304676,-10.2485874615845));
#86031=CARTESIAN_POINT('Ctrl Pts',(-6.43914819295539,27.2162249558894,-10.7922239637205));
#86032=CARTESIAN_POINT('Ctrl Pts',(-5.99034924244256,31.7766262509208,-9.19360309786621));
#86033=CARTESIAN_POINT('Ctrl Pts',(-5.54155029192973,35.1956822959411,-5.77827855619686));
#86034=CARTESIAN_POINT('Ctrl Pts',(-5.09275134141691,36.7894800611825,-1.21573330540808));
#86035=CARTESIAN_POINT('Ctrl Pts',(-4.64383850166433,36.2503450657148,3.58749685357029));
#86036=CARTESIAN_POINT('Ctrl Pts',(-4.34452531208268,34.5340360157071,6.3159769203004));
#86037=CARTESIAN_POINT('Ctrl Pts',(-4.19481177267199,33.4220840089498,7.42715751574294));
#86038=CARTESIAN_POINT('Ctrl Pts',(-7.72512838823515,19.6336030274158,-6.36124459506567));
#86039=CARTESIAN_POINT('Ctrl Pts',(-7.57539379881907,20.5860955965676,-7.31452183663775));
#86040=CARTESIAN_POINT('Ctrl Pts',(-7.27605955923203,22.9246700651593,-8.7843106806011));
#86041=CARTESIAN_POINT('Ctrl Pts',(-6.82712566947407,27.0424556467005,-9.25027459513849));
#86042=CARTESIAN_POINT('Ctrl Pts',(-6.37832671896124,30.9512852248186,-7.8800582215364));
#86043=CARTESIAN_POINT('Ctrl Pts',(-5.92952776844841,33.8818403521886,-4.95270145539072));
#86044=CARTESIAN_POINT('Ctrl Pts',(-5.48072881793558,35.247922730312,-1.04203424125412));
#86045=CARTESIAN_POINT('Ctrl Pts',(-5.03181597818301,34.7858171653526,3.07492979355112));
#86046=CARTESIAN_POINT('Ctrl Pts',(-4.73250278860136,33.3147274199893,5.41357564907264));
#86047=CARTESIAN_POINT('Ctrl Pts',(-4.58278924919067,32.3616466246225,6.36599524925758));
#86048=CARTESIAN_POINT('Ctrl Pts',(-8.11310586475383,20.6948322580786,-5.30087422596197));
#86049=CARTESIAN_POINT('Ctrl Pts',(-7.96337127533775,21.4885516686094,-6.09524751007768));
#86050=CARTESIAN_POINT('Ctrl Pts',(-7.66403703575072,23.4373038256427,-7.32003389961774));
#86051=CARTESIAN_POINT('Ctrl Pts',(-7.21510314599275,26.8686863375116,-7.70832522655642));
#86052=CARTESIAN_POINT('Ctrl Pts',(-6.76630419547992,30.1259441987164,-6.56651334520659));
#86053=CARTESIAN_POINT('Ctrl Pts',(-6.3175052449671,32.5679984084359,-4.12712435458457));
#86054=CARTESIAN_POINT('Ctrl Pts',(-5.86870629445427,33.7063653994416,-0.868335177100162));
#86055=CARTESIAN_POINT('Ctrl Pts',(-5.41979345470168,33.3212892649903,2.56236273353193));
#86056=CARTESIAN_POINT('Ctrl Pts',(-5.12048026512005,32.0954188242716,4.51117437784488));
#86057=CARTESIAN_POINT('Ctrl Pts',(-4.97076672570934,31.301209240295,5.30483298277222));
#86058=CARTESIAN_POINT('Ctrl Pts',(-8.50108334127251,21.7560614887415,-4.24050385685827));
#86059=CARTESIAN_POINT('Ctrl Pts',(-8.35134875185642,22.3910077406511,-4.87597318351759));
#86060=CARTESIAN_POINT('Ctrl Pts',(-8.05201451226939,23.949937586126,-5.85575711863438));
#86061=CARTESIAN_POINT('Ctrl Pts',(-7.60308062251143,26.6949170283227,-6.16637585797436));
#86062=CARTESIAN_POINT('Ctrl Pts',(-7.1542816719986,29.3006031726142,-5.25296846887678));
#86063=CARTESIAN_POINT('Ctrl Pts',(-6.70548272148578,31.2541564646834,-3.30154725377842));
#86064=CARTESIAN_POINT('Ctrl Pts',(-6.25668377097295,32.1648080685711,-0.694636112946202));
#86065=CARTESIAN_POINT('Ctrl Pts',(-5.80777093122036,31.856761364628,2.04979567351274));
#86066=CARTESIAN_POINT('Ctrl Pts',(-5.50845774163872,30.8761102285537,3.60877310661714));
#86067=CARTESIAN_POINT('Ctrl Pts',(-5.35874420222803,30.2407718559677,4.24367071628685));
#86068=CARTESIAN_POINT('',(-4.19515344039126,33.4246212024587,7.42462120245876));
#86069=CARTESIAN_POINT('',(-4.19515344039125,33.4246212024587,7.42462120245876));
#86070=CARTESIAN_POINT('',(-7.33674614183372,18.5753788014852,-7.42462119851477));
#86071=CARTESIAN_POINT('Ctrl Pts',(-7.33674609398104,18.5753787975412,-7.42462120245874));
#86072=CARTESIAN_POINT('Ctrl Pts',(-7.1871464438101,19.6860995320808,-8.53534193699833));
#86073=CARTESIAN_POINT('Ctrl Pts',(-6.88794714346822,22.4134803337522,-10.2487508662659));
#86074=CARTESIAN_POINT('Ctrl Pts',(-6.43914819295539,27.2162249558894,-10.7922239637205));
#86075=CARTESIAN_POINT('Ctrl Pts',(-5.99034924244256,31.7766262509208,-9.19360309786621));
#86076=CARTESIAN_POINT('Ctrl Pts',(-5.54155029192973,35.1956822959411,-5.77827855619686));
#86077=CARTESIAN_POINT('Ctrl Pts',(-5.09275134141691,36.7894800611825,-1.21573330540808));
#86078=CARTESIAN_POINT('Ctrl Pts',(-4.64395239090408,36.250481844326,3.58627827351926));
#86079=CARTESIAN_POINT('Ctrl Pts',(-4.34475309056219,34.5353419369983,6.31390046791915));
#86080=CARTESIAN_POINT('Ctrl Pts',(-4.19515344039125,33.4246212024587,7.42462120245876));
#86081=CARTESIAN_POINT('',(-7.33674618680146,18.5753787975412,-7.42462120245874));
#86082=CARTESIAN_POINT('Ctrl Pts',(-5.22962377781481,18.5753787975412,-7.42462120245874));
#86083=CARTESIAN_POINT('Ctrl Pts',(-5.08002412764387,19.6860995320808,-8.53534193699833));
#86084=CARTESIAN_POINT('Ctrl Pts',(-4.78082482730198,22.4134803337522,-10.2487508662659));
#86085=CARTESIAN_POINT('Ctrl Pts',(-4.33202587678916,27.2162249558894,-10.7922239637205));
#86086=CARTESIAN_POINT('Ctrl Pts',(-3.88322692627633,31.7766262509208,-9.19360309786621));
#86087=CARTESIAN_POINT('Ctrl Pts',(-3.4344279757635,35.1956822959411,-5.77827855619686));
#86088=CARTESIAN_POINT('Ctrl Pts',(-2.98562902525067,36.7894800611825,-1.21573330540808));
#86089=CARTESIAN_POINT('Ctrl Pts',(-2.53683007473785,36.250481844326,3.58627827351926));
#86090=CARTESIAN_POINT('Ctrl Pts',(-2.23763077439596,34.5353419369983,6.31390046791915));
#86091=CARTESIAN_POINT('Ctrl Pts',(-2.08803112422502,33.4246212024587,7.42462120245876));
#86092=CARTESIAN_POINT('Ctrl Pts',(-5.93199788320355,18.5753787975412,-7.42462120245874));
#86093=CARTESIAN_POINT('Ctrl Pts',(-5.78239823303261,19.6860995320808,-8.53534193699833));
#86094=CARTESIAN_POINT('Ctrl Pts',(-5.48319893269072,22.4134803337522,-10.2487508662659));
#86095=CARTESIAN_POINT('Ctrl Pts',(-5.0343999821779,27.2162249558894,-10.7922239637205));
#86096=CARTESIAN_POINT('Ctrl Pts',(-4.58560103166507,31.7766262509208,-9.19360309786621));
#86097=CARTESIAN_POINT('Ctrl Pts',(-4.13680208115225,35.1956822959411,-5.77827855619686));
#86098=CARTESIAN_POINT('Ctrl Pts',(-3.68800313063942,36.7894800611825,-1.21573330540808));
#86099=CARTESIAN_POINT('Ctrl Pts',(-3.23920418012659,36.250481844326,3.58627827351926));
#86100=CARTESIAN_POINT('Ctrl Pts',(-2.94000487978471,34.5353419369983,6.31390046791915));
#86101=CARTESIAN_POINT('Ctrl Pts',(-2.79040522961376,33.4246212024587,7.42462120245876));
#86102=CARTESIAN_POINT('Ctrl Pts',(-6.6343719885923,18.5753787975412,-7.42462120245874));
#86103=CARTESIAN_POINT('Ctrl Pts',(-6.48477233842136,19.6860995320808,-8.53534193699833));
#86104=CARTESIAN_POINT('Ctrl Pts',(-6.18557303807947,22.4134803337522,-10.2487508662659));
#86105=CARTESIAN_POINT('Ctrl Pts',(-5.73677408756665,27.2162249558894,-10.7922239637205));
#86106=CARTESIAN_POINT('Ctrl Pts',(-5.28797513705382,31.7766262509208,-9.19360309786621));
#86107=CARTESIAN_POINT('Ctrl Pts',(-4.83917618654099,35.1956822959411,-5.77827855619686));
#86108=CARTESIAN_POINT('Ctrl Pts',(-4.39037723602816,36.7894800611825,-1.21573330540808));
#86109=CARTESIAN_POINT('Ctrl Pts',(-3.94157828551533,36.250481844326,3.58627827351927));
#86110=CARTESIAN_POINT('Ctrl Pts',(-3.64237898517345,34.5353419369983,6.31390046791915));
#86111=CARTESIAN_POINT('Ctrl Pts',(-3.49277933500251,33.4246212024587,7.42462120245876));
#86112=CARTESIAN_POINT('Ctrl Pts',(-7.33674609398104,18.5753787975412,-7.42462120245874));
#86113=CARTESIAN_POINT('Ctrl Pts',(-7.1871464438101,19.6860995320808,-8.53534193699833));
#86114=CARTESIAN_POINT('Ctrl Pts',(-6.88794714346822,22.4134803337522,-10.2487508662659));
#86115=CARTESIAN_POINT('Ctrl Pts',(-6.43914819295539,27.2162249558894,-10.7922239637205));
#86116=CARTESIAN_POINT('Ctrl Pts',(-5.99034924244256,31.7766262509208,-9.19360309786621));
#86117=CARTESIAN_POINT('Ctrl Pts',(-5.54155029192973,35.1956822959411,-5.77827855619686));
#86118=CARTESIAN_POINT('Ctrl Pts',(-5.09275134141691,36.7894800611825,-1.21573330540808));
#86119=CARTESIAN_POINT('Ctrl Pts',(-4.64395239090408,36.250481844326,3.58627827351926));
#86120=CARTESIAN_POINT('Ctrl Pts',(-4.34475309056219,34.5353419369983,6.31390046791915));
#86121=CARTESIAN_POINT('Ctrl Pts',(-4.19515344039125,33.4246212024587,7.42462120245876));
#86122=CARTESIAN_POINT('',(-7.33674618680146,18.5753787975412,-7.42462120245874));
#86123=CARTESIAN_POINT('',(-4.19515344039125,33.4246212024587,7.42462120245876));
#86124=CARTESIAN_POINT('Ctrl Pts',(-10.3492814380484,21.7560621627659,-4.2405050092528));
#86125=CARTESIAN_POINT('Ctrl Pts',(-10.1995469203954,22.3910082818704,-4.87597392987967));
#86126=CARTESIAN_POINT('Ctrl Pts',(-9.90021275257146,23.9499413459023,-5.85575518849289));
#86127=CARTESIAN_POINT('Ctrl Pts',(-9.45127893457658,26.6949168047227,-6.16638084397979));
#86128=CARTESIAN_POINT('Ctrl Pts',(-9.00247998406375,29.3005993803806,-5.25296846874784));
#86129=CARTESIAN_POINT('Ctrl Pts',(-8.55368103355092,31.254154562729,-3.30155339634265));
#86130=CARTESIAN_POINT('Ctrl Pts',(-8.1048820830381,32.1647989151806,-0.694641763526773));
#86131=CARTESIAN_POINT('Ctrl Pts',(-7.65596869508309,31.8567582889011,2.04979291948575));
#86132=CARTESIAN_POINT('Ctrl Pts',(-7.35665495729904,30.8761069131734,3.60877902517104));
#86133=CARTESIAN_POINT('Ctrl Pts',(-7.20694086968591,30.2407651154807,4.24367792953755));
#86134=CARTESIAN_POINT('Ctrl Pts',(-10.7372588854526,20.6948332400255,-5.30087552725679));
#86135=CARTESIAN_POINT('Ctrl Pts',(-10.5875243677996,21.4885524636896,-6.09524828293874));
#86136=CARTESIAN_POINT('Ctrl Pts',(-10.2881901999756,23.4373085929068,-7.32003129451753));
#86137=CARTESIAN_POINT('Ctrl Pts',(-9.83925638198077,26.8686860351764,-7.70833125683706));
#86138=CARTESIAN_POINT('Ctrl Pts',(-9.39045743146795,30.1259393498091,-6.56651317252976));
#86139=CARTESIAN_POINT('Ctrl Pts',(-8.94165848095512,32.5679958583287,-4.12713192471575));
#86140=CARTESIAN_POINT('Ctrl Pts',(-8.49285953044229,33.7063537547143,-0.868342217838437));
#86141=CARTESIAN_POINT('Ctrl Pts',(-8.04394614248728,33.3212852278094,2.56235922352107));
#86142=CARTESIAN_POINT('Ctrl Pts',(-7.74463240470322,32.0954145197162,4.51118165786049));
#86143=CARTESIAN_POINT('Ctrl Pts',(-7.59491831709011,31.3012006750246,5.30484186038235));
#86144=CARTESIAN_POINT('Ctrl Pts',(-11.1252363328568,19.6336043172851,-6.36124604526076));
#86145=CARTESIAN_POINT('Ctrl Pts',(-10.9755018152038,20.5860966455086,-7.31452263599781));
#86146=CARTESIAN_POINT('Ctrl Pts',(-10.6761676473798,22.9246758399115,-8.78430740054218));
#86147=CARTESIAN_POINT('Ctrl Pts',(-10.2272338293849,27.0424552656302,-9.25028166969433));
#86148=CARTESIAN_POINT('Ctrl Pts',(-9.77843487887213,30.9512793192374,-7.88005787631169));
#86149=CARTESIAN_POINT('Ctrl Pts',(-9.3296359283593,33.8818371539285,-4.95271045308884));
#86150=CARTESIAN_POINT('Ctrl Pts',(-8.88083697784648,35.247908594248,-1.0420426721501));
#86151=CARTESIAN_POINT('Ctrl Pts',(-8.43192358989148,34.7858121667177,3.0749255275564));
#86152=CARTESIAN_POINT('Ctrl Pts',(-8.13260985210742,33.314722126259,5.41358429054993));
#86153=CARTESIAN_POINT('Ctrl Pts',(-7.98289576449429,32.3616362345684,6.36600579122716));
#86154=CARTESIAN_POINT('Ctrl Pts',(-11.513213780261,18.5723753945447,-7.42161656326474));
#86155=CARTESIAN_POINT('Ctrl Pts',(-11.363479262608,19.6836408273278,-8.53379698905687));
#86156=CARTESIAN_POINT('Ctrl Pts',(-11.0641450947841,22.4120430869161,-10.2485835065668));
#86157=CARTESIAN_POINT('Ctrl Pts',(-10.6152112767892,27.2162244960841,-10.7922320825516));
#86158=CARTESIAN_POINT('Ctrl Pts',(-10.1664123262763,31.7766192886659,-9.1936025800936));
#86159=CARTESIAN_POINT('Ctrl Pts',(-9.7176133757635,35.1956784495283,-5.77828898146194));
#86160=CARTESIAN_POINT('Ctrl Pts',(-9.26881442525067,36.7894634337816,-1.21574312646176));
#86161=CARTESIAN_POINT('Ctrl Pts',(-8.81990103729567,36.250339105626,3.58749183159172));
#86162=CARTESIAN_POINT('Ctrl Pts',(-8.52058729951161,34.5340297328017,6.31598692323937));
#86163=CARTESIAN_POINT('Ctrl Pts',(-8.37087321189849,33.4220717941122,7.42716972207196));
#86164=CARTESIAN_POINT('',(-11.5128092391113,18.5753787991571,-7.42462120084288));
#86165=CARTESIAN_POINT('',(-10.3231683825981,21.8280699909994,-4.17193000900062));
#86166=CARTESIAN_POINT('',(-8.37121652422502,33.4246212024587,7.42462120245876));
#86167=CARTESIAN_POINT('Ctrl Pts',(-11.5128091778148,18.5753787975412,-7.42462120245874));
#86168=CARTESIAN_POINT('Ctrl Pts',(-11.3632095276439,19.6860995320808,-8.53534193699833));
#86169=CARTESIAN_POINT('Ctrl Pts',(-11.213609451507,21.0497941968264,-9.39204359968316));
#86170=CARTESIAN_POINT('Ctrl Pts',(-11.0640099052434,22.5320974583249,-9.91097616832263));
#86171=CARTESIAN_POINT('Ctrl Pts',(-10.9144103589797,24.0144007198234,-10.4299087369621));
#86172=CARTESIAN_POINT('Ctrl Pts',(-10.7648108479412,25.6153125949017,-10.6110701604612));
#86173=CARTESIAN_POINT('Ctrl Pts',(-10.615211325617,27.1758334271763,-10.4352130137814));
#86174=CARTESIAN_POINT('Ctrl Pts',(-10.4656118032928,28.7363542594509,-10.2593558671016));
#86175=CARTESIAN_POINT('Ctrl Pts',(-10.3160122275825,30.2564852600915,-9.72648007747699));
#86176=CARTESIAN_POINT('Ctrl Pts',(-10.1664125253831,31.5863940042371,-8.8908232015921));
#86177=CARTESIAN_POINT('Ctrl Pts',(-10.0168128231837,32.9163027483828,-8.05516632570722));
#86178=CARTESIAN_POINT('Ctrl Pts',(-9.8672134190413,34.0559892681328,-6.91672982584028));
#86179=CARTESIAN_POINT('Ctrl Pts',(-9.7176136600352,34.8914626930057,-5.58708752460106));
#86180=CARTESIAN_POINT('Ctrl Pts',(-9.56801390102909,35.7269361178786,-4.25744522336183));
#86181=CARTESIAN_POINT('Ctrl Pts',(-9.41841355447926,36.2581960188536,-2.73659663848387));
#86182=CARTESIAN_POINT('Ctrl Pts',(-9.26881361325665,36.4339956847859,-1.17583727852711));
#86183=CARTESIAN_POINT('Ctrl Pts',(-9.11921367203404,36.6097953507183,0.384922081429656));
#86184=CARTESIAN_POINT('Ctrl Pts',(-8.96961418003796,36.4301347482737,1.98559219616138));
#86185=CARTESIAN_POINT('Ctrl Pts',(-8.8200147653941,35.9115214019404,3.46783679709374));
#86186=CARTESIAN_POINT('Ctrl Pts',(-8.67041535075024,35.3929080556071,4.9500813980261));
#86187=CARTESIAN_POINT('Ctrl Pts',(-8.52081617439596,34.5353419369983,6.31390046791915));
#86188=CARTESIAN_POINT('Ctrl Pts',(-8.37121652422502,33.4246212024587,7.42462120245876));
#86189=CARTESIAN_POINT('',(-7.18157563618792,30.1719300090006,4.17193000900064));
#86190=CARTESIAN_POINT('Ctrl Pts',(-13.6203358688322,18.5723770836602,-7.42161825376526));
#86191=CARTESIAN_POINT('Ctrl Pts',(-13.4706014270443,19.683642207911,-8.53379785982716));
#86192=CARTESIAN_POINT('Ctrl Pts',(-13.1712673350853,22.4120465854243,-10.2485818670356));
#86193=CARTESIAN_POINT('Ctrl Pts',(-12.7223335929554,27.2162241792528,-10.7922358496953));
#86194=CARTESIAN_POINT('Ctrl Pts',(-12.2735346424426,31.776615948509,-9.19360257337038));
#86195=CARTESIAN_POINT('Ctrl Pts',(-11.8247356919297,35.1956764374484,-5.77829392033626));
#86196=CARTESIAN_POINT('Ctrl Pts',(-11.3759367414169,36.7894556396735,-1.21574785540399));
#86197=CARTESIAN_POINT('Ctrl Pts',(-10.9270235257324,36.2503366865871,3.5874848749837));
#86198=CARTESIAN_POINT('Ctrl Pts',(-10.6277099602189,34.5340317104571,6.31598378636594));
#86199=CARTESIAN_POINT('Ctrl Pts',(-10.4779960448763,33.4220756325766,7.42716588627459));
#86200=CARTESIAN_POINT('Ctrl Pts',(-14.008313289448,19.6336056917925,-6.36124756744431));
#86201=CARTESIAN_POINT('Ctrl Pts',(-13.85857884766,20.5860977665283,-7.31452346654261));
#86202=CARTESIAN_POINT('Ctrl Pts',(-13.559244755701,22.9246788031716,-8.78430609636367));
#86203=CARTESIAN_POINT('Ctrl Pts',(-13.1103110135711,27.0424550060647,-9.2502850050701));
#86204=CARTESIAN_POINT('Ctrl Pts',(-12.6615120630582,30.9512765132955,-7.88005796124472));
#86205=CARTESIAN_POINT('Ctrl Pts',(-12.2127131125454,33.8818355200426,-4.95271474332016));
#86206=CARTESIAN_POINT('Ctrl Pts',(-11.7639141620326,35.2479020201693,-1.04204673743367));
#86207=CARTESIAN_POINT('Ctrl Pts',(-11.3150009463482,34.7858101944217,3.0749196002712));
#86208=CARTESIAN_POINT('Ctrl Pts',(-11.0156873808346,33.314723905544,5.41358166416799));
#86209=CARTESIAN_POINT('Ctrl Pts',(-10.8659734654919,32.3616395978279,6.3660025767426));
#86210=CARTESIAN_POINT('Ctrl Pts',(-14.3962907100637,20.6948342999247,-5.30087688112336));
#86211=CARTESIAN_POINT('Ctrl Pts',(-14.2465562682757,21.4885533251457,-6.09524907325806));
#86212=CARTESIAN_POINT('Ctrl Pts',(-13.9472221763167,23.4373110209188,-7.32003032569173));
#86213=CARTESIAN_POINT('Ctrl Pts',(-13.4982884341868,26.8686858328766,-7.70833416044494));
#86214=CARTESIAN_POINT('Ctrl Pts',(-13.049489483674,30.1259370780819,-6.56651334911906));
#86215=CARTESIAN_POINT('Ctrl Pts',(-12.6006905331612,32.5679946026368,-4.12713556630407));
#86216=CARTESIAN_POINT('Ctrl Pts',(-12.1518915826484,33.7063484006651,-0.868345619463353));
#86217=CARTESIAN_POINT('Ctrl Pts',(-11.7029783669638,33.3212837022564,2.5623543255587));
#86218=CARTESIAN_POINT('Ctrl Pts',(-11.4036648014502,32.0954161006308,4.51117954197003));
#86219=CARTESIAN_POINT('Ctrl Pts',(-11.2539508861077,31.3012035630792,5.30483926721062));
#86220=CARTESIAN_POINT('Ctrl Pts',(-14.7842681306794,21.7560629080571,-4.24050619480241));
#86221=CARTESIAN_POINT('Ctrl Pts',(-14.6345336888914,22.3910088837629,-4.87597467997351));
#86222=CARTESIAN_POINT('Ctrl Pts',(-14.3351995969325,23.9499432386661,-5.8557545550198));
#86223=CARTESIAN_POINT('Ctrl Pts',(-13.8862658548025,26.6949166596885,-6.16638331581976));
#86224=CARTESIAN_POINT('Ctrl Pts',(-13.4374669042897,29.3005976428683,-5.2529687369934));
#86225=CARTESIAN_POINT('Ctrl Pts',(-12.9886679537769,31.254153685231,-3.30155638928797));
#86226=CARTESIAN_POINT('Ctrl Pts',(-12.539869003264,32.164794781161,-0.69464450149303));
#86227=CARTESIAN_POINT('Ctrl Pts',(-12.0909557875795,31.856757210091,2.04978905084621));
#86228=CARTESIAN_POINT('Ctrl Pts',(-11.7916422220659,30.8761082957176,3.60877741977209));
#86229=CARTESIAN_POINT('Ctrl Pts',(-11.6419283067234,30.2407675283306,4.24367595767864));
#86230=CARTESIAN_POINT('',(-10.4783388403913,33.4246212024587,7.42462120245876));
#86231=CARTESIAN_POINT('',(-10.4783388403913,33.4246212024587,7.42462120245876));
#86232=CARTESIAN_POINT('',(-13.6199315418337,18.5753788014852,-7.42462119851477));
#86233=CARTESIAN_POINT('Ctrl Pts',(-13.619931493981,18.5753787975412,-7.42462120245874));
#86234=CARTESIAN_POINT('Ctrl Pts',(-13.4703318438101,19.6860995320808,-8.53534193699833));
#86235=CARTESIAN_POINT('Ctrl Pts',(-13.1711325434682,22.4134890318387,-10.248745098249));
#86236=CARTESIAN_POINT('Ctrl Pts',(-12.7223335929554,27.2162241792528,-10.7922358496953));
#86237=CARTESIAN_POINT('Ctrl Pts',(-12.2735346424426,31.776615948509,-9.19360257337038));
#86238=CARTESIAN_POINT('Ctrl Pts',(-11.8247356919297,35.1956764374484,-5.77829392033626));
#86239=CARTESIAN_POINT('Ctrl Pts',(-11.3759367414169,36.7894556396735,-1.21574785540399));
#86240=CARTESIAN_POINT('Ctrl Pts',(-10.9271377909041,36.2504739124864,3.58626227294545));
#86241=CARTESIAN_POINT('Ctrl Pts',(-10.6279384905622,34.5353419369983,6.31390046791915));
#86242=CARTESIAN_POINT('Ctrl Pts',(-10.4783388403913,33.4246212024587,7.42462120245876));
#86243=CARTESIAN_POINT('',(-13.6199315868015,18.5753787975412,-7.42462120245874));
#86244=CARTESIAN_POINT('Ctrl Pts',(-11.5128091778148,18.5753787975412,-7.42462120245874));
#86245=CARTESIAN_POINT('Ctrl Pts',(-11.3632095276439,19.6860995320808,-8.53534193699833));
#86246=CARTESIAN_POINT('Ctrl Pts',(-11.064010227302,22.4134890318387,-10.248745098249));
#86247=CARTESIAN_POINT('Ctrl Pts',(-10.6152112767892,27.2162241792528,-10.7922358496953));
#86248=CARTESIAN_POINT('Ctrl Pts',(-10.1664123262763,31.776615948509,-9.19360257337038));
#86249=CARTESIAN_POINT('Ctrl Pts',(-9.71761337576351,35.1956764374484,-5.77829392033626));
#86250=CARTESIAN_POINT('Ctrl Pts',(-9.26881442525068,36.7894556396735,-1.21574785540399));
#86251=CARTESIAN_POINT('Ctrl Pts',(-8.82001547473785,36.2504739124864,3.58626227294545));
#86252=CARTESIAN_POINT('Ctrl Pts',(-8.52081617439596,34.5353419369983,6.31390046791915));
#86253=CARTESIAN_POINT('Ctrl Pts',(-8.37121652422502,33.4246212024587,7.42462120245876));
#86254=CARTESIAN_POINT('Ctrl Pts',(-12.2151832832036,18.5753787975412,-7.42462120245874));
#86255=CARTESIAN_POINT('Ctrl Pts',(-12.0655836330326,19.6860995320808,-8.53534193699833));
#86256=CARTESIAN_POINT('Ctrl Pts',(-11.7663843326907,22.4134890318387,-10.248745098249));
#86257=CARTESIAN_POINT('Ctrl Pts',(-11.3175853821779,27.2162241792528,-10.7922358496953));
#86258=CARTESIAN_POINT('Ctrl Pts',(-10.8687864316651,31.7766159485089,-9.19360257337038));
#86259=CARTESIAN_POINT('Ctrl Pts',(-10.4199874811522,35.1956764374484,-5.77829392033625));
#86260=CARTESIAN_POINT('Ctrl Pts',(-9.97118853063942,36.7894556396735,-1.21574785540399));
#86261=CARTESIAN_POINT('Ctrl Pts',(-9.52238958012659,36.2504739124864,3.58626227294544));
#86262=CARTESIAN_POINT('Ctrl Pts',(-9.22319027978471,34.5353419369983,6.31390046791915));
#86263=CARTESIAN_POINT('Ctrl Pts',(-9.07359062961376,33.4246212024587,7.42462120245876));
#86264=CARTESIAN_POINT('Ctrl Pts',(-12.9175573885923,18.5753787975412,-7.42462120245874));
#86265=CARTESIAN_POINT('Ctrl Pts',(-12.7679577384214,19.6860995320808,-8.53534193699833));
#86266=CARTESIAN_POINT('Ctrl Pts',(-12.4687584380795,22.4134890318387,-10.248745098249));
#86267=CARTESIAN_POINT('Ctrl Pts',(-12.0199594875667,27.2162241792528,-10.7922358496953));
#86268=CARTESIAN_POINT('Ctrl Pts',(-11.5711605370538,31.776615948509,-9.19360257337038));
#86269=CARTESIAN_POINT('Ctrl Pts',(-11.122361586541,35.1956764374484,-5.77829392033626));
#86270=CARTESIAN_POINT('Ctrl Pts',(-10.6735626360282,36.7894556396735,-1.21574785540399));
#86271=CARTESIAN_POINT('Ctrl Pts',(-10.2247636855153,36.2504739124864,3.58626227294545));
#86272=CARTESIAN_POINT('Ctrl Pts',(-9.92556438517345,34.5353419369983,6.31390046791915));
#86273=CARTESIAN_POINT('Ctrl Pts',(-9.77596473500251,33.4246212024587,7.42462120245876));
#86274=CARTESIAN_POINT('Ctrl Pts',(-13.619931493981,18.5753787975412,-7.42462120245874));
#86275=CARTESIAN_POINT('Ctrl Pts',(-13.4703318438101,19.6860995320808,-8.53534193699833));
#86276=CARTESIAN_POINT('Ctrl Pts',(-13.1711325434682,22.4134890318387,-10.248745098249));
#86277=CARTESIAN_POINT('Ctrl Pts',(-12.7223335929554,27.2162241792528,-10.7922358496953));
#86278=CARTESIAN_POINT('Ctrl Pts',(-12.2735346424426,31.776615948509,-9.19360257337038));
#86279=CARTESIAN_POINT('Ctrl Pts',(-11.8247356919297,35.1956764374484,-5.77829392033626));
#86280=CARTESIAN_POINT('Ctrl Pts',(-11.3759367414169,36.7894556396735,-1.21574785540399));
#86281=CARTESIAN_POINT('Ctrl Pts',(-10.9271377909041,36.2504739124864,3.58626227294545));
#86282=CARTESIAN_POINT('Ctrl Pts',(-10.6279384905622,34.5353419369983,6.31390046791915));
#86283=CARTESIAN_POINT('Ctrl Pts',(-10.4783388403913,33.4246212024587,7.42462120245876));
#86284=CARTESIAN_POINT('',(-13.6199315868015,18.5753787975412,-7.42462120245874));
#86285=CARTESIAN_POINT('',(-10.4783388403913,33.4246212024587,7.42462120245876));
#86286=CARTESIAN_POINT('Ctrl Pts',(-17.341,36.2781643676599,2.14693670874701));
#86287=CARTESIAN_POINT('Ctrl Pts',(-17.1478414134638,35.8634651076156,4.13225241019146));
#86288=CARTESIAN_POINT('Ctrl Pts',(-16.9546828269275,34.8587505394928,5.99049186542473));
#86289=CARTESIAN_POINT('Ctrl Pts',(-16.7615242403913,33.4246212024587,7.42462120245876));
#86290=CARTESIAN_POINT('Ctrl Pts',(-17.5341585865363,35.5470552038234,1.99422022691288));
#86291=CARTESIAN_POINT('Ctrl Pts',(-17.341,35.1618544435509,3.83831591566697));
#86292=CARTESIAN_POINT('Ctrl Pts',(-17.1478414134638,34.2286075034518,5.56437458007748));
#86293=CARTESIAN_POINT('Ctrl Pts',(-16.9546828269275,32.8964910417647,6.89649104176468));
#86294=CARTESIAN_POINT('Ctrl Pts',(-17.7273171730725,34.8159460399869,1.84150374507876));
#86295=CARTESIAN_POINT('Ctrl Pts',(-17.5341585865363,34.4602437794863,3.54437942114248));
#86296=CARTESIAN_POINT('Ctrl Pts',(-17.341,33.5984644674109,5.13825729473024));
#86297=CARTESIAN_POINT('Ctrl Pts',(-17.1478414134638,32.3683608810706,6.3683608810706));
#86298=CARTESIAN_POINT('Ctrl Pts',(-17.9204757596088,34.0848368761504,1.68878726324463));
#86299=CARTESIAN_POINT('Ctrl Pts',(-17.7273171730725,33.7586331154217,3.250442926618));
#86300=CARTESIAN_POINT('Ctrl Pts',(-17.5341585865363,32.96832143137,4.71214000938299));
#86301=CARTESIAN_POINT('Ctrl Pts',(-17.341,31.8402307203765,5.84023072037652));
#86302=CARTESIAN_POINT('',(-16.7615242403913,33.4246212024587,7.42462120245876));
#86303=CARTESIAN_POINT('Ctrl Pts',(14.6516813050447,33.4616240069009,7.39654333888314));
#86304=CARTESIAN_POINT('Ctrl Pts',(14.8027409813318,32.3443801052069,8.52379090131628));
#86305=CARTESIAN_POINT('Ctrl Pts',(15.1034003077898,29.6043323150422,10.2532339919884));
#86306=CARTESIAN_POINT('Ctrl Pts',(15.5536592844188,24.7830334023154,10.7988321378608));
#86307=CARTESIAN_POINT('Ctrl Pts',(16.0024582349316,20.2198596429615,9.19921822804673));
#86308=CARTESIAN_POINT('Ctrl Pts',(16.4512571854445,16.7987093355857,5.78182911764146));
#86309=CARTESIAN_POINT('Ctrl Pts',(16.9000561359573,15.2039632259476,1.21649604870047));
#86310=CARTESIAN_POINT('Ctrl Pts',(17.3489898284458,15.7434301636902,-3.58988937742563));
#86311=CARTESIAN_POINT('Ctrl Pts',(17.6483238707635,17.4609906653758,-6.32021516100136));
#86312=CARTESIAN_POINT('Ctrl Pts',(17.7980582629102,18.573847497101,-7.43215861796121));
#86313=CARTESIAN_POINT('Ctrl Pts',(14.2631510305718,32.3946700237951,6.33889538324544));
#86314=CARTESIAN_POINT('Ctrl Pts',(14.4142107068588,31.4371832781721,7.30495534421649));
#86315=CARTESIAN_POINT('Ctrl Pts',(14.7148700333168,29.0889409315559,8.78710157398526));
#86316=CARTESIAN_POINT('Ctrl Pts',(15.1651290099459,24.9570501254182,9.25468344426202));
#86317=CARTESIAN_POINT('Ctrl Pts',(15.6139279604586,21.0463745907998,7.88380183601246));
#86318=CARTESIAN_POINT('Ctrl Pts',(16.0627269109714,18.1144220698418,4.9550726902204));
#86319=CARTESIAN_POINT('Ctrl Pts',(16.5115258614844,16.7477122043441,1.04254661042898));
#86320=CARTESIAN_POINT('Ctrl Pts',(16.9604595539729,17.2100395813897,-3.07656322126833));
#86321=CARTESIAN_POINT('Ctrl Pts',(17.2597935962906,18.6820023396344,-5.41647373234195));
#86322=CARTESIAN_POINT('Ctrl Pts',(17.4095279884373,19.6357293320462,-6.36941795544942));
#86323=CARTESIAN_POINT('Ctrl Pts',(13.8746207560988,31.3277160406894,5.28124742760773));
#86324=CARTESIAN_POINT('Ctrl Pts',(14.0256804323859,30.5299864511372,6.08611978711668));
#86325=CARTESIAN_POINT('Ctrl Pts',(14.3263397588439,28.5735495480696,7.32096915598215));
#86326=CARTESIAN_POINT('Ctrl Pts',(14.7765987354728,25.131066848521,7.71053475066323));
#86327=CARTESIAN_POINT('Ctrl Pts',(15.2253976859856,21.8728895386381,6.56838544397819));
#86328=CARTESIAN_POINT('Ctrl Pts',(15.6741966364985,19.430134804098,4.12831626279934));
#86329=CARTESIAN_POINT('Ctrl Pts',(16.1229955870113,18.2914611827405,0.868597172157502));
#86330=CARTESIAN_POINT('Ctrl Pts',(16.5719292794999,18.6766489990893,-2.56323706511104));
#86331=CARTESIAN_POINT('Ctrl Pts',(16.8712633218176,19.9030140138931,-4.51273230368253));
#86332=CARTESIAN_POINT('Ctrl Pts',(17.0209977139643,20.6976111669914,-5.30667729293762));
#86333=CARTESIAN_POINT('Ctrl Pts',(13.4860904816258,30.2607620575836,4.22359947197002));
#86334=CARTESIAN_POINT('Ctrl Pts',(13.637150157913,29.6227896241023,4.86728423001688));
#86335=CARTESIAN_POINT('Ctrl Pts',(13.937809484371,28.0581581645833,5.85483673797904));
#86336=CARTESIAN_POINT('Ctrl Pts',(14.3880684609999,25.3050835716238,6.16638605706443));
#86337=CARTESIAN_POINT('Ctrl Pts',(14.8368674115127,22.6994044864765,5.25296905194393));
#86338=CARTESIAN_POINT('Ctrl Pts',(15.2856663620255,20.7458475383541,3.30155983537828));
#86339=CARTESIAN_POINT('Ctrl Pts',(15.7344653125384,19.835210161137,0.694647733886021));
#86340=CARTESIAN_POINT('Ctrl Pts',(16.183399005027,20.1432584167887,-2.04991090895374));
#86341=CARTESIAN_POINT('Ctrl Pts',(16.4827330473447,21.1240256881518,-3.60899087502311));
#86342=CARTESIAN_POINT('Ctrl Pts',(16.6324674394913,21.7594930019366,-4.24393663042583));
#86343=CARTESIAN_POINT('Ctrl Pts',(11.6418674365106,30.243937729078,4.2405051874113));
#86344=CARTESIAN_POINT('Ctrl Pts',(11.7916019429138,29.6089916310296,4.87597404391556));
#86345=CARTESIAN_POINT('Ctrl Pts',(12.0909360994881,28.0500582137326,5.85575499156165));
#86346=CARTESIAN_POINT('Ctrl Pts',(12.5398699062332,25.3050832312864,6.16638143414342));
#86347=CARTESIAN_POINT('Ctrl Pts',(12.9886688567461,22.6994010669056,5.25296850297539));
#86348=CARTESIAN_POINT('Ctrl Pts',(13.4374678072589,20.7458456743692,3.30155412730027));
#86349=CARTESIAN_POINT('Ctrl Pts',(13.8862667577717,19.8352021475569,0.694642440642844));
#86350=CARTESIAN_POINT('Ctrl Pts',(14.335200564517,20.1432560444607,-2.04991703657224));
#86351=CARTESIAN_POINT('Ctrl Pts',(14.6345347210911,21.124026847436,-3.6089917582658));
#86352=CARTESIAN_POINT('Ctrl Pts',(14.7842692274945,21.7594948113833,-4.24393772890585));
#86353=CARTESIAN_POINT('Ctrl Pts',(11.2538899933664,31.3051666043796,5.3008757295882));
#86354=CARTESIAN_POINT('Ctrl Pts',(11.4036244997697,30.511447410088,6.09524840205956));
#86355=CARTESIAN_POINT('Ctrl Pts',(11.7029586563439,28.5626908467601,7.3200310202034));
#86356=CARTESIAN_POINT('Ctrl Pts',(12.1518924630891,25.1313140131761,7.70833196494418));
#86357=CARTESIAN_POINT('Ctrl Pts',(12.6006914136019,21.874061225185,6.56651319007401));
#86358=CARTESIAN_POINT('Ctrl Pts',(13.0494903641148,19.4320044633055,4.12713282258986));
#86359=CARTESIAN_POINT('Ctrl Pts',(13.4982893146276,18.2936476033927,0.868343060934551));
#86360=CARTESIAN_POINT('Ctrl Pts',(13.9472231213727,18.6787327178621,-2.5625143671782));
#86361=CARTESIAN_POINT('Ctrl Pts',(14.246557277947,19.9047527121812,-4.51144756914065));
#86362=CARTESIAN_POINT('Ctrl Pts',(14.3962917843502,20.699124268905,-5.30516660416449));
#86363=CARTESIAN_POINT('Ctrl Pts',(10.8659125502221,32.3663954796812,6.3612462717651));
#86364=CARTESIAN_POINT('Ctrl Pts',(11.0156470566255,31.4139031891465,7.31452276020357));
#86365=CARTESIAN_POINT('Ctrl Pts',(11.3149812131996,29.0753234797877,8.78430704884515));
#86366=CARTESIAN_POINT('Ctrl Pts',(11.7639150199449,24.957544795066,9.25028249574495));
#86367=CARTESIAN_POINT('Ctrl Pts',(12.2127139704577,21.0487213834643,7.88005787717263));
#86368=CARTESIAN_POINT('Ctrl Pts',(12.6615129209705,18.1181632522417,4.95271151787947));
#86369=CARTESIAN_POINT('Ctrl Pts',(13.1103118714834,16.7520930592284,1.04204368122625));
#86370=CARTESIAN_POINT('Ctrl Pts',(13.5592456782285,17.2142093912634,-3.07511169778416));
#86371=CARTESIAN_POINT('Ctrl Pts',(13.8585798348028,18.6854785769265,-5.4139033800155));
#86372=CARTESIAN_POINT('Ctrl Pts',(14.008314341206,19.6387537264267,-6.36639547942313));
#86373=CARTESIAN_POINT('Ctrl Pts',(10.477935107078,33.4276243549829,7.421616813942));
#86374=CARTESIAN_POINT('Ctrl Pts',(10.6276696134812,32.316358968205,8.53379711834758));
#86375=CARTESIAN_POINT('Ctrl Pts',(10.9270037700554,29.5879561128153,10.2485830774869));
#86376=CARTESIAN_POINT('Ctrl Pts',(11.3759375768006,24.7837755769558,10.7922330265457));
#86377=CARTESIAN_POINT('Ctrl Pts',(11.8247365273135,20.2233815417436,9.19360256427124));
#86378=CARTESIAN_POINT('Ctrl Pts',(12.2735354778263,16.804322041178,5.77829021316907));
#86379=CARTESIAN_POINT('Ctrl Pts',(12.7223344283391,15.2105385150642,1.21574430151796));
#86380=CARTESIAN_POINT('Ctrl Pts',(13.1712682350843,15.7496860646647,-3.58770902839013));
#86381=CARTESIAN_POINT('Ctrl Pts',(13.4706023916585,17.4662044416717,-6.31635919089035));
#86382=CARTESIAN_POINT('Ctrl Pts',(13.6203368980619,18.5783831839484,-7.42762435468178));
#86383=CARTESIAN_POINT('Ctrl Pts',(10.478339675775,33.4246212024587,7.42462120245875));
#86384=CARTESIAN_POINT('Ctrl Pts',(10.6279393259459,32.3139004679191,8.53534193699834));
#86385=CARTESIAN_POINT('Ctrl Pts',(10.9271386262878,29.5865129742571,10.2487463857135));
#86386=CARTESIAN_POINT('Ctrl Pts',(11.3759375768006,24.7837755769558,10.7922330265457));
#86387=CARTESIAN_POINT('Ctrl Pts',(11.8247365273135,20.2233815417436,9.19360256427124));
#86388=CARTESIAN_POINT('Ctrl Pts',(12.2735354778263,16.804322041178,5.77829021316907));
#86389=CARTESIAN_POINT('Ctrl Pts',(12.7223344283391,15.2105385150642,1.21574430151797));
#86390=CARTESIAN_POINT('Ctrl Pts',(13.1711333788519,15.7495241089239,-3.58626610827894));
#86391=CARTESIAN_POINT('Ctrl Pts',(13.4703326791938,17.4646580630017,-6.31390046791915));
#86392=CARTESIAN_POINT('Ctrl Pts',(13.6199323293648,18.5753787975412,-7.42462120245874));
#86393=CARTESIAN_POINT('Ctrl Pts',(8.37081273969933,33.4276247350626,7.42161643355506));
#86394=CARTESIAN_POINT('Ctrl Pts',(8.52054726317341,32.3163592768284,8.53379692106831));
#86395=CARTESIAN_POINT('Ctrl Pts',(8.81988143681844,29.5879591503046,10.2485849356456));
#86396=CARTESIAN_POINT('Ctrl Pts',(9.2688152606344,24.7837753005194,10.7922291011963));
#86397=CARTESIAN_POINT('Ctrl Pts',(9.71761421114723,20.2233781174552,9.19360269140817));
#86398=CARTESIAN_POINT('Ctrl Pts',(10.1664131616601,16.8043200601272,5.77828511785067));
#86399=CARTESIAN_POINT('Ctrl Pts',(10.6152121121729,15.2105304314665,1.21573946002376));
#86400=CARTESIAN_POINT('Ctrl Pts',(11.0641459359888,15.7496834327425,-3.58771450934957));
#86401=CARTESIAN_POINT('Ctrl Pts',(11.3634801096339,17.4662046398477,-6.31635949733812));
#86402=CARTESIAN_POINT('Ctrl Pts',(11.5132146331079,18.5783835643338,-7.42762473476445));
#86403=CARTESIAN_POINT('Ctrl Pts',(7.98283529009083,32.3663957877751,6.36124592805898));
#86404=CARTESIAN_POINT('Ctrl Pts',(8.13256981356493,31.4139034386388,7.31452257079588));
#86405=CARTESIAN_POINT('Ctrl Pts',(8.43190398720995,29.0753260747516,8.7843086171207));
#86406=CARTESIAN_POINT('Ctrl Pts',(8.88083781102592,24.957544561021,9.25027910554244));
#86407=CARTESIAN_POINT('Ctrl Pts',(9.32963676153874,21.0487184621757,7.88005796425917));
#86408=CARTESIAN_POINT('Ctrl Pts',(9.77843571205157,18.118161576126,4.95270713680419));
#86409=CARTESIAN_POINT('Ctrl Pts',(10.2272346625643,16.752086156267,1.04203952857104));
#86410=CARTESIAN_POINT('Ctrl Pts',(10.6761684863804,17.2142071597807,-3.07511638710569));
#86411=CARTESIAN_POINT('Ctrl Pts',(10.9755026600254,18.6854787671028,-5.41390362764302));
#86412=CARTESIAN_POINT('Ctrl Pts',(11.1252371834995,19.6387540701316,-6.36639578751951));
#86413=CARTESIAN_POINT('Ctrl Pts',(7.59485784048235,31.3051668404876,5.3008754225629));
#86414=CARTESIAN_POINT('Ctrl Pts',(7.74459236395643,30.5114476004492,6.09524822052343));
#86415=CARTESIAN_POINT('Ctrl Pts',(8.04392653760145,28.5626929991986,7.32003229859578));
#86416=CARTESIAN_POINT('Ctrl Pts',(8.49286036141743,25.1313138215225,7.70832910988854));
#86417=CARTESIAN_POINT('Ctrl Pts',(8.94165931193025,21.8740588068962,6.56651323711017));
#86418=CARTESIAN_POINT('Ctrl Pts',(9.39045826244308,19.4320030921246,4.1271291557577));
#86419=CARTESIAN_POINT('Ctrl Pts',(9.83925721295591,18.2936418810676,0.868339597118319));
#86420=CARTESIAN_POINT('Ctrl Pts',(10.2881910367718,18.6787308868189,-2.56251826486181));
#86421=CARTESIAN_POINT('Ctrl Pts',(10.5875252104169,19.9047528943578,-4.51144775794791));
#86422=CARTESIAN_POINT('Ctrl Pts',(10.737259733891,20.6991245759293,-5.30516684027456));
#86423=CARTESIAN_POINT('Ctrl Pts',(7.20688039087386,30.2439378932,4.24050491706681));
#86424=CARTESIAN_POINT('Ctrl Pts',(7.35661491434794,29.6089917622597,4.87597387025098));
#86425=CARTESIAN_POINT('Ctrl Pts',(7.65594908799297,28.0500599236457,5.85575598007085));
#86426=CARTESIAN_POINT('Ctrl Pts',(8.10488291180894,25.3050830820241,6.16637911423465));
#86427=CARTESIAN_POINT('Ctrl Pts',(8.55368186232177,22.6993991516167,5.25296850996117));
#86428=CARTESIAN_POINT('Ctrl Pts',(9.0024808128346,20.7458446081234,3.30155117471121));
#86429=CARTESIAN_POINT('Ctrl Pts',(9.45127976334742,19.8351976058681,0.694639665665589));
#86430=CARTESIAN_POINT('Ctrl Pts',(9.9002135871634,20.143254613857,-2.04992014261793));
#86431=CARTESIAN_POINT('Ctrl Pts',(10.1995477608084,21.124027021613,-3.6089918882528));
#86432=CARTESIAN_POINT('Ctrl Pts',(10.3492822842825,21.759495081727,-4.24393789302962));
#86433=CARTESIAN_POINT('Ctrl Pts',(8.37121735960875,33.4246212024587,7.42462120245875));
#86434=CARTESIAN_POINT('Ctrl Pts',(8.52081700977969,32.3139004679191,8.53534193699834));
#86435=CARTESIAN_POINT('Ctrl Pts',(8.82001631012158,29.5865129742571,10.2487463857135));
#86436=CARTESIAN_POINT('Ctrl Pts',(9.2688152606344,24.7837755769558,10.7922330265457));
#86437=CARTESIAN_POINT('Ctrl Pts',(9.71761421114723,20.2233815417436,9.19360256427124));
#86438=CARTESIAN_POINT('Ctrl Pts',(10.1664131616601,16.804322041178,5.77829021316907));
#86439=CARTESIAN_POINT('Ctrl Pts',(10.6152121121729,15.2105385150642,1.21574430151797));
#86440=CARTESIAN_POINT('Ctrl Pts',(11.0640110626857,15.7495241089239,-3.58626610827894));
#86441=CARTESIAN_POINT('Ctrl Pts',(11.3632103630276,17.4646580630017,-6.31390046791915));
#86442=CARTESIAN_POINT('Ctrl Pts',(11.5128100131985,18.5753787975412,-7.42462120245874));
#86443=CARTESIAN_POINT('Ctrl Pts',(10.478339675775,33.4246212024587,7.42462120245875));
#86444=CARTESIAN_POINT('Ctrl Pts',(10.6279393259459,32.3139004679191,8.53534193699834));
#86445=CARTESIAN_POINT('Ctrl Pts',(10.9271386262878,29.5865129742571,10.2487463857135));
#86446=CARTESIAN_POINT('Ctrl Pts',(11.3759375768006,24.7837755769558,10.7922330265457));
#86447=CARTESIAN_POINT('Ctrl Pts',(11.8247365273135,20.2233815417436,9.19360256427124));
#86448=CARTESIAN_POINT('Ctrl Pts',(12.2735354778263,16.804322041178,5.77829021316907));
#86449=CARTESIAN_POINT('Ctrl Pts',(12.7223344283391,15.2105385150642,1.21574430151797));
#86450=CARTESIAN_POINT('Ctrl Pts',(13.1711333788519,15.7495241089239,-3.58626610827894));
#86451=CARTESIAN_POINT('Ctrl Pts',(13.4703326791938,17.4646580630017,-6.31390046791915));
#86452=CARTESIAN_POINT('Ctrl Pts',(13.6199323293648,18.5753787975412,-7.42462120245874));
#86453=CARTESIAN_POINT('Ctrl Pts',(9.77596557038624,33.4246212024587,7.42462120245875));
#86454=CARTESIAN_POINT('Ctrl Pts',(9.92556522055718,32.3139004679191,8.53534193699834));
#86455=CARTESIAN_POINT('Ctrl Pts',(10.2247645208991,29.5865129742571,10.2487463857135));
#86456=CARTESIAN_POINT('Ctrl Pts',(10.6735634714119,24.7837755769558,10.7922330265457));
#86457=CARTESIAN_POINT('Ctrl Pts',(11.1223624219247,20.2233815417436,9.19360256427124));
#86458=CARTESIAN_POINT('Ctrl Pts',(11.5711613724375,16.804322041178,5.77829021316907));
#86459=CARTESIAN_POINT('Ctrl Pts',(12.0199603229504,15.2105385150642,1.21574430151797));
#86460=CARTESIAN_POINT('Ctrl Pts',(12.4687592734632,15.7495241089239,-3.58626610827895));
#86461=CARTESIAN_POINT('Ctrl Pts',(12.7679585738051,17.4646580630017,-6.31390046791915));
#86462=CARTESIAN_POINT('Ctrl Pts',(12.917558223976,18.5753787975412,-7.42462120245874));
#86463=CARTESIAN_POINT('Ctrl Pts',(9.07359146499749,33.4246212024587,7.42462120245875));
#86464=CARTESIAN_POINT('Ctrl Pts',(9.22319111516843,32.3139004679191,8.53534193699834));
#86465=CARTESIAN_POINT('Ctrl Pts',(9.52239041551032,29.5865129742571,10.2487463857135));
#86466=CARTESIAN_POINT('Ctrl Pts',(9.97118936602315,24.7837755769558,10.7922330265457));
#86467=CARTESIAN_POINT('Ctrl Pts',(10.419988316536,20.2233815417436,9.19360256427124));
#86468=CARTESIAN_POINT('Ctrl Pts',(10.8687872670488,16.804322041178,5.77829021316907));
#86469=CARTESIAN_POINT('Ctrl Pts',(11.3175862175616,15.2105385150642,1.21574430151797));
#86470=CARTESIAN_POINT('Ctrl Pts',(11.7663851680745,15.7495241089239,-3.58626610827894));
#86471=CARTESIAN_POINT('Ctrl Pts',(12.0655844684163,17.4646580630017,-6.31390046791915));
#86472=CARTESIAN_POINT('Ctrl Pts',(12.2151841185873,18.5753787975412,-7.42462120245874));
#86473=CARTESIAN_POINT('Ctrl Pts',(8.37121735960875,33.4246212024587,7.42462120245875));
#86474=CARTESIAN_POINT('Ctrl Pts',(8.52081700977969,32.3139004679191,8.53534193699834));
#86475=CARTESIAN_POINT('Ctrl Pts',(8.82001631012158,29.5865129742571,10.2487463857135));
#86476=CARTESIAN_POINT('Ctrl Pts',(9.2688152606344,24.7837755769558,10.7922330265457));
#86477=CARTESIAN_POINT('Ctrl Pts',(9.71761421114723,20.2233815417436,9.19360256427124));
#86478=CARTESIAN_POINT('Ctrl Pts',(10.1664131616601,16.804322041178,5.77829021316907));
#86479=CARTESIAN_POINT('Ctrl Pts',(10.6152121121729,15.2105385150642,1.21574430151797));
#86480=CARTESIAN_POINT('Ctrl Pts',(11.0640110626857,15.7495241089239,-3.58626610827894));
#86481=CARTESIAN_POINT('Ctrl Pts',(11.3632103630276,17.4646580630017,-6.31390046791915));
#86482=CARTESIAN_POINT('Ctrl Pts',(11.5128100131985,18.5753787975412,-7.42462120245874));
#86483=CARTESIAN_POINT('Ctrl Pts',(5.35868174475438,30.2439392339151,4.24050270859203));
#86484=CARTESIAN_POINT('Ctrl Pts',(5.5084164076812,29.6089928430004,4.87597245720932));
#86485=CARTESIAN_POINT('Ctrl Pts',(5.80775072077896,28.0500642248033,5.85575779538567));
#86486=CARTESIAN_POINT('Ctrl Pts',(6.25668468404766,25.3050829459043,6.16637363300279));
#86487=CARTESIAN_POINT('Ctrl Pts',(6.70548363456049,22.6993954022398,5.25296843898345));
#86488=CARTESIAN_POINT('Ctrl Pts',(7.15428258507332,20.7458430022638,3.30154467940644));
#86489=CARTESIAN_POINT('Ctrl Pts',(7.60308153558614,19.8351883604915,0.694633848166402));
#86490=CARTESIAN_POINT('Ctrl Pts',(8.05201549885485,20.143252256087,-2.04992724536302));
#86491=CARTESIAN_POINT('Ctrl Pts',(8.35134981195262,21.1240284360682,-3.60899296659441));
#86492=CARTESIAN_POINT('Ctrl Pts',(8.50108447487943,21.7594972901986,-4.24393923374772));
#86493=CARTESIAN_POINT('Ctrl Pts',(4.9707042423387,31.3051687692584,5.30087291443731));
#86494=CARTESIAN_POINT('Ctrl Pts',(5.12043890526552,30.5114491664153,6.09524674458825));
#86495=CARTESIAN_POINT('Ctrl Pts',(5.41977321836328,28.5626984980101,7.3200349166553));
#86496=CARTESIAN_POINT('Ctrl Pts',(5.86870718163198,25.1313136099707,7.70832262534694));
#86497=CARTESIAN_POINT('Ctrl Pts',(6.31750613214481,21.8740539233512,6.56651346128887));
#86498=CARTESIAN_POINT('Ctrl Pts',(6.76630508265764,19.4320007717319,4.12712123291654));
#86499=CARTESIAN_POINT('Ctrl Pts',(7.21510403317047,18.2936299565934,0.868332366286644));
#86500=CARTESIAN_POINT('Ctrl Pts',(7.66403799643918,18.6787275906001,-2.56252726581087));
#86501=CARTESIAN_POINT('Ctrl Pts',(7.96337230953693,19.9047543720601,-4.51144932091485));
#86502=CARTESIAN_POINT('Ctrl Pts',(8.11310697246375,20.6991270840509,-5.30516876904924));
#86503=CARTESIAN_POINT('Ctrl Pts',(4.58272673992303,32.3663983046018,6.36124312028259));
#86504=CARTESIAN_POINT('Ctrl Pts',(4.73246140284985,31.4139054898301,7.31452103196719));
#86505=CARTESIAN_POINT('Ctrl Pts',(5.0317957159476,29.075332771217,8.78431203792494));
#86506=CARTESIAN_POINT('Ctrl Pts',(5.48072967921631,24.9575442740369,9.25027161769109));
#86507=CARTESIAN_POINT('Ctrl Pts',(5.92952862972914,21.0487124444625,7.88005848359428));
#86508=CARTESIAN_POINT('Ctrl Pts',(6.37832758024196,18.1181585412,4.95269778642663));
#86509=CARTESIAN_POINT('Ctrl Pts',(6.82712653075479,16.7520715526952,1.04203088440688));
#86510=CARTESIAN_POINT('Ctrl Pts',(7.2760604940235,17.2142029251132,-3.07512728625873));
#86511=CARTESIAN_POINT('Ctrl Pts',(7.57539480712126,18.6854803080521,-5.41390567523528));
#86512=CARTESIAN_POINT('Ctrl Pts',(7.72512947004808,19.6387568779032,-6.36639830435076));
#86513=CARTESIAN_POINT('Ctrl Pts',(4.19474923750735,33.4276278399451,7.42161332612787));
#86514=CARTESIAN_POINT('Ctrl Pts',(4.34448390043417,32.3163618132449,8.53379531934612));
#86515=CARTESIAN_POINT('Ctrl Pts',(4.64381821353193,29.5879670444238,10.2485891591946));
#86516=CARTESIAN_POINT('Ctrl Pts',(5.09275217680063,24.7837749381033,10.7922206100352));
#86517=CARTESIAN_POINT('Ctrl Pts',(5.54155112731346,20.2233709655738,9.19360350589969));
#86518=CARTESIAN_POINT('Ctrl Pts',(5.99035007782629,16.8043163106681,5.77827433993672));
#86519=CARTESIAN_POINT('Ctrl Pts',(6.43914902833912,15.210513148797,1.21572940252713));
#86520=CARTESIAN_POINT('Ctrl Pts',(6.88808299160782,15.7496782596263,-3.58772730670658));
#86521=CARTESIAN_POINT('Ctrl Pts',(7.18741730470558,17.4662062440441,-6.31636202955571));
#86522=CARTESIAN_POINT('Ctrl Pts',(7.3371519676324,18.5783866717555,-7.42762783965229));
#86523=CARTESIAN_POINT('Ctrl Pts',(4.19515427577498,33.4246212024587,7.42462120245875));
#86524=CARTESIAN_POINT('Ctrl Pts',(4.34475392594592,32.3139004679191,8.53534193699834));
#86525=CARTESIAN_POINT('Ctrl Pts',(4.64395322628781,29.5865222278826,10.2487526513479));
#86526=CARTESIAN_POINT('Ctrl Pts',(5.09275217680063,24.7837749381033,10.7922206100352));
#86527=CARTESIAN_POINT('Ctrl Pts',(5.54155112731346,20.2233709655738,9.1936035058997));
#86528=CARTESIAN_POINT('Ctrl Pts',(5.99035007782629,16.8043163106681,5.77827433993673));
#86529=CARTESIAN_POINT('Ctrl Pts',(6.43914902833912,15.2105131487971,1.21572940252714));
#86530=CARTESIAN_POINT('Ctrl Pts',(6.88794797885194,15.7495161106836,-3.58628271132928));
#86531=CARTESIAN_POINT('Ctrl Pts',(7.18714727919383,17.4646580630017,-6.31390046791915));
#86532=CARTESIAN_POINT('Ctrl Pts',(7.33674692936478,18.5753787975412,-7.42462120245874));
#86533=CARTESIAN_POINT('Ctrl Pts',(2.08762722947389,33.4276297757683,7.4216136630885));
#86534=CARTESIAN_POINT('Ctrl Pts',(2.23736192827097,32.3163634308879,8.53379621253978));
#86535=CARTESIAN_POINT('Ctrl Pts',(2.53669627723901,29.5879716382176,10.2485932995738));
#86536=CARTESIAN_POINT('Ctrl Pts',(2.98563027637797,24.7837746802806,10.7922175564503));
#86537=CARTESIAN_POINT('Ctrl Pts',(3.4344292268908,20.2233662640449,9.19360566949466));
#86538=CARTESIAN_POINT('Ctrl Pts',(3.88322817740363,16.8043131390746,5.77826939950743));
#86539=CARTESIAN_POINT('Ctrl Pts',(4.33202712791647,15.210502056439,1.21572426912528));
#86540=CARTESIAN_POINT('Ctrl Pts',(4.78096112705543,15.7496740126713,-3.58773440230587));
#86541=CARTESIAN_POINT('Ctrl Pts',(5.08029547602347,17.4662053513639,-6.31636364499683));
#86542=CARTESIAN_POINT('Ctrl Pts',(5.23003017482055,18.5783863347936,-7.42762977547842));
#86543=CARTESIAN_POINT('Ctrl Pts',(1.69964957489386,32.3663997101047,6.36124315556745));
#86544=CARTESIAN_POINT('Ctrl Pts',(1.84938427369095,31.4139066605754,7.31452150601911));
#86545=CARTESIAN_POINT('Ctrl Pts',(2.14871862265898,29.0753365860982,8.78431523663789));
#86546=CARTESIAN_POINT('Ctrl Pts',(2.59765262179796,24.9575440945989,9.25026863171355));
#86547=CARTESIAN_POINT('Ctrl Pts',(3.04645157231079,21.0487086120065,7.88006002399772));
#86548=CARTESIAN_POINT('Ctrl Pts',(3.49525052282361,18.1181561368879,4.9526933544726));
#86549=CARTESIAN_POINT('Ctrl Pts',(3.94404947333644,16.7520624137522,1.04202644291405));
#86550=CARTESIAN_POINT('Ctrl Pts',(4.39298347247541,17.2141996351108,-3.07513324550561));
#86551=CARTESIAN_POINT('Ctrl Pts',(4.69231782144344,18.6854798344402,-5.41390684409329));
#86552=CARTESIAN_POINT('Ctrl Pts',(4.84205252024054,19.6387568426173,-6.36639970985615));
#86553=CARTESIAN_POINT('Ctrl Pts',(1.31167192031384,31.305169644441,5.3008726480464));
#86554=CARTESIAN_POINT('Ctrl Pts',(1.46140661911093,30.5114498902629,6.09524679949844));
#86555=CARTESIAN_POINT('Ctrl Pts',(1.76074096807896,28.5627015339787,7.32003717370199));
#86556=CARTESIAN_POINT('Ctrl Pts',(2.20967496721793,25.131313508917,7.70831970697682));
#86557=CARTESIAN_POINT('Ctrl Pts',(2.65847391773076,21.8740509599683,6.56651437850079));
#86558=CARTESIAN_POINT('Ctrl Pts',(3.10727286824359,19.4319991347012,4.12711730943777));
#86559=CARTESIAN_POINT('Ctrl Pts',(3.55607181875642,18.2936227710653,0.868328616702831));
#86560=CARTESIAN_POINT('Ctrl Pts',(4.00500581789539,18.6787252575502,-2.56253208870534));
#86561=CARTESIAN_POINT('Ctrl Pts',(4.30434016686343,19.9047543175165,-4.51145004318976));
#86562=CARTESIAN_POINT('Ctrl Pts',(4.45407486566051,20.6991273504409,-5.30516964423389));
#86563=CARTESIAN_POINT('Ctrl Pts',(0.923694265733817,30.2439395787773,4.24050214052534));
#86564=CARTESIAN_POINT('Ctrl Pts',(1.0734289645309,29.6089931199504,4.87597209297777));
#86565=CARTESIAN_POINT('Ctrl Pts',(1.37276331349894,28.0500664818591,5.85575911076608));
#86566=CARTESIAN_POINT('Ctrl Pts',(1.82169731263791,25.3050829232352,6.16637078224008));
#86567=CARTESIAN_POINT('Ctrl Pts',(2.27049626315073,22.6993933079299,5.25296873300386));
#86568=CARTESIAN_POINT('Ctrl Pts',(2.71929521366356,20.7458421325144,3.30154126440294));
#86569=CARTESIAN_POINT('Ctrl Pts',(3.16809416417639,19.8351831283785,0.6946307904916));
#86570=CARTESIAN_POINT('Ctrl Pts',(3.61702816331537,20.1432508799898,-2.04993093190507));
#86571=CARTESIAN_POINT('Ctrl Pts',(3.9163625122834,21.124028800593,-3.60899324228622));
#86572=CARTESIAN_POINT('Ctrl Pts',(4.06609721108049,21.7594978582645,-4.24393957861161));
#86573=CARTESIAN_POINT('Ctrl Pts',(2.08803195960875,33.4246212024587,7.42462120245875));
#86574=CARTESIAN_POINT('Ctrl Pts',(2.21811206017887,32.4588257297478,8.39041667516967));
#86575=CARTESIAN_POINT('Ctrl Pts',(2.34820226714463,31.3016837902186,9.16424028291839));
#86576=CARTESIAN_POINT('Ctrl Pts',(2.62717564621961,28.599440768817,10.2935716436691));
#86577=CARTESIAN_POINT('Ctrl Pts',(2.7581160852288,27.2104401715646,10.4952143025461));
#86578=CARTESIAN_POINT('Ctrl Pts',(3.03683618944768,24.2839074379147,10.508047074406));
#86579=CARTESIAN_POINT('Ctrl Pts',(3.17097575048872,22.9060540952459,10.0808266335396));
#86580=CARTESIAN_POINT('Ctrl Pts',(3.39661765884711,20.7150047323306,9.17859210179939));
#86581=CARTESIAN_POINT('Ctrl Pts',(3.52698910038257,19.5549163112383,8.40289350048828));
#86582=CARTESIAN_POINT('Ctrl Pts',(3.7906967856087,17.5961616011175,6.44526974701291));
#86583=CARTESIAN_POINT('Ctrl Pts',(3.92095407984858,16.821005659722,5.28667072334715));
#86584=CARTESIAN_POINT('Ctrl Pts',(4.15157399185054,15.9001504081183,3.04686683603555));
#86585=CARTESIAN_POINT('Ctrl Pts',(4.28507227448216,15.4945892500986,1.67135405527008));
#86586=CARTESIAN_POINT('Ctrl Pts',(4.55616748351115,15.5046184878954,-1.17517952963084));
#86587=CARTESIAN_POINT('Ctrl Pts',(4.68788920228244,15.6947442723585,-2.57456045049193));
#86588=CARTESIAN_POINT('Ctrl Pts',(4.96973339204285,16.8367707735847,-5.30408588680115));
#86589=CARTESIAN_POINT('Ctrl Pts',(5.09968523508116,17.6106281357367,-6.45987054065413));
#86590=CARTESIAN_POINT('Ctrl Pts',(5.22962461319854,18.5753787975412,-7.42462120245874));
#86591=CARTESIAN_POINT('Ctrl Pts',(4.19515427577498,33.4246212024587,7.42462120245875));
#86592=CARTESIAN_POINT('Ctrl Pts',(4.34475392594592,32.3139004679191,8.53534193699834));
#86593=CARTESIAN_POINT('Ctrl Pts',(4.64395322628781,29.5865222278826,10.2487526513479));
#86594=CARTESIAN_POINT('Ctrl Pts',(5.09275217680063,24.7837749381033,10.7922206100352));
#86595=CARTESIAN_POINT('Ctrl Pts',(5.54155112731346,20.2233709655738,9.1936035058997));
#86596=CARTESIAN_POINT('Ctrl Pts',(5.99035007782629,16.8043163106681,5.77827433993673));
#86597=CARTESIAN_POINT('Ctrl Pts',(6.43914902833912,15.2105131487971,1.21572940252714));
#86598=CARTESIAN_POINT('Ctrl Pts',(6.88794797885194,15.7495161106836,-3.58628271132928));
#86599=CARTESIAN_POINT('Ctrl Pts',(7.18714727919383,17.4646580630017,-6.31390046791915));
#86600=CARTESIAN_POINT('Ctrl Pts',(7.33674692936478,18.5753787975412,-7.42462120245874));
#86601=CARTESIAN_POINT('Ctrl Pts',(3.49277937258034,33.4246212024587,7.42462120245875));
#86602=CARTESIAN_POINT('Ctrl Pts',(3.64237902275128,32.3139004679191,8.53534193699834));
#86603=CARTESIAN_POINT('Ctrl Pts',(3.94157832309317,29.5865222278826,10.2487526513479));
#86604=CARTESIAN_POINT('Ctrl Pts',(4.39037727360599,24.7837749381034,10.7922206100352));
#86605=CARTESIAN_POINT('Ctrl Pts',(4.83917622411882,20.2233709655738,9.1936035058997));
#86606=CARTESIAN_POINT('Ctrl Pts',(5.28797517463164,16.8043163106681,5.77827433993673));
#86607=CARTESIAN_POINT('Ctrl Pts',(5.73677412514448,15.2105131487971,1.21572940252714));
#86608=CARTESIAN_POINT('Ctrl Pts',(6.1855730756573,15.7495161106836,-3.58628271132928));
#86609=CARTESIAN_POINT('Ctrl Pts',(6.48477237599919,17.4646580630017,-6.31390046791915));
#86610=CARTESIAN_POINT('Ctrl Pts',(6.63437202617013,18.5753787975412,-7.42462120245874));
#86611=CARTESIAN_POINT('Ctrl Pts',(2.79040446938569,33.4246212024587,7.42462120245875));
#86612=CARTESIAN_POINT('Ctrl Pts',(2.94000411955663,32.3139004679191,8.53534193699834));
#86613=CARTESIAN_POINT('Ctrl Pts',(3.23920341989852,29.5865222278826,10.2487526513479));
#86614=CARTESIAN_POINT('Ctrl Pts',(3.68800237041135,24.7837749381034,10.7922206100352));
#86615=CARTESIAN_POINT('Ctrl Pts',(4.13680132092417,20.2233709655738,9.1936035058997));
#86616=CARTESIAN_POINT('Ctrl Pts',(4.585600271437,16.8043163106681,5.77827433993673));
#86617=CARTESIAN_POINT('Ctrl Pts',(5.03439922194982,15.2105131487971,1.21572940252714));
#86618=CARTESIAN_POINT('Ctrl Pts',(5.48319817246266,15.7495161106836,-3.58628271132928));
#86619=CARTESIAN_POINT('Ctrl Pts',(5.78239747280454,17.4646580630017,-6.31390046791915));
#86620=CARTESIAN_POINT('Ctrl Pts',(5.93199712297549,18.5753787975412,-7.42462120245874));
#86621=CARTESIAN_POINT('Ctrl Pts',(2.08802956619104,33.4246212024587,7.42462120245875));
#86622=CARTESIAN_POINT('Ctrl Pts',(2.23762921636198,32.3139004679191,8.53534193699834));
#86623=CARTESIAN_POINT('Ctrl Pts',(2.53682851670387,29.5865222278826,10.2487526513479));
#86624=CARTESIAN_POINT('Ctrl Pts',(2.98562746721669,24.7837749381033,10.7922206100352));
#86625=CARTESIAN_POINT('Ctrl Pts',(3.43442641772952,20.2233709655738,9.1936035058997));
#86626=CARTESIAN_POINT('Ctrl Pts',(3.88322536824235,16.8043163106681,5.77827433993673));
#86627=CARTESIAN_POINT('Ctrl Pts',(4.33202431875518,15.2105131487971,1.21572940252714));
#86628=CARTESIAN_POINT('Ctrl Pts',(4.780823269268,15.7495161106836,-3.58628271132928));
#86629=CARTESIAN_POINT('Ctrl Pts',(5.08002256960989,17.4646580630017,-6.31390046791915));
#86630=CARTESIAN_POINT('Ctrl Pts',(5.22962221978083,18.5753787975412,-7.42462120245874));
#86631=CARTESIAN_POINT('Ctrl Pts',(-0.924503774144115,30.2439398471762,
4.24050169840643));
#86632=CARTESIAN_POINT('Ctrl Pts',(-0.774769047429751,29.6089933369654,
4.87597181055117));
#86633=CARTESIAN_POINT('Ctrl Pts',(-0.475434670544444,28.0500666106541,
5.85575897175579));
#86634=CARTESIAN_POINT('Ctrl Pts',(-0.0265006434881952,25.3050829374398,
6.16637065619458));
#86635=CARTESIAN_POINT('Ctrl Pts',(0.422298307024632,22.6993933753954,5.25296862563014));
#86636=CARTESIAN_POINT('Ctrl Pts',(0.871097257537459,20.7458422399122,3.30154119691606));
#86637=CARTESIAN_POINT('Ctrl Pts',(1.31989620805029,19.8351832543889,0.694630776291687));
#86638=CARTESIAN_POINT('Ctrl Pts',(1.76883023510653,20.143251018862,-2.04993106067715));
#86639=CARTESIAN_POINT('Ctrl Pts',(2.06816461199185,21.1240290832044,-3.60899345932658));
#86640=CARTESIAN_POINT('Ctrl Pts',(2.21789933870621,21.759498300383,-4.24393984701044));
#86641=CARTESIAN_POINT('Ctrl Pts',(-1.31248159385698,31.3051704533329,5.30087256836657));
#86642=CARTESIAN_POINT('Ctrl Pts',(-1.16274686714261,30.5114505640989,6.09524699032489));
#86643=CARTESIAN_POINT('Ctrl Pts',(-0.863412490257304,28.5627019236485,
7.32003765309461));
#86644=CARTESIAN_POINT('Ctrl Pts',(-0.414478463201055,25.131313449161,7.70832023722244));
#86645=CARTESIAN_POINT('Ctrl Pts',(0.0343204873117733,21.8740506761476,
6.56651483020448));
#86646=CARTESIAN_POINT('Ctrl Pts',(0.4831194378246,19.431998682895,4.12711759333603));
#86647=CARTESIAN_POINT('Ctrl Pts',(0.931918388337429,18.2936222409493,0.868328676432679));
#86648=CARTESIAN_POINT('Ctrl Pts',(1.38085241539368,18.6787247778748,-2.56253247833145));
#86649=CARTESIAN_POINT('Ctrl Pts',(1.68018679227898,19.9047541269212,-4.51145071705737));
#86650=CARTESIAN_POINT('Ctrl Pts',(1.82992151899334,20.6991274301201,-5.30517045312578));
#86651=CARTESIAN_POINT('Ctrl Pts',(-1.70045941356983,32.3664010594897,6.36124343832671));
#86652=CARTESIAN_POINT('Ctrl Pts',(-1.55072468685547,31.4139077912323,7.31452217009862));
#86653=CARTESIAN_POINT('Ctrl Pts',(-1.25139030997017,29.0753372366429,8.78431633443344));
#86654=CARTESIAN_POINT('Ctrl Pts',(-0.802456282913913,24.9575439608823,
9.25026981825031));
#86655=CARTESIAN_POINT('Ctrl Pts',(-0.353657332401086,21.0487079768996,
7.88006103477882));
#86656=CARTESIAN_POINT('Ctrl Pts',(0.0951416181117414,18.1181551258777,
4.952693989756));
#86657=CARTESIAN_POINT('Ctrl Pts',(0.54394056862457,16.7520612275095,1.04202657657367));
#86658=CARTESIAN_POINT('Ctrl Pts',(0.992874595680818,17.2141985368875,-3.07513389598574));
#86659=CARTESIAN_POINT('Ctrl Pts',(1.29220897256613,18.6854791706381,-5.41390797478815));
#86660=CARTESIAN_POINT('Ctrl Pts',(1.44194369928049,19.6387565598573,-6.36640105924111));
#86661=CARTESIAN_POINT('Ctrl Pts',(-2.08843723328269,33.4276316656465,7.42161430828685));
#86662=CARTESIAN_POINT('Ctrl Pts',(-1.93870250656833,32.3163650183657,8.53379734987234));
#86663=CARTESIAN_POINT('Ctrl Pts',(-1.63936812968302,29.5879725496372,10.2485950157723));
#86664=CARTESIAN_POINT('Ctrl Pts',(-1.19043410262678,24.7837744726036,10.7922193992782));
#86665=CARTESIAN_POINT('Ctrl Pts',(-0.741635152113946,20.2233652776518,
9.19360723935315));
#86666=CARTESIAN_POINT('Ctrl Pts',(-0.292836201601118,16.8043115688604,
5.77827038617597));
#86667=CARTESIAN_POINT('Ctrl Pts',(0.15596274891171,15.2105002140697,1.21572447671466));
#86668=CARTESIAN_POINT('Ctrl Pts',(0.604896775967959,15.7496722959002,-3.58773531364002));
#86669=CARTESIAN_POINT('Ctrl Pts',(0.904231152853266,17.4662042143551,-6.31636523251894));
#86670=CARTESIAN_POINT('Ctrl Pts',(1.05396587956763,18.5783856895944,-7.42763166535646));
#86671=CARTESIAN_POINT('Ctrl Pts',(-2.08803112422502,33.4246212024587,7.42462120245876));
#86672=CARTESIAN_POINT('Ctrl Pts',(-1.95795102164571,32.4588257148303,8.39041669008711));
#86673=CARTESIAN_POINT('Ctrl Pts',(-1.82785996694436,31.3016837529055,9.1642403083045));
#86674=CARTESIAN_POINT('Ctrl Pts',(-1.54888671495528,28.599441070071,10.2935715065643));
#86675=CARTESIAN_POINT('Ctrl Pts',(-1.4179475651678,27.210440567088,10.4952142905163));
#86676=CARTESIAN_POINT('Ctrl Pts',(-1.13922861879923,24.2839070763066,10.5080470913502));
#86677=CARTESIAN_POINT('Ctrl Pts',(-1.00508812325812,22.9060536884507,10.0808264748192));
#86678=CARTESIAN_POINT('Ctrl Pts',(-0.779445153014362,20.7150047089726,
9.17859207969596));
#86679=CARTESIAN_POINT('Ctrl Pts',(-0.649074110348536,19.5549162993542,
8.40289349433808));
#86680=CARTESIAN_POINT('Ctrl Pts',(-0.385366820301348,17.5961615542775,
6.44526969447176));
#86681=CARTESIAN_POINT('Ctrl Pts',(-0.255108777477327,16.8210056428898,
5.28667067345667));
#86682=CARTESIAN_POINT('Ctrl Pts',(-0.0244870309043847,15.9001505892118,
3.04686728314339));
#86683=CARTESIAN_POINT('Ctrl Pts',(0.109012683773514,15.4945892040144,1.67135439212475));
#86684=CARTESIAN_POINT('Ctrl Pts',(0.380107909868443,15.5046185193411,-1.17517988914753));
#86685=CARTESIAN_POINT('Ctrl Pts',(0.511829062496731,15.6947443684176,-2.57456079137983));
#86686=CARTESIAN_POINT('Ctrl Pts',(0.793671459716859,16.8367708937086,-5.30408607867575));
#86687=CARTESIAN_POINT('Ctrl Pts',(0.923622163707121,17.6106282282455,-6.45987063316294));
#86688=CARTESIAN_POINT('Ctrl Pts',(1.05356152936475,18.5753787975412,-7.42462120245874));
#86689=CARTESIAN_POINT('Ctrl Pts',(-4.1955583921502,33.427627197915,7.42161396868715));
#86690=CARTESIAN_POINT('Ctrl Pts',(-4.04582375805961,32.3163612875677,8.53379564973379));
#86691=CARTESIAN_POINT('Ctrl Pts',(-3.74648947379807,29.5879667358391,10.2485891941145));
#86692=CARTESIAN_POINT('Ctrl Pts',(-3.2975555393656,24.7837749381033,10.7922206100334));
#86693=CARTESIAN_POINT('Ctrl Pts',(-2.84875658885277,20.2233709655724,9.19360350589995));
#86694=CARTESIAN_POINT('Ctrl Pts',(-2.39995763833994,16.8043163106674,5.77827433993448));
#86695=CARTESIAN_POINT('Ctrl Pts',(-1.95115868782712,15.2105131487934,1.21572940252506));
#86696=CARTESIAN_POINT('Ctrl Pts',(-1.50222475339464,15.7496782249932,-3.58772699817009));
#86697=CARTESIAN_POINT('Ctrl Pts',(-1.2028904691331,17.4662059133223,-6.31636150383227));
#86698=CARTESIAN_POINT('Ctrl Pts',(-1.05315583504251,18.5783860291971,-7.42762719762228));
#86699=CARTESIAN_POINT('Ctrl Pts',(-4.58353588364633,32.3663977841704,6.36124370087948));
#86700=CARTESIAN_POINT('Ctrl Pts',(-4.43380124955573,31.4139050646589,7.31452134946661));
#86701=CARTESIAN_POINT('Ctrl Pts',(-4.1344669652942,29.0753325211495,8.78431210906737));
#86702=CARTESIAN_POINT('Ctrl Pts',(-3.68553303086173,24.9575442691462,9.25027166108737));
#86703=CARTESIAN_POINT('Ctrl Pts',(-3.23673408034891,21.0487124212322,7.88005852056394));
#86704=CARTESIAN_POINT('Ctrl Pts',(-2.78793512983608,18.1181585042216,4.95269780966037));
#86705=CARTESIAN_POINT('Ctrl Pts',(-2.33913617932325,16.7520715093053,1.04203088929382));
#86706=CARTESIAN_POINT('Ctrl Pts',(-1.89020224489077,17.2142028542096,-3.0751270362317));
#86707=CARTESIAN_POINT('Ctrl Pts',(-1.59086796062924,18.6854799902663,-5.41390525002451));
#86708=CARTESIAN_POINT('Ctrl Pts',(-1.44113332653865,19.6387562973071,-6.36639778391949));
#86709=CARTESIAN_POINT('Ctrl Pts',(-4.97151337514246,31.3051683704258,5.30087343307181));
#86710=CARTESIAN_POINT('Ctrl Pts',(-4.82177874105187,30.5114488417502,6.09524704919943));
#86711=CARTESIAN_POINT('Ctrl Pts',(-4.52244445679034,28.56269830646,7.32003502402029));
#86712=CARTESIAN_POINT('Ctrl Pts',(-4.07351052235786,25.1313136001892,7.70832271214129));
#86713=CARTESIAN_POINT('Ctrl Pts',(-3.62471157184503,21.8740538768921,6.56651353522793));
#86714=CARTESIAN_POINT('Ctrl Pts',(-3.1759126213322,19.4320006977758,4.12712127938628));
#86715=CARTESIAN_POINT('Ctrl Pts',(-2.72711367081938,18.2936298698171,0.868332376062584));
#86716=CARTESIAN_POINT('Ctrl Pts',(-2.27817973638691,18.678727483426,-2.56252707429332));
#86717=CARTESIAN_POINT('Ctrl Pts',(-1.97884545212538,19.9047540672103,-4.51144899621676));
#86718=CARTESIAN_POINT('Ctrl Pts',(-1.82911081803478,20.699126565417,-5.30516837021671));
#86719=CARTESIAN_POINT('Ctrl Pts',(-5.3594908666386,30.2439389566812,4.24050316526413));
#86720=CARTESIAN_POINT('Ctrl Pts',(-5.209756232548,29.6089926188414,4.87597274893225));
#86721=CARTESIAN_POINT('Ctrl Pts',(-4.91042194828647,28.0500640917706,5.8557579389732));
#86722=CARTESIAN_POINT('Ctrl Pts',(-4.46148801385399,25.3050829312321,6.16637376319522));
#86723=CARTESIAN_POINT('Ctrl Pts',(-4.01268906334117,22.6993953325519,5.25296854989192));
#86724=CARTESIAN_POINT('Ctrl Pts',(-3.56389011282834,20.74584289133,3.30154474911218));
#86725=CARTESIAN_POINT('Ctrl Pts',(-3.11509116231551,19.835188230329,0.694633862831345));
#86726=CARTESIAN_POINT('Ctrl Pts',(-2.66615722788303,20.1432521126424,-2.04992711235493));
#86727=CARTESIAN_POINT('Ctrl Pts',(-2.3668229436215,21.1240281441544,-3.608992742409));
#86728=CARTESIAN_POINT('Ctrl Pts',(-2.21708830953092,21.759496833527,-4.24393895651391));
#86729=CARTESIAN_POINT('Ctrl Pts',(-4.19515344039125,33.4246212024587,7.42462120245875));
#86730=CARTESIAN_POINT('Ctrl Pts',(-4.04555379022031,32.3139004679191,8.53534193699834));
#86731=CARTESIAN_POINT('Ctrl Pts',(-3.74635448987842,29.586522227884,10.2487526513489));
#86732=CARTESIAN_POINT('Ctrl Pts',(-3.2975555393656,24.7837749381033,10.7922206100334));
#86733=CARTESIAN_POINT('Ctrl Pts',(-2.84875658885277,20.2233709655724,9.19360350589995));
#86734=CARTESIAN_POINT('Ctrl Pts',(-2.39995763833994,16.8043163106674,5.77827433993448));
#86735=CARTESIAN_POINT('Ctrl Pts',(-1.95115868782712,15.2105131487934,1.21572940252506));
#86736=CARTESIAN_POINT('Ctrl Pts',(-1.50235973731429,15.7495161106825,-3.58628271133166));
#86737=CARTESIAN_POINT('Ctrl Pts',(-1.2031604369724,17.4646580630017,-6.31390046791915));
#86738=CARTESIAN_POINT('Ctrl Pts',(-1.05356078680146,18.5753787975412,-7.42462120245874));
#86739=CARTESIAN_POINT('Ctrl Pts',(-2.08802985083253,33.4246212024587,7.42462120245875));
#86740=CARTESIAN_POINT('Ctrl Pts',(-1.93843020066159,32.3139004679191,8.53534193699834));
#86741=CARTESIAN_POINT('Ctrl Pts',(-1.6392309003197,29.586522227884,10.2487526513489));
#86742=CARTESIAN_POINT('Ctrl Pts',(-1.19043194980688,24.7837749381033,10.7922206100334));
#86743=CARTESIAN_POINT('Ctrl Pts',(-0.741632999294046,20.2233709655724,
9.19360350589995));
#86744=CARTESIAN_POINT('Ctrl Pts',(-0.292834048781219,16.8043163106674,
5.77827433993448));
#86745=CARTESIAN_POINT('Ctrl Pts',(0.155964901731608,15.2105131487934,1.21572940252506));
#86746=CARTESIAN_POINT('Ctrl Pts',(0.604763852244435,15.7495161106825,-3.58628271133166));
#86747=CARTESIAN_POINT('Ctrl Pts',(0.90396315258632,17.4646580630017,-6.31390046791915));
#86748=CARTESIAN_POINT('Ctrl Pts',(1.05356280275726,18.5753787975412,-7.42462120245874));
#86749=CARTESIAN_POINT('Ctrl Pts',(-2.79040438068543,33.4246212024587,7.42462120245875));
#86750=CARTESIAN_POINT('Ctrl Pts',(-2.64080473051449,32.3139004679191,8.53534193699834));
#86751=CARTESIAN_POINT('Ctrl Pts',(-2.34160543017261,29.586522227884,10.2487526513489));
#86752=CARTESIAN_POINT('Ctrl Pts',(-1.89280647965978,24.7837749381033,10.7922206100334));
#86753=CARTESIAN_POINT('Ctrl Pts',(-1.44400752914695,20.2233709655724,9.19360350589994));
#86754=CARTESIAN_POINT('Ctrl Pts',(-0.995208578634126,16.8043163106674,
5.77827433993448));
#86755=CARTESIAN_POINT('Ctrl Pts',(-0.5464096281213,15.2105131487934,1.21572940252506));
#86756=CARTESIAN_POINT('Ctrl Pts',(-0.0976106776084724,15.7495161106825,
-3.58628271133166));
#86757=CARTESIAN_POINT('Ctrl Pts',(0.201588622733412,17.4646580630017,-6.31390046791915));
#86758=CARTESIAN_POINT('Ctrl Pts',(0.351188272904354,18.5753787975412,-7.42462120245874));
#86759=CARTESIAN_POINT('Ctrl Pts',(-3.49277891053835,33.4246212024587,7.42462120245875));
#86760=CARTESIAN_POINT('Ctrl Pts',(-3.3431792603674,32.3139004679191,8.53534193699834));
#86761=CARTESIAN_POINT('Ctrl Pts',(-3.04397996002552,29.586522227884,10.2487526513489));
#86762=CARTESIAN_POINT('Ctrl Pts',(-2.59518100951269,24.7837749381033,10.7922206100334));
#86763=CARTESIAN_POINT('Ctrl Pts',(-2.14638205899987,20.2233709655724,9.19360350589995));
#86764=CARTESIAN_POINT('Ctrl Pts',(-1.69758310848704,16.8043163106674,5.77827433993448));
#86765=CARTESIAN_POINT('Ctrl Pts',(-1.24878415797421,15.2105131487934,1.21572940252507));
#86766=CARTESIAN_POINT('Ctrl Pts',(-0.79998520746138,15.7495161106825,-3.58628271133166));
#86767=CARTESIAN_POINT('Ctrl Pts',(-0.500785907119496,17.4646580630017,
-6.31390046791915));
#86768=CARTESIAN_POINT('Ctrl Pts',(-0.351186256948554,18.5753787975412,
-7.42462120245874));
#86769=CARTESIAN_POINT('Ctrl Pts',(-4.19515344039125,33.4246212024587,7.42462120245875));
#86770=CARTESIAN_POINT('Ctrl Pts',(-4.04555379022031,32.3139004679191,8.53534193699834));
#86771=CARTESIAN_POINT('Ctrl Pts',(-3.74635448987842,29.586522227884,10.2487526513489));
#86772=CARTESIAN_POINT('Ctrl Pts',(-3.2975555393656,24.7837749381033,10.7922206100334));
#86773=CARTESIAN_POINT('Ctrl Pts',(-2.84875658885277,20.2233709655724,9.19360350589995));
#86774=CARTESIAN_POINT('Ctrl Pts',(-2.39995763833994,16.8043163106674,5.77827433993448));
#86775=CARTESIAN_POINT('Ctrl Pts',(-1.95115868782712,15.2105131487934,1.21572940252506));
#86776=CARTESIAN_POINT('Ctrl Pts',(-1.50235973731429,15.7495161106825,-3.58628271133166));
#86777=CARTESIAN_POINT('Ctrl Pts',(-1.2031604369724,17.4646580630017,-6.31390046791915));
#86778=CARTESIAN_POINT('Ctrl Pts',(-1.05356078680146,18.5753787975412,-7.42462120245874));
#86779=CARTESIAN_POINT('Ctrl Pts',(-7.20768885204555,30.2439381858381,4.24050443502072));
#86780=CARTESIAN_POINT('Ctrl Pts',(-7.05795429813301,29.6089919988744,4.8759735623196));
#86781=CARTESIAN_POINT('Ctrl Pts',(-6.75862009404954,28.0500600640715,5.85575582850576));
#86782=CARTESIAN_POINT('Ctrl Pts',(-6.30968623979511,25.3050830975113,6.16637897680622));
#86783=CARTESIAN_POINT('Ctrl Pts',(-5.86088728928228,22.699399225175,5.2529683928905));
#86784=CARTESIAN_POINT('Ctrl Pts',(-5.41208833876945,20.7458447252201,3.30155110112974));
#86785=CARTESIAN_POINT('Ctrl Pts',(-4.96328938825663,19.8351977432586,0.694639650183325));
#86786=CARTESIAN_POINT('Ctrl Pts',(-4.51435553400221,20.14325476527,-2.04992028301914));
#86787=CARTESIAN_POINT('Ctrl Pts',(-4.21502132991872,21.1240273297457,-3.60899212489599));
#86788=CARTESIAN_POINT('Ctrl Pts',(-4.06528677600618,21.7594955637725,-4.24393818566755));
#86789=CARTESIAN_POINT('Ctrl Pts',(-7.5956663131803,31.3051672614807,5.30087487511165));
#86790=CARTESIAN_POINT('Ctrl Pts',(-7.44593175926777,30.5114479431546,6.09524789898784));
#86791=CARTESIAN_POINT('Ctrl Pts',(-7.14659755518428,28.5626932013935,7.32003218526599));
#86792=CARTESIAN_POINT('Ctrl Pts',(-6.69766370092986,25.1313138318473,7.70832901826905));
#86793=CARTESIAN_POINT('Ctrl Pts',(-6.24886475041704,21.8740588559346,6.56651315906309));
#86794=CARTESIAN_POINT('Ctrl Pts',(-5.80006579990421,19.4320031701889,4.1271291067027));
#86795=CARTESIAN_POINT('Ctrl Pts',(-5.35126684939138,18.2936419726602,0.868339586796149));
#86796=CARTESIAN_POINT('Ctrl Pts',(-4.90233299513695,18.6787309999456,-2.56251846702403));
#86797=CARTESIAN_POINT('Ctrl Pts',(-4.60299879105348,19.9047532161451,-4.51144810068888));
#86798=CARTESIAN_POINT('Ctrl Pts',(-4.45326423714094,20.6991251233798,-5.30516726126762));
#86799=CARTESIAN_POINT('Ctrl Pts',(-7.98364377431505,32.3663963371234,6.36124531520258));
#86800=CARTESIAN_POINT('Ctrl Pts',(-7.83390922040251,31.4139038874348,7.31452223565608));
#86801=CARTESIAN_POINT('Ctrl Pts',(-7.53457501631904,29.0753263387154,8.78430854202622));
#86802=CARTESIAN_POINT('Ctrl Pts',(-7.08564116206461,24.9575445661833,9.2502790597319));
#86803=CARTESIAN_POINT('Ctrl Pts',(-6.63684221155178,21.0487184866942,7.88005792523567));
#86804=CARTESIAN_POINT('Ctrl Pts',(-6.18804326103897,18.1181616151576,4.95270711227565));
#86805=CARTESIAN_POINT('Ctrl Pts',(-5.73924431052613,16.7520862020617,1.04203952340898));
#86806=CARTESIAN_POINT('Ctrl Pts',(-5.29031045627171,17.2142072346213,-3.07511665102894));
#86807=CARTESIAN_POINT('Ctrl Pts',(-4.99097625218822,18.6854791025447,-5.41390407648176));
#86808=CARTESIAN_POINT('Ctrl Pts',(-4.84124169827569,19.6387546829872,-6.36639633686769));
#86809=CARTESIAN_POINT('Ctrl Pts',(-8.37162123544981,33.4276254127661,7.42161575529352));
#86810=CARTESIAN_POINT('Ctrl Pts',(-8.22188668153727,32.3163598317151,8.53379657232431));
#86811=CARTESIAN_POINT('Ctrl Pts',(-7.92255247745379,29.5879594760374,10.2485848987865));
#86812=CARTESIAN_POINT('Ctrl Pts',(-7.47361862319936,24.7837753005193,10.7922291011947));
#86813=CARTESIAN_POINT('Ctrl Pts',(-7.02481967268654,20.2233781174538,9.19360269140826));
#86814=CARTESIAN_POINT('Ctrl Pts',(-6.57602072217371,16.8043200601264,5.7782851178486));
#86815=CARTESIAN_POINT('Ctrl Pts',(-6.12722177166088,15.2105304314633,1.2157394600218));
#86816=CARTESIAN_POINT('Ctrl Pts',(-5.67828791740646,15.749683469297,-3.58771483503384));
#86817=CARTESIAN_POINT('Ctrl Pts',(-5.37895371332298,17.4662049889442,-6.31636005227465));
#86818=CARTESIAN_POINT('Ctrl Pts',(-5.22921915941045,18.5783842425945,-7.42762541246777));
#86819=CARTESIAN_POINT('Ctrl Pts',(-8.37121652422502,33.4246212024587,7.42462120245875));
#86820=CARTESIAN_POINT('Ctrl Pts',(-8.22161687405408,32.3139004679191,8.53534193699834));
#86821=CARTESIAN_POINT('Ctrl Pts',(-8.07201676796994,30.9502068124086,9.39204424902068));
#86822=CARTESIAN_POINT('Ctrl Pts',(-7.92241722279933,29.4679036763263,9.91097645495401));
#86823=CARTESIAN_POINT('Ctrl Pts',(-7.77281767762872,27.985600540244,10.4299086608873));
#86824=CARTESIAN_POINT('Ctrl Pts',(-7.62321818610899,26.384687907658,10.6110686467821));
#86825=CARTESIAN_POINT('Ctrl Pts',(-7.47361866868718,24.8241663324414,10.43521127997));
#86826=CARTESIAN_POINT('Ctrl Pts',(-7.32401915126538,23.2636447572247,10.259353913158));
#86827=CARTESIAN_POINT('Ctrl Pts',(-7.17441957677565,21.7435129664056,9.72647916848619));
#86828=CARTESIAN_POINT('Ctrl Pts',(-7.02481986772503,20.4136040170806,8.8908221268261));
#86829=CARTESIAN_POINT('Ctrl Pts',(-6.87522015867441,19.0836950677556,8.05516508516602));
#86830=CARTESIAN_POINT('Ctrl Pts',(-6.72562077057793,17.9440089158971,6.91672732344894));
#86831=CARTESIAN_POINT('Ctrl Pts',(-6.57602101558995,17.108534919825,5.58708444540028));
#86832=CARTESIAN_POINT('Ctrl Pts',(-6.42642126060197,16.2730609237529,4.25744156735162));
#86833=CARTESIAN_POINT('Ctrl Pts',(-6.27682088159159,15.7417995729601,2.73659303696763));
#86834=CARTESIAN_POINT('Ctrl Pts',(-6.1272209307994,15.5659998279322,1.1758336557523));
#86835=CARTESIAN_POINT('Ctrl Pts',(-5.97762098000721,15.3902000829043,-0.384925725463033));
#86836=CARTESIAN_POINT('Ctrl Pts',(-5.82802150279226,15.5698619777324,-1.98559593691079));
#86837=CARTESIAN_POINT('Ctrl Pts',(-5.67842209597348,16.0884764653087,-3.46783962661608));
#86838=CARTESIAN_POINT('Ctrl Pts',(-5.52882268915469,16.6070909528849,-4.95008331632137));
#86839=CARTESIAN_POINT('Ctrl Pts',(-5.37922352080617,17.4646580630017,-6.31390046791915));
#86840=CARTESIAN_POINT('Ctrl Pts',(-5.22962387063524,18.5753787975412,-7.4246212024587));
#86841=CARTESIAN_POINT('Ctrl Pts',(-10.4787433156322,33.4276236613913,7.42161750810454));
#86842=CARTESIAN_POINT('Ctrl Pts',(-10.3290088403809,32.3163584003089,8.53379747526706));
#86843=CARTESIAN_POINT('Ctrl Pts',(-10.0296747149587,29.5879557794486,10.2485831152121));
#86844=CARTESIAN_POINT('Ctrl Pts',(-9.5807409393656,24.7837755769557,10.7922330265442));
#86845=CARTESIAN_POINT('Ctrl Pts',(-9.13194198885277,20.2233815417423,9.19360256427126));
#86846=CARTESIAN_POINT('Ctrl Pts',(-8.68314303833994,16.8043220411772,5.77829021316709));
#86847=CARTESIAN_POINT('Ctrl Pts',(-8.23434408782711,15.2105385150611,1.21574430151608));
#86848=CARTESIAN_POINT('Ctrl Pts',(-7.78541031223398,15.7496860272516,-3.58770869507484));
#86849=CARTESIAN_POINT('Ctrl Pts',(-7.4860761868118,17.4662040843916,-6.31635862294282));
#86850=CARTESIAN_POINT('Ctrl Pts',(-7.33634171156056,18.5783824897868,-7.42762366109035));
#86851=CARTESIAN_POINT('Ctrl Pts',(-10.8667207469799,32.3663949174539,6.36124689898917));
#86852=CARTESIAN_POINT('Ctrl Pts',(-10.7169862717286,31.4139027298284,7.31452310319999));
#86853=CARTESIAN_POINT('Ctrl Pts',(-10.4176521463065,29.0753232096377,8.78430712570177));
#86854=CARTESIAN_POINT('Ctrl Pts',(-9.96871837071332,24.9575447897825,9.25028254262678));
#86855=CARTESIAN_POINT('Ctrl Pts',(-9.5199194202005,21.0487213583686,7.88005791711107));
#86856=CARTESIAN_POINT('Ctrl Pts',(-9.07112046968767,18.1181632122936,4.95271154297956));
#86857=CARTESIAN_POINT('Ctrl Pts',(-8.62232151917484,16.7520930123547,1.04204368650602));
#86858=CARTESIAN_POINT('Ctrl Pts',(-8.17338774358171,17.2142093146667,-3.07511142767717));
#86859=CARTESIAN_POINT('Ctrl Pts',(-7.87405361815953,18.685478233621,-5.41390292065324));
#86860=CARTESIAN_POINT('Ctrl Pts',(-7.72431914290828,19.6387530992035,-6.36639491719599));
#86861=CARTESIAN_POINT('Ctrl Pts',(-11.2546981783276,31.3051661735166,5.30087628987379));
#86862=CARTESIAN_POINT('Ctrl Pts',(-11.1049637030764,30.5114470593478,6.0952487311329));
#86863=CARTESIAN_POINT('Ctrl Pts',(-10.8056295776542,28.5626906398269,7.32003113619143));
#86864=CARTESIAN_POINT('Ctrl Pts',(-10.3566958020611,25.1313140026092,7.70833205870936));
#86865=CARTESIAN_POINT('Ctrl Pts',(-9.90789685154823,21.874061174995,6.5665132699509));
#86866=CARTESIAN_POINT('Ctrl Pts',(-9.4590979010354,19.43200438341,4.12713287279204));
#86867=CARTESIAN_POINT('Ctrl Pts',(-9.01029895052258,18.2936475096483,0.868343071495974));
#86868=CARTESIAN_POINT('Ctrl Pts',(-8.56136517492943,18.6787326020819,-2.56251416027952));
#86869=CARTESIAN_POINT('Ctrl Pts',(-8.26203104950726,19.9047523828503,-4.51144721836367));
#86870=CARTESIAN_POINT('Ctrl Pts',(-8.11229657425601,20.6991237086201,-5.30516617330163));
#86871=CARTESIAN_POINT('Ctrl Pts',(-11.6426756096754,30.2439374295793,4.2405056807584));
#86872=CARTESIAN_POINT('Ctrl Pts',(-11.4929411344241,29.6089913888673,4.87597435906582));
#86873=CARTESIAN_POINT('Ctrl Pts',(-11.1936070090019,28.050058070016,5.85575514668108));
#86874=CARTESIAN_POINT('Ctrl Pts',(-10.7446732334088,25.3050832154359,6.16638157479195));
#86875=CARTESIAN_POINT('Ctrl Pts',(-10.295874282896,22.6994009916213,5.25296862279071));
#86876=CARTESIAN_POINT('Ctrl Pts',(-9.84707533238312,20.7458455545263,3.30155420260451));
#86877=CARTESIAN_POINT('Ctrl Pts',(-9.3982763818703,19.835202006942,0.694642456485917));
#86878=CARTESIAN_POINT('Ctrl Pts',(-8.94934260627717,20.143255889497,-2.04991689288185));
#86879=CARTESIAN_POINT('Ctrl Pts',(-8.65000848085499,21.1240265320798,-3.6089915160741));
#86880=CARTESIAN_POINT('Ctrl Pts',(-8.50027400560374,21.7594943180368,-4.24393742940726));
#86881=CARTESIAN_POINT('Ctrl Pts',(-10.4783388403913,33.4246212024587,7.42462120245875));
#86882=CARTESIAN_POINT('Ctrl Pts',(-10.3287391902203,32.3139004679191,8.53534193699834));
#86883=CARTESIAN_POINT('Ctrl Pts',(-10.0295398898784,29.5865129742582,10.2487463857142));
#86884=CARTESIAN_POINT('Ctrl Pts',(-9.58074093936559,24.7837755769557,10.7922330265442));
#86885=CARTESIAN_POINT('Ctrl Pts',(-9.13194198885277,20.2233815417423,9.19360256427126));
#86886=CARTESIAN_POINT('Ctrl Pts',(-8.68314303833994,16.8043220411772,5.77829021316709));
#86887=CARTESIAN_POINT('Ctrl Pts',(-8.23434408782711,15.2105385150611,1.21574430151608));
#86888=CARTESIAN_POINT('Ctrl Pts',(-7.78554513731429,15.7495241089229,-3.58626610828099));
#86889=CARTESIAN_POINT('Ctrl Pts',(-7.4863458369724,17.4646580630017,-6.31390046791915));
#86890=CARTESIAN_POINT('Ctrl Pts',(-7.33674618680146,18.5753787975412,-7.42462120245874));
#86891=CARTESIAN_POINT('Ctrl Pts',(-8.37121652422502,33.4246212024587,7.42462120245875));
#86892=CARTESIAN_POINT('Ctrl Pts',(-8.22161687405408,32.3139004679191,8.53534193699834));
#86893=CARTESIAN_POINT('Ctrl Pts',(-7.92241757371219,29.5865129742582,10.2487463857142));
#86894=CARTESIAN_POINT('Ctrl Pts',(-7.47361862319936,24.7837755769557,10.7922330265442));
#86895=CARTESIAN_POINT('Ctrl Pts',(-7.02481967268654,20.2233815417423,9.19360256427126));
#86896=CARTESIAN_POINT('Ctrl Pts',(-6.57602072217371,16.8043220411772,5.77829021316709));
#86897=CARTESIAN_POINT('Ctrl Pts',(-6.12722177166088,15.2105385150611,1.21574430151608));
#86898=CARTESIAN_POINT('Ctrl Pts',(-5.67842282114805,15.7495241089229,-3.58626610828099));
#86899=CARTESIAN_POINT('Ctrl Pts',(-5.37922352080617,17.4646580630017,-6.31390046791915));
#86900=CARTESIAN_POINT('Ctrl Pts',(-5.22962387063522,18.5753787975412,-7.42462120245874));
#86901=CARTESIAN_POINT('Ctrl Pts',(-9.07359062961376,33.4246212024587,7.42462120245875));
#86902=CARTESIAN_POINT('Ctrl Pts',(-8.92399097944282,32.3139004679191,8.53534193699834));
#86903=CARTESIAN_POINT('Ctrl Pts',(-8.62479167910094,29.5865129742582,10.2487463857142));
#86904=CARTESIAN_POINT('Ctrl Pts',(-8.17599272858811,24.7837755769557,10.7922330265442));
#86905=CARTESIAN_POINT('Ctrl Pts',(-7.72719377807528,20.2233815417423,9.19360256427126));
#86906=CARTESIAN_POINT('Ctrl Pts',(-7.27839482756245,16.8043220411772,5.77829021316709));
#86907=CARTESIAN_POINT('Ctrl Pts',(-6.82959587704963,15.2105385150611,1.21574430151608));
#86908=CARTESIAN_POINT('Ctrl Pts',(-6.3807969265368,15.7495241089229,-3.586266108281));
#86909=CARTESIAN_POINT('Ctrl Pts',(-6.08159762619491,17.4646580630017,-6.31390046791915));
#86910=CARTESIAN_POINT('Ctrl Pts',(-5.93199797602397,18.5753787975412,-7.42462120245874));
#86911=CARTESIAN_POINT('Ctrl Pts',(-9.77596473500251,33.4246212024587,7.42462120245875));
#86912=CARTESIAN_POINT('Ctrl Pts',(-9.62636508483157,32.3139004679191,8.53534193699834));
#86913=CARTESIAN_POINT('Ctrl Pts',(-9.32716578448968,29.5865129742582,10.2487463857142));
#86914=CARTESIAN_POINT('Ctrl Pts',(-8.87836683397685,24.7837755769557,10.7922330265442));
#86915=CARTESIAN_POINT('Ctrl Pts',(-8.42956788346403,20.2233815417423,9.19360256427127));
#86916=CARTESIAN_POINT('Ctrl Pts',(-7.98076893295119,16.8043220411772,5.77829021316709));
#86917=CARTESIAN_POINT('Ctrl Pts',(-7.53196998243837,15.2105385150611,1.21574430151608));
#86918=CARTESIAN_POINT('Ctrl Pts',(-7.08317103192554,15.7495241089229,-3.586266108281));
#86919=CARTESIAN_POINT('Ctrl Pts',(-6.78397173158366,17.4646580630017,-6.31390046791915));
#86920=CARTESIAN_POINT('Ctrl Pts',(-6.63437208141271,18.5753787975412,-7.42462120245874));
#86921=CARTESIAN_POINT('Ctrl Pts',(-10.4783388403913,33.4246212024587,7.42462120245875));
#86922=CARTESIAN_POINT('Ctrl Pts',(-10.3287391902203,32.3139004679191,8.53534193699834));
#86923=CARTESIAN_POINT('Ctrl Pts',(-10.0295398898784,29.5865129742582,10.2487463857142));
#86924=CARTESIAN_POINT('Ctrl Pts',(-9.58074093936559,24.7837755769557,10.7922330265442));
#86925=CARTESIAN_POINT('Ctrl Pts',(-9.13194198885277,20.2233815417423,9.19360256427126));
#86926=CARTESIAN_POINT('Ctrl Pts',(-8.68314303833994,16.8043220411772,5.77829021316709));
#86927=CARTESIAN_POINT('Ctrl Pts',(-8.23434408782711,15.2105385150611,1.21574430151608));
#86928=CARTESIAN_POINT('Ctrl Pts',(-7.78554513731429,15.7495241089229,-3.58626610828099));
#86929=CARTESIAN_POINT('Ctrl Pts',(-7.4863458369724,17.4646580630017,-6.31390046791915));
#86930=CARTESIAN_POINT('Ctrl Pts',(-7.33674618680146,18.5753787975412,-7.42462120245874));
#86931=CARTESIAN_POINT('Ctrl Pts',(-13.4908740109291,30.2439369421926,4.24050648359456));
#86932=CARTESIAN_POINT('Ctrl Pts',(-13.3411395863725,29.608990997377,4.87597487355288));
#86933=CARTESIAN_POINT('Ctrl Pts',(-13.041805511645,28.0500549640659,5.8557535852361));
#86934=CARTESIAN_POINT('Ctrl Pts',(-12.5928717867465,25.3050835881141,6.16638591073518));
#86935=CARTESIAN_POINT('Ctrl Pts',(-12.1440728362336,22.6994045647989,5.25296892729081));
#86936=CARTESIAN_POINT('Ctrl Pts',(-11.6952738857208,20.7458476630348,3.30155975703115));
#86937=CARTESIAN_POINT('Ctrl Pts',(-11.246474935208,19.8352103074259,0.694647717400992));
#86938=CARTESIAN_POINT('Ctrl Pts',(-10.7975412103096,20.1432585780077,-2.04991105844832));
#86939=CARTESIAN_POINT('Ctrl Pts',(-10.498207135582,21.1240260162405,-3.60899112699502));
#86940=CARTESIAN_POINT('Ctrl Pts',(-10.3484727110254,21.7594935152029,-4.24393694201739));
#86941=CARTESIAN_POINT('Ctrl Pts',(-13.8788514230801,31.305165472356,5.30087720164032));
#86942=CARTESIAN_POINT('Ctrl Pts',(-13.7291169985234,30.5114464918125,6.09524926868588));
#86943=CARTESIAN_POINT('Ctrl Pts',(-13.4297829237959,28.5626867128182,7.32002905749346));
#86944=CARTESIAN_POINT('Ctrl Pts',(-12.9808491988975,25.1313144835263,7.70833734535978));
#86945=CARTESIAN_POINT('Ctrl Pts',(-12.5320502483847,21.8740657131446,6.56651353684457));
#86946=CARTESIAN_POINT('Ctrl Pts',(-12.0832512978718,19.4320071329416,4.12713974465246));
#86947=CARTESIAN_POINT('Ctrl Pts',(-11.634452347359,18.2936580192251,0.868349632900707));
#86948=CARTESIAN_POINT('Ctrl Pts',(-11.1855186224605,18.6787360896981,-2.56250682251239));
#86949=CARTESIAN_POINT('Ctrl Pts',(-10.886184547733,19.904751843607,-4.5114466538425));
#86950=CARTESIAN_POINT('Ctrl Pts',(-10.7364501231764,20.6991227968565,-5.30516547213704));
#86951=CARTESIAN_POINT('Ctrl Pts',(-14.266828835231,32.3663940025195,6.36124791968608));
#86952=CARTESIAN_POINT('Ctrl Pts',(-14.1170944106744,31.413901986248,7.3145236638189));
#86953=CARTESIAN_POINT('Ctrl Pts',(-13.8177603359469,29.0753184615703,8.78430452975083));
#86954=CARTESIAN_POINT('Ctrl Pts',(-13.3688266110484,24.9575453789385,9.25028877998437));
#86955=CARTESIAN_POINT('Ctrl Pts',(-12.9200276605356,21.0487268614902,7.88005814639835));
#86956=CARTESIAN_POINT('Ctrl Pts',(-12.4712287100228,18.1181666028484,4.95271973227379));
#86957=CARTESIAN_POINT('Ctrl Pts',(-12.0224297595099,16.7521057310242,1.04205154840042));
#86958=CARTESIAN_POINT('Ctrl Pts',(-11.5734960346114,17.2142136013887,-3.07510258657646));
#86959=CARTESIAN_POINT('Ctrl Pts',(-11.2741619598839,18.6854776709736,-5.41390218068998));
#86960=CARTESIAN_POINT('Ctrl Pts',(-11.1244275353273,19.63875207851,-6.36639400225669));
#86961=CARTESIAN_POINT('Ctrl Pts',(-14.6548062473819,33.4276225326829,7.42161863773185));
#86962=CARTESIAN_POINT('Ctrl Pts',(-14.5050718228254,32.3163574806835,8.5337980589519));
#86963=CARTESIAN_POINT('Ctrl Pts',(-14.2057377480978,29.5879502103225,10.2485800020082));
#86964=CARTESIAN_POINT('Ctrl Pts',(-13.7568040231994,24.7837762743506,10.792240214609));
#86965=CARTESIAN_POINT('Ctrl Pts',(-13.3080050726865,20.2233880098358,9.19360275595211));
#86966=CARTESIAN_POINT('Ctrl Pts',(-12.8592061221737,16.8043260727552,5.7782997198951));
#86967=CARTESIAN_POINT('Ctrl Pts',(-12.4104071716609,15.2105534428233,1.21575346390014));
#86968=CARTESIAN_POINT('Ctrl Pts',(-11.9614734467625,15.7496911130792,-3.58769835064053));
#86969=CARTESIAN_POINT('Ctrl Pts',(-11.6621393720349,17.4662034983402,-6.31635770753746));
#86970=CARTESIAN_POINT('Ctrl Pts',(-11.5124049474783,18.5783813601636,-7.42762253237636));
#86971=CARTESIAN_POINT('Ctrl Pts',(-14.654401924225,33.4246212024587,7.42462120245875));
#86972=CARTESIAN_POINT('Ctrl Pts',(-14.5048022740541,32.3139004679191,8.53534193699834));
#86973=CARTESIAN_POINT('Ctrl Pts',(-14.3552022737683,30.950203150656,9.39204196234938));
#86974=CARTESIAN_POINT('Ctrl Pts',(-14.2056027244668,29.467899597397,9.91097554778974));
#86975=CARTESIAN_POINT('Ctrl Pts',(-14.0560031751652,27.9855960441379,10.4299091332301));
#86976=CARTESIAN_POINT('Ctrl Pts',(-13.9064036151766,26.3846862358993,10.6110743887871));
#86977=CARTESIAN_POINT('Ctrl Pts',(-13.7568040801578,24.8241674369159,10.4352178717254));
#86978=CARTESIAN_POINT('Ctrl Pts',(-13.6072045451391,23.2636486379325,10.2593613546637));
#86979=CARTESIAN_POINT('Ctrl Pts',(-13.4576049659318,21.7435197923166,9.72648287486196));
#86980=CARTESIAN_POINT('Ctrl Pts',(-13.308005280278,20.4136116476536,8.89082647512689));
#86981=CARTESIAN_POINT('Ctrl Pts',(-13.1584055946242,19.0837035029906,8.05517007539182));
#86982=CARTESIAN_POINT('Ctrl Pts',(-13.0088061501224,17.944016056696,6.91673693379781));
#86983=CARTESIAN_POINT('Ctrl Pts',(-12.8592063826122,17.1085441761431,5.58709619172128));
#86984=CARTESIAN_POINT('Ctrl Pts',(-12.7096066151021,16.2730722955903,4.25745544964474));
#86985=CARTESIAN_POINT('Ctrl Pts',(-12.5600063513476,15.7418162640707,2.73660675503515));
#86986=CARTESIAN_POINT('Ctrl Pts',(-12.4104064355152,15.5660167942965,1.17584743948898));
#86987=CARTESIAN_POINT('Ctrl Pts',(-12.2608065196829,15.3902173245223,-0.384911876057196));
#86988=CARTESIAN_POINT('Ctrl Pts',(-12.1112069917185,15.5698744476954,-1.98558179310599));
#86989=CARTESIAN_POINT('Ctrl Pts',(-11.961607556327,16.0884846261068,-3.46782894584021));
#86990=CARTESIAN_POINT('Ctrl Pts',(-11.8120081209356,16.6070948045182,-4.95007609857443));
#86991=CARTESIAN_POINT('Ctrl Pts',(-11.6624089208062,17.4646580630017,-6.31390046791915));
#86992=CARTESIAN_POINT('Ctrl Pts',(-11.5128092706352,18.5753787975412,-7.4246212024587));
#86993=CARTESIAN_POINT('Ctrl Pts',(-16.7615242403913,33.4246212024587,7.42462120245875));
#86994=CARTESIAN_POINT('Ctrl Pts',(-16.6119245902203,32.3139004679191,8.53534193699834));
#86995=CARTESIAN_POINT('Ctrl Pts',(-16.3127252898784,29.5865056944476,10.2487418519882));
#86996=CARTESIAN_POINT('Ctrl Pts',(-15.8639263393656,24.7837766896879,10.7922435813033));
#86997=CARTESIAN_POINT('Ctrl Pts',(-15.4151273888528,20.2233911279431,9.19360303844964));
#86998=CARTESIAN_POINT('Ctrl Pts',(-14.9663284383399,16.8043281386818,5.77830424745898));
#86999=CARTESIAN_POINT('Ctrl Pts',(-14.5175294878271,15.2105604801153,1.2157578802817));
#87000=CARTESIAN_POINT('Ctrl Pts',(-14.0686160154007,15.7496693261982,-3.58747702651184));
#87001=CARTESIAN_POINT('Ctrl Pts',(-13.7693021931453,17.4659712295614,-6.31598847532156));
#87002=CARTESIAN_POINT('Ctrl Pts',(-13.6195880210608,18.5779300880552,-7.42717160290573));
#87003=CARTESIAN_POINT('Ctrl Pts',(-17.1494939834484,32.3638424588395,6.3638424588395));
#87004=CARTESIAN_POINT('Ctrl Pts',(-16.9998943332774,31.4118138532541,7.31587106442488));
#87005=CARTESIAN_POINT('Ctrl Pts',(-16.7006950329356,29.0740904612934,8.78447219984358));
#87006=CARTESIAN_POINT('Ctrl Pts',(-16.2518960824227,24.9575423000662,9.25032214520139));
#87007=CARTESIAN_POINT('Ctrl Pts',(-15.8030971319099,21.0487132197491,7.88008435318242));
#87008=CARTESIAN_POINT('Ctrl Pts',(-15.3542981813971,18.1181424031123,4.9527399320917));
#87009=CARTESIAN_POINT('Ctrl Pts',(-14.9054992308842,16.7520812912335,1.04205876734065));
#87010=CARTESIAN_POINT('Ctrl Pts',(-14.4565857584578,17.2141659782612,-3.07492301612194));
#87011=CARTESIAN_POINT('Ctrl Pts',(-14.1572719362024,18.6852544859406,-5.41360354053909));
#87012=CARTESIAN_POINT('Ctrl Pts',(-14.0075577641179,19.6383443208567,-6.36602847563537));
#87013=CARTESIAN_POINT('Ctrl Pts',(-17.5374637265055,31.3030637152202,5.30306371522026));
#87014=CARTESIAN_POINT('Ctrl Pts',(-17.3878640763346,30.5097272385891,6.09640019185142));
#87015=CARTESIAN_POINT('Ctrl Pts',(-17.0886647759927,28.5616752281392,7.32020254769893));
#87016=CARTESIAN_POINT('Ctrl Pts',(-16.6398658254799,25.1313079104446,7.70840070909949));
#87017=CARTESIAN_POINT('Ctrl Pts',(-16.191066874967,21.8740353115551,6.5665656679152));
#87018=CARTESIAN_POINT('Ctrl Pts',(-15.7422679244542,19.431956667543,4.1271756167244));
#87019=CARTESIAN_POINT('Ctrl Pts',(-15.2934689739414,18.2936021023516,0.868359654399596));
#87020=CARTESIAN_POINT('Ctrl Pts',(-14.844555501515,18.6786626303243,-2.56236900573204));
#87021=CARTESIAN_POINT('Ctrl Pts',(-14.5452416792596,19.9045377423199,-4.51121860575662));
#87022=CARTESIAN_POINT('Ctrl Pts',(-14.395527507175,20.6987585536582,-5.30488534836501));
#87023=CARTESIAN_POINT('Ctrl Pts',(-17.9254334695626,30.242284971601,4.242284971601));
#87024=CARTESIAN_POINT('Ctrl Pts',(-17.7758338193916,29.607640623924,4.87692931927796));
#87025=CARTESIAN_POINT('Ctrl Pts',(-17.4766345190497,28.049259994985,5.85593289555428));
#87026=CARTESIAN_POINT('Ctrl Pts',(-17.0278355685369,25.3050735208229,6.1664792729976));
#87027=CARTESIAN_POINT('Ctrl Pts',(-16.5790366180241,22.699357403361,5.25304698264799));
#87028=CARTESIAN_POINT('Ctrl Pts',(-16.1302376675113,20.7457709319735,3.30161130135711));
#87029=CARTESIAN_POINT('Ctrl Pts',(-15.6814387169984,19.8351229134697,0.694660541458542));
#87030=CARTESIAN_POINT('Ctrl Pts',(-15.2325252445721,20.1431592823874,-2.04981499534212));
#87031=CARTESIAN_POINT('Ctrl Pts',(-14.9332114223166,21.1238209986992,-3.60883367097415));
#87032=CARTESIAN_POINT('Ctrl Pts',(-14.7834972502322,21.7591727864597,-4.24374222109464));
#87033=CARTESIAN_POINT('Ctrl Pts',(-16.7615242403913,33.4246212024587,7.42462120245875));
#87034=CARTESIAN_POINT('Ctrl Pts',(-16.6119245902203,32.3139004679191,8.53534193699834));
#87035=CARTESIAN_POINT('Ctrl Pts',(-16.3127252898784,29.5865056944476,10.2487418519882));
#87036=CARTESIAN_POINT('Ctrl Pts',(-15.8639263393656,24.7837766896879,10.7922435813033));
#87037=CARTESIAN_POINT('Ctrl Pts',(-15.4151273888528,20.2233911279431,9.19360303844964));
#87038=CARTESIAN_POINT('Ctrl Pts',(-14.9663284383399,16.8043281386818,5.77830424745898));
#87039=CARTESIAN_POINT('Ctrl Pts',(-14.5175294878271,15.2105604801153,1.2157578802817));
#87040=CARTESIAN_POINT('Ctrl Pts',(-14.0687305373143,15.7495317946237,-3.58625167756031));
#87041=CARTESIAN_POINT('Ctrl Pts',(-13.7695312369724,17.4646580630017,-6.31390046791915));
#87042=CARTESIAN_POINT('Ctrl Pts',(-13.6199315868015,18.5753787975412,-7.42462120245874));
#87043=CARTESIAN_POINT('Ctrl Pts',(-14.654401924225,33.4246212024587,7.42462120245875));
#87044=CARTESIAN_POINT('Ctrl Pts',(-14.5048022740541,32.3139004679191,8.53534193699834));
#87045=CARTESIAN_POINT('Ctrl Pts',(-14.2056029737122,29.5865056944476,10.2487418519882));
#87046=CARTESIAN_POINT('Ctrl Pts',(-13.7568040231994,24.7837766896879,10.7922435813033));
#87047=CARTESIAN_POINT('Ctrl Pts',(-13.3080050726865,20.2233911279431,9.19360303844964));
#87048=CARTESIAN_POINT('Ctrl Pts',(-12.8592061221737,16.8043281386818,5.77830424745898));
#87049=CARTESIAN_POINT('Ctrl Pts',(-12.4104071716609,15.2105604801153,1.2157578802817));
#87050=CARTESIAN_POINT('Ctrl Pts',(-11.9616082211481,15.7495317946237,-3.58625167756031));
#87051=CARTESIAN_POINT('Ctrl Pts',(-11.6624089208062,17.4646580630017,-6.31390046791915));
#87052=CARTESIAN_POINT('Ctrl Pts',(-11.5128092706352,18.5753787975412,-7.42462120245874));
#87053=CARTESIAN_POINT('Ctrl Pts',(-15.3567760296138,33.4246212024587,7.42462120245875));
#87054=CARTESIAN_POINT('Ctrl Pts',(-15.2071763794428,32.3139004679191,8.53534193699834));
#87055=CARTESIAN_POINT('Ctrl Pts',(-14.9079770791009,29.5865056944476,10.2487418519882));
#87056=CARTESIAN_POINT('Ctrl Pts',(-14.4591781285881,24.7837766896879,10.7922435813033));
#87057=CARTESIAN_POINT('Ctrl Pts',(-14.0103791780753,20.2233911279431,9.19360303844963));
#87058=CARTESIAN_POINT('Ctrl Pts',(-13.5615802275625,16.8043281386818,5.77830424745898));
#87059=CARTESIAN_POINT('Ctrl Pts',(-13.1127812770496,15.2105604801153,1.2157578802817));
#87060=CARTESIAN_POINT('Ctrl Pts',(-12.6639823265368,15.7495317946237,-3.58625167756031));
#87061=CARTESIAN_POINT('Ctrl Pts',(-12.3647830261949,17.4646580630017,-6.31390046791915));
#87062=CARTESIAN_POINT('Ctrl Pts',(-12.215183376024,18.5753787975412,-7.42462120245874));
#87063=CARTESIAN_POINT('Ctrl Pts',(-16.0591501350025,33.4246212024587,7.42462120245875));
#87064=CARTESIAN_POINT('Ctrl Pts',(-15.9095504848316,32.3139004679191,8.53534193699834));
#87065=CARTESIAN_POINT('Ctrl Pts',(-15.6103511844897,29.5865056944476,10.2487418519882));
#87066=CARTESIAN_POINT('Ctrl Pts',(-15.1615522339768,24.7837766896879,10.7922435813033));
#87067=CARTESIAN_POINT('Ctrl Pts',(-14.712753283464,20.2233911279431,9.19360303844964));
#87068=CARTESIAN_POINT('Ctrl Pts',(-14.2639543329512,16.8043281386818,5.77830424745898));
#87069=CARTESIAN_POINT('Ctrl Pts',(-13.8151553824384,15.2105604801153,1.2157578802817));
#87070=CARTESIAN_POINT('Ctrl Pts',(-13.3663564319255,15.7495317946237,-3.58625167756031));
#87071=CARTESIAN_POINT('Ctrl Pts',(-13.0671571315837,17.4646580630017,-6.31390046791915));
#87072=CARTESIAN_POINT('Ctrl Pts',(-12.9175574814127,18.5753787975412,-7.42462120245874));
#87073=CARTESIAN_POINT('Ctrl Pts',(-16.7615242403913,33.4246212024587,7.42462120245875));
#87074=CARTESIAN_POINT('Ctrl Pts',(-16.6119245902203,32.3139004679191,8.53534193699834));
#87075=CARTESIAN_POINT('Ctrl Pts',(-16.3127252898784,29.5865056944476,10.2487418519882));
#87076=CARTESIAN_POINT('Ctrl Pts',(-15.8639263393656,24.7837766896879,10.7922435813033));
#87077=CARTESIAN_POINT('Ctrl Pts',(-15.4151273888528,20.2233911279431,9.19360303844964));
#87078=CARTESIAN_POINT('Ctrl Pts',(-14.9663284383399,16.8043281386818,5.77830424745898));
#87079=CARTESIAN_POINT('Ctrl Pts',(-14.5175294878271,15.2105604801153,1.2157578802817));
#87080=CARTESIAN_POINT('Ctrl Pts',(-14.0687305373143,15.7495317946237,-3.58625167756031));
#87081=CARTESIAN_POINT('Ctrl Pts',(-13.7695312369724,17.4646580630017,-6.31390046791915));
#87082=CARTESIAN_POINT('Ctrl Pts',(-13.6199315868015,18.5753787975412,-7.42462120245874));
#87083=CARTESIAN_POINT('Origin',(-36.6591285358979,26.,7.7715611723761E-15));
#88466=UNCERTAINTY_MEASURE_WITH_UNIT(LENGTH_MEASURE(0.01),#88484,
'DISTANCE_ACCURACY_VALUE',
'Maximum model space distance between geometric entities at asserted c
onnectivities');
#88472=UNCERTAINTY_MEASURE_WITH_UNIT(LENGTH_MEASURE(0.01),#88484,
'DISTANCE_ACCURACY_VALUE',
'Maximum model space distance between geometric entities at asserted c
onnectivities');
#88477=(
GEOMETRIC_REPRESENTATION_CONTEXT(3)
GLOBAL_UNCERTAINTY_ASSIGNED_CONTEXT((#88466))
GLOBAL_UNIT_ASSIGNED_CONTEXT((#88484,#88486,#88487))
REPRESENTATION_CONTEXT('','3D')
);
#88483=(
GEOMETRIC_REPRESENTATION_CONTEXT(3)
GLOBAL_UNCERTAINTY_ASSIGNED_CONTEXT((#88472))
GLOBAL_UNIT_ASSIGNED_CONTEXT((#88484,#88486,#88487))
REPRESENTATION_CONTEXT('','3D')
);
#88484=(
LENGTH_UNIT()
NAMED_UNIT(*)
SI_UNIT(.MILLI.,.METRE.)
);
#88486=(
NAMED_UNIT(*)
PLANE_ANGLE_UNIT()
SI_UNIT($,.RADIAN.)
);
#88487=(
NAMED_UNIT(*)
SI_UNIT($,.STERADIAN.)
SOLID_ANGLE_UNIT()
);
#88492=SHAPE_DEFINITION_REPRESENTATION(#88502,#88523);
#88502=PRODUCT_DEFINITION_SHAPE('',$,#88534);
#88523=SHAPE_REPRESENTATION('',(#13828),#88477);
#88529=PRODUCT_DEFINITION_CONTEXT('part definition',#88561,'design');
#88534=PRODUCT_DEFINITION('Wormgear_Shaft','Wormgear_Shaft',#88544,#88529);
#88544=PRODUCT_DEFINITION_FORMATION('',$,#88567);
#88561=APPLICATION_CONTEXT(
'Core Data for Automotive Mechanical Design Process');
#88562=PRODUCT_CONTEXT('part definition',#88561,'mechanical');
#88567=PRODUCT('Wormgear_Shaft','Wormgear_Shaft',$,(#88562));
#88574=PRESENTATION_STYLE_ASSIGNMENT((#88576));
#88576=SURFACE_STYLE_USAGE(.BOTH.,#88578);
#88578=SURFACE_SIDE_STYLE('',(#88580));
#88580=SURFACE_STYLE_FILL_AREA(#88582);
#88582=FILL_AREA_STYLE('Opaque(160,160,160)',(#88584));
#88584=FILL_AREA_STYLE_COLOUR('Opaque(160,160,160)',#88586);
#88586=COLOUR_RGB('Opaque(160,160,160)', 0.66274510, 0.83137255, 0.94901961);
ENDSEC;
END-ISO-10303-21;
